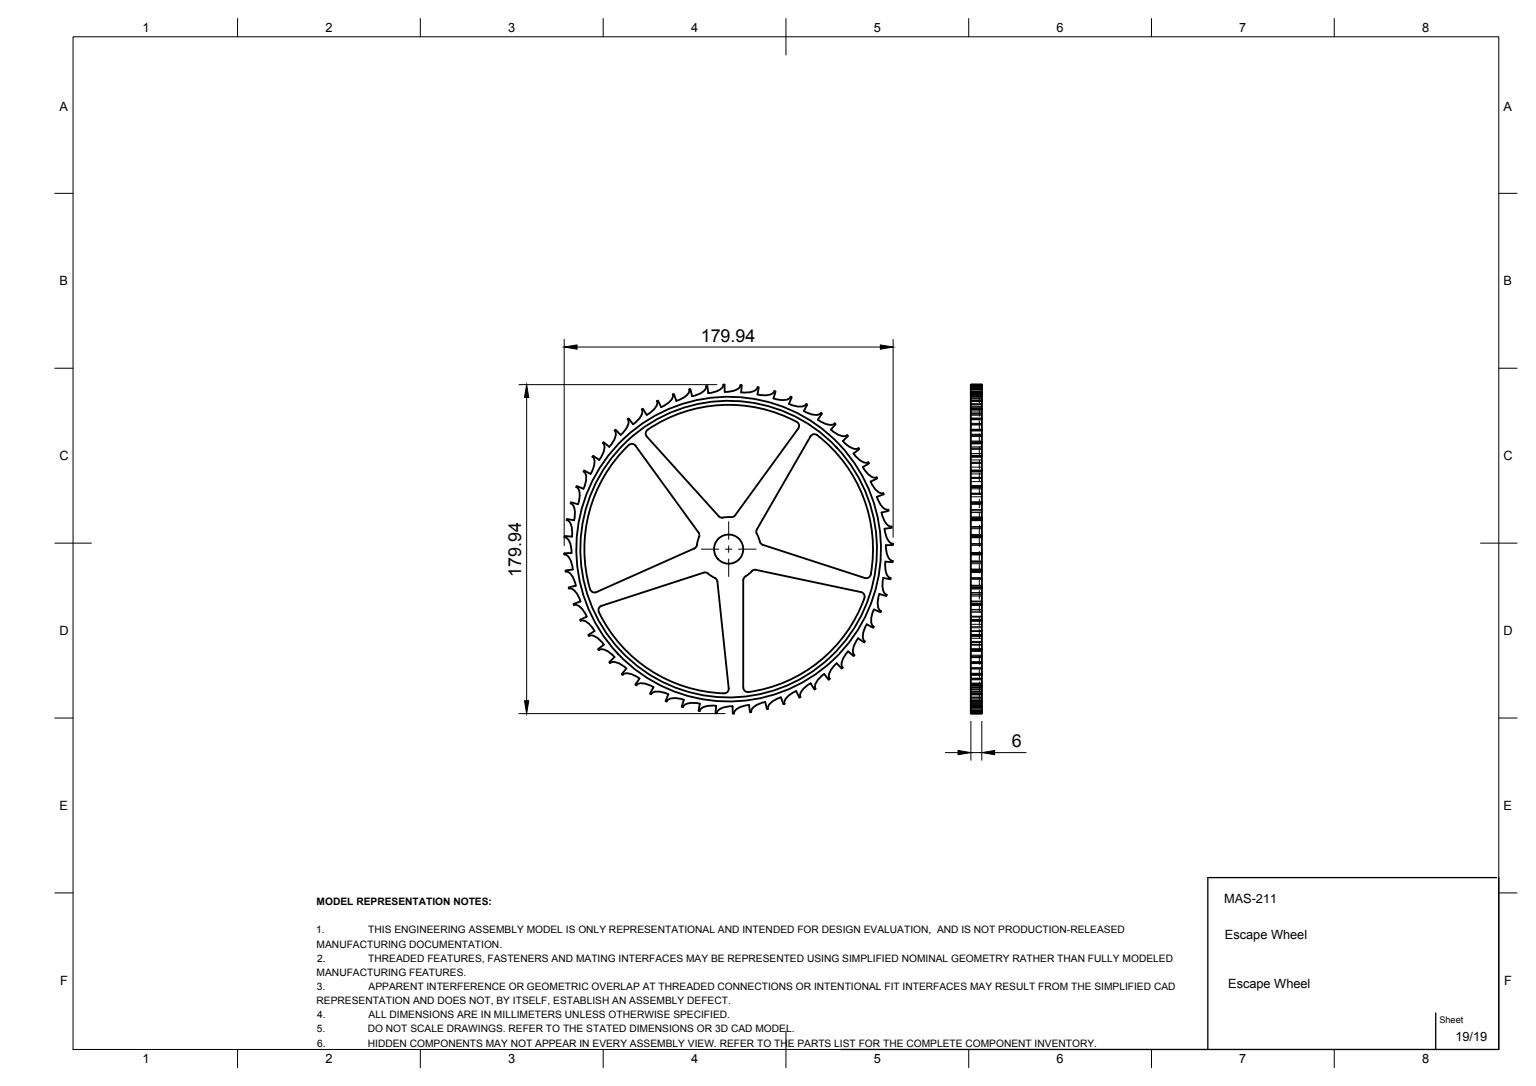
ISO-10303-21;
HEADER;
FILE_DESCRIPTION(
 (''),
 '2;1');
FILE_NAME ( 'Escape Wheel.step', '2026-10-05T20:07:59+06:00', ( '' ), ( '' ), 'STEP AP214', 'Unspecified', '' );
FILE_SCHEMA (('AUTOMOTIVE_DESIGN { 1 0 10303 214 3 1 1 }'));
ENDSEC;
DATA;
#10=MECHANICAL_DESIGN_GEOMETRIC_PRESENTATION_REPRESENTATION('',(#337),#196741);
#71=(
BOUNDED_SURFACE()
B_SPLINE_SURFACE(2,1,((#194862,#194863),(#194864,#194865),(#194866,#194867),
(#194868,#194869),(#194870,#194871)),.UNSPECIFIED.,.F.,.F.,.F.)
B_SPLINE_SURFACE_WITH_KNOTS((3,2,3),(2,2),(-88.8644935634662,-88.8637621488937,
-87.3177026764144),(0.,0.72),.UNSPECIFIED.)
GEOMETRIC_REPRESENTATION_ITEM()
RATIONAL_B_SPLINE_SURFACE(((1.,1.),(1.00013629089276,1.00013629089276),
(1.0002727088269,1.0002727088269),(0.711913347097769,0.711913347097769),
(0.991190559346467,0.991190559346467)))
REPRESENTATION_ITEM('')
SURFACE()
) ;
#72=(
BOUNDED_SURFACE()
B_SPLINE_SURFACE(2,1,((#194889,#194890),(#194891,#194892),(#194893,#194894),
(#194895,#194896),(#194897,#194898)),.UNSPECIFIED.,.F.,.F.,.F.)
B_SPLINE_SURFACE_WITH_KNOTS((3,2,3),(2,2),(-82.6275148008652,-82.6267833862927,
-81.0807239138134),(0.,0.720000000000001),.UNSPECIFIED.)
GEOMETRIC_REPRESENTATION_ITEM()
RATIONAL_B_SPLINE_SURFACE(((0.991190559346467,0.991190559346467),(0.991325649592695,
0.991325649592695),(0.991460865761138,0.991460865761138),(0.705641788716053,
0.705641788716053),(0.982458724937563,0.982458724937563)))
REPRESENTATION_ITEM('')
SURFACE()
) ;
#73=(
BOUNDED_SURFACE()
B_SPLINE_SURFACE(2,1,((#194916,#194917),(#194918,#194919),(#194920,#194921),
(#194922,#194923),(#194924,#194925)),.UNSPECIFIED.,.F.,.F.,.F.)
B_SPLINE_SURFACE_WITH_KNOTS((3,2,3),(2,2),(-76.3905360382642,-76.3898046236916,
-74.8437451512123),(0.,0.720000000000001),.UNSPECIFIED.)
GEOMETRIC_REPRESENTATION_ITEM()
RATIONAL_B_SPLINE_SURFACE(((0.982458724937563,0.982458724937563),(0.982592625114284,
0.982592625114284),(0.982726650103915,0.982726650103915),(0.699425479255707,
0.699425479255707),(0.97380381310568,0.97380381310568)))
REPRESENTATION_ITEM('')
SURFACE()
) ;
#74=(
BOUNDED_SURFACE()
B_SPLINE_SURFACE(2,1,((#194943,#194944),(#194945,#194946),(#194947,#194948),
(#194949,#194950),(#194951,#194952)),.UNSPECIFIED.,.F.,.F.,.F.)
B_SPLINE_SURFACE_WITH_KNOTS((3,2,3),(2,2),(-70.1535572756631,-70.1528258610906,
-68.6067663886113),(0.,0.720000000000001),.UNSPECIFIED.)
GEOMETRIC_REPRESENTATION_ITEM()
RATIONAL_B_SPLINE_SURFACE(((0.97380381310568,0.97380381310568),(0.97393653369674,
0.97393653369674),(0.974069378001179,0.974069378001179),(0.693263932004635,
0.693263932004635),(0.965225146205942,0.965225146205942)))
REPRESENTATION_ITEM('')
SURFACE()
) ;
#75=(
BOUNDED_SURFACE()
B_SPLINE_SURFACE(2,1,((#194970,#194971),(#194972,#194973),(#194974,#194975),
(#194976,#194977),(#194978,#194979)),.UNSPECIFIED.,.F.,.F.,.F.)
B_SPLINE_SURFACE_WITH_KNOTS((3,2,3),(2,2),(-63.9165785130621,-63.9158470984896,
-62.3697876260103),(0.,0.72),.UNSPECIFIED.)
GEOMETRIC_REPRESENTATION_ITEM()
RATIONAL_B_SPLINE_SURFACE(((0.965225146205942,0.965225146205942),(0.965356697602832,
0.965356697602832),(0.965488371623255,0.965488371623255),(0.687156664538405,
0.687156664538405),(0.956722052563143,0.956722052563143)))
REPRESENTATION_ITEM('')
SURFACE()
) ;
#76=(
BOUNDED_SURFACE()
B_SPLINE_SURFACE(2,1,((#194997,#194998),(#194999,#195000),(#195001,#195002),
(#195003,#195004),(#195005,#195006)),.UNSPECIFIED.,.F.,.F.,.F.)
B_SPLINE_SURFACE_WITH_KNOTS((3,2,3),(2,2),(-57.6795997504611,-57.6788683358886,
-56.1328088634093),(0.,0.720000000000001),.UNSPECIFIED.)
GEOMETRIC_REPRESENTATION_ITEM()
RATIONAL_B_SPLINE_SURFACE(((0.956722052563143,0.956722052563143),(0.956852445065809,
0.956852445065809),(0.956982959111764,0.956982959111764),(0.681103198682475,
0.681103198682475),(0.948293866419162,0.948293866419162)))
REPRESENTATION_ITEM('')
SURFACE()
) ;
#77=(
BOUNDED_SURFACE()
B_SPLINE_SURFACE(2,1,((#195024,#195025),(#195026,#195027),(#195028,#195029),
(#195030,#195031),(#195032,#195033)),.UNSPECIFIED.,.F.,.F.,.F.)
B_SPLINE_SURFACE_WITH_KNOTS((3,2,3),(2,2),(-51.4426209878601,-51.4418895732875,
-49.8958301008082),(0.,0.720000000000001),.UNSPECIFIED.)
GEOMETRIC_REPRESENTATION_ITEM()
RATIONAL_B_SPLINE_SURFACE(((0.948293866419162,0.948293866419162),(0.948423110236814,
0.948423110236814),(0.948552474527026,0.948552474527026),(0.67510306047475,
0.67510306047475),(0.939939927880833,0.939939927880833)))
REPRESENTATION_ITEM('')
SURFACE()
) ;
#78=(
BOUNDED_SURFACE()
B_SPLINE_SURFACE(2,1,((#195051,#195052),(#195053,#195054),(#195055,#195056),
(#195057,#195058),(#195059,#195060)),.UNSPECIFIED.,.F.,.F.,.F.)
B_SPLINE_SURFACE_WITH_KNOTS((3,2,3),(2,2),(-45.205642225259,-45.2049108106865,
-43.6588513382072),(0.,0.72),.UNSPECIFIED.)
GEOMETRIC_REPRESENTATION_ITEM()
RATIONAL_B_SPLINE_SURFACE(((0.939939927880833,0.939939927880833),(0.940068033132744,
0.940068033132744),(0.940196257795919,0.940196257795919),(0.66915578012848,
0.66915578012848),(0.931659582868281,0.931659582868281)))
REPRESENTATION_ITEM('')
SURFACE()
) ;
#79=(
BOUNDED_SURFACE()
B_SPLINE_SURFACE(2,1,((#195078,#195079),(#195080,#195081),(#195082,#195083),
(#195084,#195085),(#195086,#195087)),.UNSPECIFIED.,.F.,.F.,.F.)
B_SPLINE_SURFACE_WITH_KNOTS((3,2,3),(2,2),(-38.968663462658,-38.9679320480855,
-37.4218725756062),(0.,0.720000000000001),.UNSPECIFIED.)
GEOMETRIC_REPRESENTATION_ITEM()
RATIONAL_B_SPLINE_SURFACE(((0.931659582868281,0.931659582868281),(0.931786559584578,
0.931786559584578),(0.931913654660192,0.931913654660192),(0.663260891995469,
0.663260891995469),(0.923452183063708,0.923452183063708)))
REPRESENTATION_ITEM('')
SURFACE()
) ;
#80=(
BOUNDED_SURFACE()
B_SPLINE_SURFACE(2,1,((#195105,#195106),(#195107,#195108),(#195109,#195110),
(#195111,#195112),(#195113,#195114)),.UNSPECIFIED.,.F.,.F.,.F.)
B_SPLINE_SURFACE_WITH_KNOTS((3,2,3),(2,2),(-32.731684700057,-32.7309532854845,
-31.1848938130052),(0.,0.720000000000001),.UNSPECIFIED.)
GEOMETRIC_REPRESENTATION_ITEM()
RATIONAL_B_SPLINE_SURFACE(((0.923452183063708,0.923452183063708),(0.923578041186158,
0.923578041186158),(0.923704016625246,0.923704016625246),(0.657417934529626,
0.657417934529626),(0.915317085860633,0.915317085860633)))
REPRESENTATION_ITEM('')
SURFACE()
) ;
#81=(
BOUNDED_SURFACE()
B_SPLINE_SURFACE(2,1,((#195132,#195133),(#195134,#195135),(#195136,#195137),
(#195138,#195139),(#195140,#195141)),.UNSPECIFIED.,.F.,.F.,.F.)
B_SPLINE_SURFACE_WITH_KNOTS((3,2,3),(2,2),(-26.4947059374559,-26.4939745228834,
-24.9479150504041),(0.,0.720000000000004),.UNSPECIFIED.)
GEOMETRIC_REPRESENTATION_ITEM()
RATIONAL_B_SPLINE_SURFACE(((0.915317085860633,0.915317085860633),(0.915441835243423,
0.915441835243423),(0.915566700909357,0.915566700909357),(0.651626450250819,
0.651626450250819),(0.907253654313579,0.907253654313579)))
REPRESENTATION_ITEM('')
SURFACE()
) ;
#82=(
BOUNDED_SURFACE()
B_SPLINE_SURFACE(2,1,((#195159,#195160),(#195161,#195162),(#195163,#195164),
(#195165,#195166),(#195167,#195168)),.UNSPECIFIED.,.F.,.F.,.F.)
B_SPLINE_SURFACE_WITH_KNOTS((3,2,3),(2,2),(-20.2577271748549,-20.2569957602824,
-18.7109362878031),(0.,0.720000000000001),.UNSPECIFIED.)
GEOMETRIC_REPRESENTATION_ITEM()
RATIONAL_B_SPLINE_SURFACE(((0.907253654313579,0.907253654313579),(0.907377304724085,
0.907377304724085),(0.907501070393345,0.907501070393345),(0.645885985709063,
0.645885985709063),(0.899261257088203,0.899261257088203)))
REPRESENTATION_ITEM('')
SURFACE()
) ;
#83=(
BOUNDED_SURFACE()
B_SPLINE_SURFACE(2,1,((#195186,#195187),(#195188,#195189),(#195190,#195191),
(#195192,#195193),(#195194,#195195)),.UNSPECIFIED.,.F.,.F.,.F.)
B_SPLINE_SURFACE_WITH_KNOTS((3,2,3),(2,2),(-14.0207484122539,-14.0200169976814,
-12.4739575252021),(0.,0.72),.UNSPECIFIED.)
GEOMETRIC_REPRESENTATION_ITEM()
RATIONAL_B_SPLINE_SURFACE(((0.899261257088203,0.899261257088203),(0.899383818207756,
0.899383818207756),(0.899506493570697,0.899506493570697),(0.64019609144901,
0.64019609144901),(0.891339268411863,0.891339268411863)))
REPRESENTATION_ITEM('')
SURFACE()
) ;
#84=(
BOUNDED_SURFACE()
B_SPLINE_SURFACE(2,1,((#195213,#195214),(#195215,#195216),(#195217,#195218),
(#195219,#195220),(#195221,#195222)),.UNSPECIFIED.,.F.,.F.,.F.)
B_SPLINE_SURFACE_WITH_KNOTS((3,2,3),(2,2),(-7.78376964965284,-7.78303823508033,
-6.23697876260103),(0.,0.72),.UNSPECIFIED.)
GEOMETRIC_REPRESENTATION_ITEM()
RATIONAL_B_SPLINE_SURFACE(((0.891339268411863,0.891339268411863),(0.891460749836507,
0.891460749836507),(0.891582344498119,0.891582344498119),(0.634556321974766,
0.634556321974766),(0.883487068024626,0.883487068024626)))
REPRESENTATION_ITEM('')
SURFACE()
) ;
#85=(
BOUNDED_SURFACE()
B_SPLINE_SURFACE(2,1,((#195240,#195241),(#195242,#195243),(#195244,#195245),
(#195246,#195247),(#195248,#195249)),.UNSPECIFIED.,.F.,.F.,.F.)
B_SPLINE_SURFACE_WITH_KNOTS((3,2,3),(2,2),(-1.54679088705182,-1.54605947247931,
0.),(0.,0.72),.UNSPECIFIED.)
GEOMETRIC_REPRESENTATION_ITEM()
RATIONAL_B_SPLINE_SURFACE(((0.883487068024626,0.883487068024626),(0.883607479265868,
0.883607479265868),(0.883728002746525,0.883728002746525),(0.628966235715006,
0.628966235715006),(0.875704041130699,0.875704041130699)))
REPRESENTATION_ITEM('')
SURFACE()
) ;
#86=(
BOUNDED_SURFACE()
B_SPLINE_SURFACE(2,1,((#195267,#195268),(#195269,#195270),(#195271,#195272),
(#195273,#195274),(#195275,#195276)),.UNSPECIFIED.,.F.,.F.,.F.)
B_SPLINE_SURFACE_WITH_KNOTS((3,2,3),(2,2),(4.69018787554921,4.69091929012172,
6.23697876260103),(0.,0.72),.UNSPECIFIED.)
GEOMETRIC_REPRESENTATION_ITEM()
RATIONAL_B_SPLINE_SURFACE(((0.875704041130699,0.875704041130699),(0.875823391616258,
0.875823391616258),(0.875942853352465,0.875942853352465),(0.623425394988399,
0.623425394988399),(0.8679895783503,0.8679895783503)))
REPRESENTATION_ITEM('')
SURFACE()
) ;
#87=(
BOUNDED_SURFACE()
B_SPLINE_SURFACE(2,1,((#195294,#195295),(#195296,#195297),(#195298,#195299),
(#195300,#195301),(#195302,#195303)),.UNSPECIFIED.,.F.,.F.,.F.)
B_SPLINE_SURFACE_WITH_KNOTS((3,2,3),(2,2),(10.9271666381502,10.9278980527228,
12.4739575252021),(0.,0.72),.UNSPECIFIED.)
GEOMETRIC_REPRESENTATION_ITEM()
RATIONAL_B_SPLINE_SURFACE(((0.8679895783503,0.8679895783503),(0.868107877424839,
0.868107877424839),(0.86822628676997,0.86822628676997),(0.617933365969343,
0.617933365969343),(0.860343075671938,0.860343075671938)))
REPRESENTATION_ITEM('')
SURFACE()
) ;
#88=(
BOUNDED_SURFACE()
B_SPLINE_SURFACE(2,1,((#195321,#195322),(#195323,#195324),(#195325,#195326),
(#195327,#195328),(#195329,#195330)),.UNSPECIFIED.,.F.,.F.,.F.)
B_SPLINE_SURFACE_WITH_KNOTS((3,2,3),(2,2),(17.1641454007513,17.1648768153238,
18.7109362878031),(0.,0.72),.UNSPECIFIED.)
GEOMETRIC_REPRESENTATION_ITEM()
RATIONAL_B_SPLINE_SURFACE(((0.860343075671938,0.860343075671938),(0.8604603325978,
0.8604603325978),(0.860577698822833,0.860577698822833),(0.612489718653998,
0.612489718653998),(0.852763934405128,0.852763934405128)))
REPRESENTATION_ITEM('')
SURFACE()
) ;
#89=(
BOUNDED_SURFACE()
B_SPLINE_SURFACE(2,1,((#195348,#195349),(#195350,#195351),(#195352,#195353),
(#195354,#195355),(#195356,#195357)),.UNSPECIFIED.,.F.,.F.,.F.)
B_SPLINE_SURFACE_WITH_KNOTS((3,2,3),(2,2),(23.4011241633523,23.4018555779248,
24.9479150504041),(0.,0.72),.UNSPECIFIED.)
GEOMETRIC_REPRESENTATION_ITEM()
RATIONAL_B_SPLINE_SURFACE(((0.852763934405128,0.852763934405128),(0.852880158363061,
0.852880158363061),(0.8529964906573,0.8529964906573),(0.607094026826617,
0.607094026826617),(0.845251561133513,0.845251561133513)))
REPRESENTATION_ITEM('')
SURFACE()
) ;
#90=(
BOUNDED_SURFACE()
B_SPLINE_SURFACE(2,1,((#195375,#195376),(#195377,#195378),(#195379,#195380),
(#195381,#195382),(#195383,#195384)),.UNSPECIFIED.,.F.,.F.,.F.)
B_SPLINE_SURFACE_WITH_KNOTS((3,2,3),(2,2),(29.6381029259533,29.6388343405258,
31.1848938130052),(0.,0.72),.UNSPECIFIED.)
GEOMETRIC_REPRESENTATION_ITEM()
RATIONAL_B_SPLINE_SURFACE(((0.845251561133513,0.845251561133513),(0.845366761223386,
0.845366761223386),(0.845482068695182,0.845482068695182),(0.601745868026174,
0.601745868026174),(0.837805367668402,0.837805367668402)))
REPRESENTATION_ITEM('')
SURFACE()
) ;
#91=(
BOUNDED_SURFACE()
B_SPLINE_SURFACE(2,1,((#195402,#195403),(#195404,#195405),(#195406,#195407),
(#195408,#195409),(#195410,#195411)),.UNSPECIFIED.,.F.,.F.,.F.)
B_SPLINE_SURFACE_WITH_KNOTS((3,2,3),(2,2),(35.8750816885544,35.8758131031269,
37.4218725756062),(0.,0.72),.UNSPECIFIED.)
GEOMETRIC_REPRESENTATION_ITEM()
RATIONAL_B_SPLINE_SURFACE(((0.837805367668402,0.837805367668402),(0.83791955290992,
0.83791955290992),(0.838033844587386,0.838033844587386),(0.596444823513289,
0.596444823513289),(0.830424771002716,0.830424771002716)))
REPRESENTATION_ITEM('')
SURFACE()
) ;
#92=(
BOUNDED_SURFACE()
B_SPLINE_SURFACE(2,1,((#195429,#195430),(#195431,#195432),(#195433,#195434),
(#195435,#195436),(#195437,#195438)),.UNSPECIFIED.,.F.,.F.,.F.)
B_SPLINE_SURFACE_WITH_KNOTS((3,2,3),(2,2),(42.1120604511554,42.1127918657279,
43.6588513382072),(0.,0.72),.UNSPECIFIED.)
GEOMETRIC_REPRESENTATION_ITEM()
RATIONAL_B_SPLINE_SURFACE(((0.830424771002716,0.830424771002716),(0.830537950336125,
0.830537950336125),(0.830651235167842,0.830651235167842),(0.591190478237442,
0.591190478237442),(0.823109193265344,0.823109193265344)))
REPRESENTATION_ITEM('')
SURFACE()
) ;
#93=(
BOUNDED_SURFACE()
B_SPLINE_SURFACE(2,1,((#195456,#195457),(#195458,#195459),(#195460,#195461),
(#195462,#195463),(#195464,#195465)),.UNSPECIFIED.,.F.,.F.,.F.)
B_SPLINE_SURFACE_WITH_KNOTS((3,2,3),(2,2),(48.3490392137564,48.3497706283289,
49.8958301008082),(0.,0.72),.UNSPECIFIED.)
GEOMETRIC_REPRESENTATION_ITEM()
RATIONAL_B_SPLINE_SURFACE(((0.823109193265344,0.823109193265344),(0.823221375552132,
0.823221375552132),(0.823333662407847,0.823333662407847),(0.585982420804475,
0.585982420804475),(0.815858061675895,0.815858061675895)))
REPRESENTATION_ITEM('')
SURFACE()
) ;
#94=(
BOUNDED_SURFACE()
B_SPLINE_SURFACE(2,1,((#195483,#195484),(#195485,#195486),(#195487,#195488),
(#195489,#195490),(#195491,#195492)),.UNSPECIFIED.,.F.,.F.,.F.)
B_SPLINE_SURFACE_WITH_KNOTS((3,2,3),(2,2),(54.5860179763575,54.58674939093,
56.1328088634093),(0.,0.720000000000001),.UNSPECIFIED.)
GEOMETRIC_REPRESENTATION_ITEM()
RATIONAL_B_SPLINE_SURFACE(((0.815858061675895,0.815858061675895),(0.815969255699486,
0.815969255699486),(0.816080553370809,0.816080553370809),(0.580820243444385,
0.580820243444385),(0.808670808499855,0.808670808499855)))
REPRESENTATION_ITEM('')
SURFACE()
) ;
#95=(
BOUNDED_SURFACE()
B_SPLINE_SURFACE(2,1,((#195510,#195511),(#195512,#195513),(#195514,#195515),
(#195516,#195517),(#195518,#195519)),.UNSPECIFIED.,.F.,.F.,.F.)
B_SPLINE_SURFACE_WITH_KNOTS((3,2,3),(2,2),(60.8229967389585,60.823728153531,
62.3697876260103),(0.,0.720000000000001),.UNSPECIFIED.)
GEOMETRIC_REPRESENTATION_ITEM()
RATIONAL_B_SPLINE_SURFACE(((0.808670808499855,0.808670808499855),(0.808781022966294,
0.808781022966294),(0.808891340167387,0.808891340167387),(0.575703541979391,
0.575703541979391),(0.801546871004132,0.801546871004132)))
REPRESENTATION_ITEM('')
SURFACE()
) ;
#96=(
BOUNDED_SURFACE()
B_SPLINE_SURFACE(2,1,((#195537,#195538),(#195539,#195540),(#195541,#195542),
(#195543,#195544),(#195545,#195546)),.UNSPECIFIED.,.F.,.F.,.F.)
B_SPLINE_SURFACE_WITH_KNOTS((3,2,3),(2,2),(67.0599755015595,67.060706916132,
68.6067663886113),(0.,0.72),.UNSPECIFIED.)
GEOMETRIC_REPRESENTATION_ITEM()
RATIONAL_B_SPLINE_SURFACE(((0.801546871004132,0.801546871004132),(0.801656114542769,
0.801656114542769),(0.801765459911026,0.801765459911026),(0.570631915792295,
0.570631915792295),(0.794485691412996,0.794485691412996)))
REPRESENTATION_ITEM('')
SURFACE()
) ;
#97=(
BOUNDED_SURFACE()
B_SPLINE_SURFACE(2,1,((#195564,#195565),(#195566,#195567),(#195568,#195569),
(#195570,#195571),(#195572,#195573)),.UNSPECIFIED.,.F.,.F.,.F.)
B_SPLINE_SURFACE_WITH_KNOTS((3,2,3),(2,2),(73.2969542641605,73.2976856787331,
74.8437451512124),(0.,0.720000000000001),.UNSPECIFIED.)
GEOMETRIC_REPRESENTATION_ITEM()
RATIONAL_B_SPLINE_SURFACE(((0.794485691412996,0.794485691412996),(0.794593972577163,
0.794593972577163),(0.794702354673887,0.794702354673887),(0.565604967795111,
0.565604967795111),(0.787486716864412,0.787486716864412)))
REPRESENTATION_ITEM('')
SURFACE()
) ;
#98=(
BOUNDED_SURFACE()
B_SPLINE_SURFACE(2,1,((#195591,#195592),(#195593,#195594),(#195595,#195596),
(#195597,#195598),(#195599,#195600)),.UNSPECIFIED.,.F.,.F.,.F.)
B_SPLINE_SURFACE_WITH_KNOTS((3,2,3),(2,2),(79.5339330267616,79.5346644413341,
81.0807239138134),(0.,0.72),.UNSPECIFIED.)
GEOMETRIC_REPRESENTATION_ITEM()
RATIONAL_B_SPLINE_SURFACE(((0.787486716864412,0.787486716864412),(0.78759404413209,
0.78759404413209),(0.787701471443165,0.787701471443165),(0.560622304397977,
0.560622304397977),(0.78054939936675,0.78054939936675)))
REPRESENTATION_ITEM('')
SURFACE()
) ;
#99=(
BOUNDED_SURFACE()
B_SPLINE_SURFACE(2,1,((#195618,#195619),(#195620,#195621),(#195622,#195623),
(#195624,#195625),(#195626,#195627)),.UNSPECIFIED.,.F.,.F.,.F.)
B_SPLINE_SURFACE_WITH_KNOTS((3,2,3),(2,2),(85.7709117893626,85.7716432039351,
87.3177026764144),(0.,0.72),.UNSPECIFIED.)
GEOMETRIC_REPRESENTATION_ITEM()
RATIONAL_B_SPLINE_SURFACE(((0.78054939936675,0.78054939936675),(0.780655781141232,
0.780655781141232),(0.780762262077786,0.780762262077786),(0.555683535478336,
0.555683535478336),(0.773673195755878,0.773673195755878)))
REPRESENTATION_ITEM('')
SURFACE()
) ;
#100=(
BOUNDED_SURFACE()
B_SPLINE_SURFACE(2,1,((#195645,#195646),(#195647,#195648),(#195649,#195650),
(#195651,#195652),(#195653,#195654)),.UNSPECIFIED.,.F.,.F.,.F.)
B_SPLINE_SURFACE_WITH_KNOTS((3,2,3),(2,2),(92.0078905519636,92.0086219665361,
93.5546814390155),(0.,0.720000000000001),.UNSPECIFIED.)
GEOMETRIC_REPRESENTATION_ITEM()
RATIONAL_B_SPLINE_SURFACE(((0.773673195755878,0.773673195755878),(0.773778640366431,
0.773778640366431),(0.773884183265494,0.773884183265494),(0.550788274350394,
0.550788274350394),(0.766857567652637,0.766857567652637)))
REPRESENTATION_ITEM('')
SURFACE()
) ;
#101=(
BOUNDED_SURFACE()
B_SPLINE_SURFACE(2,1,((#195672,#195673),(#195674,#195675),(#195676,#195677),
(#195678,#195679),(#195680,#195681)),.UNSPECIFIED.,.F.,.F.,.F.)
B_SPLINE_SURFACE_WITH_KNOTS((3,2,3),(2,2),(98.2448693145647,98.2456007291372,
99.7916602016165),(0.,0.720000000000001),.UNSPECIFIED.)
GEOMETRIC_REPRESENTATION_ITEM()
RATIONAL_B_SPLINE_SURFACE(((0.766857567652637,0.766857567652637),(0.766962083355152,
0.766962083355152),(0.767066696480309,0.767066696480309),(0.545936137734843,
0.545936137734843),(0.760101981420689,0.760101981420689)))
REPRESENTATION_ITEM('')
SURFACE()
) ;
#102=(
BOUNDED_SURFACE()
B_SPLINE_SURFACE(2,1,((#195699,#195700),(#195701,#195702),(#195703,#195704),
(#195705,#195706),(#195707,#195708)),.UNSPECIFIED.,.F.,.F.,.F.)
B_SPLINE_SURFACE_WITH_KNOTS((3,2,3),(2,2),(104.481848077166,104.482579491738,
106.028638964218),(0.,0.720000000000001),.UNSPECIFIED.)
GEOMETRIC_REPRESENTATION_ITEM()
RATIONAL_B_SPLINE_SURFACE(((0.760101981420689,0.760101981420689),(0.760205576398325,
0.760205576398325),(0.760309267940364,0.760309267940364),(0.541126745728849,
0.541126745728849),(0.753405908124731,0.753405908124731)))
REPRESENTATION_ITEM('')
SURFACE()
) ;
#103=(
BOUNDED_SURFACE()
B_SPLINE_SURFACE(2,1,((#195726,#195727),(#195728,#195729),(#195730,#195731),
(#195732,#195733),(#195734,#195735)),.UNSPECIFIED.,.F.,.F.,.F.)
B_SPLINE_SURFACE_WITH_KNOTS((3,2,3),(2,2),(110.718826839767,110.719558254339,
112.265617726819),(0.,0.720000000000001),.UNSPECIFIED.)
GEOMETRIC_REPRESENTATION_ITEM()
RATIONAL_B_SPLINE_SURFACE(((0.753405908124731,0.753405908124731),(0.753508590488559,
0.753508590488559),(0.753611368566113,0.753611368566113),(0.536359721776312,
0.536359721776312),(0.746768823489085,0.746768823489085)))
REPRESENTATION_ITEM('')
SURFACE()
) ;
#104=(
BOUNDED_SURFACE()
B_SPLINE_SURFACE(2,1,((#195753,#195754),(#195755,#195756),(#195757,#195758),
(#195759,#195760),(#195761,#195762)),.UNSPECIFIED.,.F.,.F.,.F.)
B_SPLINE_SURFACE_WITH_KNOTS((3,2,3),(2,2),(116.955805602368,116.95653701694,
118.50259648942),(0.,0.720000000000001),.UNSPECIFIED.)
GEOMETRIC_REPRESENTATION_ITEM()
RATIONAL_B_SPLINE_SURFACE(((0.746768823489085,0.746768823489085),(0.746870601278723,
0.746870601278723),(0.746972473938902,0.746972473938902),(0.531634692638378,
0.531634692638378),(0.74019020785665,0.74019020785665)))
REPRESENTATION_ITEM('')
SURFACE()
) ;
#105=(
BOUNDED_SURFACE()
B_SPLINE_SURFACE(2,1,((#195780,#195781),(#195782,#195783),(#195784,#195785),
(#195786,#195787),(#195788,#195789)),.UNSPECIFIED.,.F.,.F.,.F.)
B_SPLINE_SURFACE_WITH_KNOTS((3,2,3),(2,2),(123.192784364969,123.193515779541,
124.739575252021),(0.,0.720000000000001),.UNSPECIFIED.)
GEOMETRIC_REPRESENTATION_ITEM()
RATIONAL_B_SPLINE_SURFACE(((0.74019020785665,0.74019020785665),(0.74029108904089,
0.74029108904089),(0.740392064259915,0.740392064259915),(0.526951288364221,
0.526951288364221),(0.73366954614821,0.73366954614821)))
REPRESENTATION_ITEM('')
SURFACE()
) ;
#106=(
BOUNDED_SURFACE()
B_SPLINE_SURFACE(2,1,((#195807,#195808),(#195809,#195810),(#195811,#195812),
(#195813,#195814),(#195815,#195816)),.UNSPECIFIED.,.F.,.F.,.F.)
B_SPLINE_SURFACE_WITH_KNOTS((3,2,3),(2,2),(129.42976312757,129.430494542142,
130.976554014622),(0.,0.720000000000003),.UNSPECIFIED.)
GEOMETRIC_REPRESENTATION_ITEM()
RATIONAL_B_SPLINE_SURFACE(((0.73366954614821,0.73366954614821),(0.733769538625645,
0.733769538625645),(0.73386962430947,0.73386962430947),(0.522309142262074,
0.522309142262074),(0.727206327822113,0.727206327822113)))
REPRESENTATION_ITEM('')
SURFACE()
) ;
#107=(
BOUNDED_SURFACE()
B_SPLINE_SURFACE(2,1,((#195834,#195835),(#195836,#195837),(#195838,#195839),
(#195840,#195841),(#195842,#195843)),.UNSPECIFIED.,.F.,.F.,.F.)
B_SPLINE_SURFACE_WITH_KNOTS((3,2,3),(2,2),(135.666741890171,135.667473304743,
137.213532777223),(0.,0.72),.UNSPECIFIED.)
GEOMETRIC_REPRESENTATION_ITEM()
RATIONAL_B_SPLINE_SURFACE(((0.727206327822113,0.727206327822113),(0.727305439421753,
0.727305439421753),(0.727404643406686,0.727404643406686),(0.517707890870518,
0.517707890870518),(0.720800046834291,0.720800046834291)))
REPRESENTATION_ITEM('')
SURFACE()
) ;
#108=(
BOUNDED_SURFACE()
B_SPLINE_SURFACE(2,1,((#195861,#195862),(#195863,#195864),(#195865,#195866),
(#195867,#195868),(#195869,#195870)),.UNSPECIFIED.,.F.,.F.,.F.)
B_SPLINE_SURFACE_WITH_KNOTS((3,2,3),(2,2),(141.903720652772,141.904452067344,
143.450511539824),(0.,0.72),.UNSPECIFIED.)
GEOMETRIC_REPRESENTATION_ITEM()
RATIONAL_B_SPLINE_SURFACE(((0.720800046834291,0.720800046834291),(0.720898285316175,
0.720898285316175),(0.72099661536949,0.72099661536949),(0.513147173930029,
0.513147173930029),(0.714450201598641,0.714450201598641)))
REPRESENTATION_ITEM('')
SURFACE()
) ;
#109=(
BOUNDED_SURFACE()
B_SPLINE_SURFACE(2,1,((#195888,#195889),(#195890,#195891),(#195892,#195893),
(#195894,#195895),(#195896,#195897)),.UNSPECIFIED.,.F.,.F.,.F.)
B_SPLINE_SURFACE_WITH_KNOTS((3,2,3),(2,2),(148.140699415373,148.141430829945,
149.687490302425),(0.,0.72),.UNSPECIFIED.)
GEOMETRIC_REPRESENTATION_ITEM()
RATIONAL_B_SPLINE_SURFACE(((0.714450201598641,0.714450201598641),(0.714547574654449,
0.714547574654449),(0.714645038474995,0.714645038474995),(0.508626634354764,
0.508626634354764),(0.708156294947753,0.708156294947753)))
REPRESENTATION_ITEM('')
SURFACE()
) ;
#110=(
BOUNDED_SURFACE()
B_SPLINE_SURFACE(2,1,((#195915,#195916),(#195917,#195918),(#195919,#195920),
(#195921,#195922),(#195923,#195924)),.UNSPECIFIED.,.F.,.F.,.F.)
B_SPLINE_SURFACE_WITH_KNOTS((3,2,3),(2,2),(154.377678177974,154.378409592546,
155.924469065026),(0.,0.72),.UNSPECIFIED.)
GEOMETRIC_REPRESENTATION_ITEM()
RATIONAL_B_SPLINE_SURFACE(((0.708156294947753,0.708156294947753),(0.708252810201405,
0.708252810201405),(0.708349415420208,0.708349415420208),(0.50414591820461,
0.50414591820461),(0.701917834093985,0.701917834093985)))
REPRESENTATION_ITEM('')
SURFACE()
) ;
#111=(
BOUNDED_SURFACE()
B_SPLINE_SURFACE(2,1,((#195942,#195943),(#195944,#195945),(#195946,#195947),
(#195948,#195949),(#195950,#195951)),.UNSPECIFIED.,.F.,.F.,.F.)
B_SPLINE_SURFACE_WITH_KNOTS((3,2,3),(2,2),(160.614656940575,160.615388355147,
162.161447827627),(0.,0.72),.UNSPECIFIED.)
GEOMETRIC_REPRESENTATION_ITEM()
RATIONAL_B_SPLINE_SURFACE(((0.701917834093985,0.701917834093985),(0.702013499102238,
0.702013499102238),(0.702109253283099,0.702109253283099),(0.499704674657466,
0.499704674657466),(0.695734330590878,0.695734330590878)))
REPRESENTATION_ITEM('')
SURFACE()
) ;
#112=(
BOUNDED_SURFACE()
B_SPLINE_SURFACE(2,1,((#195969,#195970),(#195971,#195972),(#195973,#195974),
(#195975,#195976),(#195977,#195978)),.UNSPECIFIED.,.F.,.F.,.F.)
B_SPLINE_SURFACE_WITH_KNOTS((3,2,3),(2,2),(166.851635703176,166.852367117749,
168.398426590228),(0.,0.720000000000001),.UNSPECIFIED.)
GEOMETRIC_REPRESENTATION_ITEM()
RATIONAL_B_SPLINE_SURFACE(((0.695734330590878,0.695734330590878),(0.695829152843917,
0.695829152843917),(0.695924063484005,0.695924063484005),(0.495302555981778,
0.495302555981778),(0.689605300294912,0.689605300294912)))
REPRESENTATION_ITEM('')
SURFACE()
) ;
#113=(
BOUNDED_SURFACE()
B_SPLINE_SURFACE(2,1,((#195996,#195997),(#195998,#195999),(#196000,#196001),
(#196002,#196003),(#196004,#196005)),.UNSPECIFIED.,.F.,.F.,.F.)
B_SPLINE_SURFACE_WITH_KNOTS((3,2,3),(2,2),(173.088614465777,173.08934588035,
174.635405352829),(0.,0.72),.UNSPECIFIED.)
GEOMETRIC_REPRESENTATION_ITEM()
RATIONAL_B_SPLINE_SURFACE(((0.689605300294912,0.689605300294912),(0.689699287216941,
0.689699287216941),(0.689793361747377,0.689793361747377),(0.490939217509313,
0.490939217509313),(0.683530263327603,0.683530263327603)))
REPRESENTATION_ITEM('')
SURFACE()
) ;
#114=(
BOUNDED_SURFACE()
B_SPLINE_SURFACE(2,1,((#196023,#196024),(#196025,#196026),(#196027,#196028),
(#196029,#196030),(#196031,#196032)),.UNSPECIFIED.,.F.,.F.,.F.)
B_SPLINE_SURFACE_WITH_KNOTS((3,2,3),(2,2),(179.325593228378,179.326324642951,
180.87238411543),(0.,0.72),.UNSPECIFIED.)
GEOMETRIC_REPRESENTATION_ITEM()
RATIONAL_B_SPLINE_SURFACE(((0.683530263327603,0.683530263327603),(0.68362342227742,
0.68362342227742),(0.683716668063863,0.683716668063863),(0.486614317608173,
0.486614317608173),(0.677508744037925,0.677508744037925)))
REPRESENTATION_ITEM('')
SURFACE()
) ;
#115=(
BOUNDED_SURFACE()
B_SPLINE_SURFACE(2,1,((#196050,#196051),(#196052,#196053),(#196054,#196055),
(#196056,#196057),(#196058,#196059)),.UNSPECIFIED.,.F.,.F.,.F.)
B_SPLINE_SURFACE_WITH_KNOTS((3,2,3),(2,2),(185.562571990979,185.563303405552,
187.109362878031),(0.,0.72),.UNSPECIFIED.)
GEOMETRIC_REPRESENTATION_ITEM()
RATIONAL_B_SPLINE_SURFACE(((0.677508744037925,0.677508744037925),(0.677601082309502,
0.677601082309502),(0.677693506652723,0.677693506652723),(0.482327517656045,
0.482327517656045),(0.671540270965073,0.671540270965073)))
REPRESENTATION_ITEM('')
SURFACE()
) ;
#116=(
BOUNDED_SURFACE()
B_SPLINE_SURFACE(2,1,((#196077,#196078),(#196079,#196080),(#196081,#196082),
(#196083,#196084),(#196085,#196086)),.UNSPECIFIED.,.F.,.F.,.F.)
B_SPLINE_SURFACE_WITH_KNOTS((3,2,3),(2,2),(191.79955075358,191.800282168153,
193.346341640632),(0.,0.72),.UNSPECIFIED.)
GEOMETRIC_REPRESENTATION_ITEM()
RATIONAL_B_SPLINE_SURFACE(((0.671540270965073,0.671540270965073),(0.671631795788127,
0.671631795788127),(0.671723405924582,0.671723405924582),(0.478078482013688,
0.478078482013688),(0.665624376801549,0.665624376801549)))
REPRESENTATION_ITEM('')
SURFACE()
) ;
#117=(
BOUNDED_SURFACE()
B_SPLINE_SURFACE(2,1,((#196104,#196105),(#196106,#196107),(#196108,#196109),
(#196110,#196111),(#196112,#196113)),.UNSPECIFIED.,.F.,.F.,.F.)
B_SPLINE_SURFACE_WITH_KNOTS((3,2,3),(2,2),(198.036529516181,198.037260930754,
199.583320403233),(0.,0.72),.UNSPECIFIED.)
GEOMETRIC_REPRESENTATION_ITEM()
RATIONAL_B_SPLINE_SURFACE(((0.665624376801549,0.665624376801549),(0.665715095342106,
0.665715095342106),(0.6658058984445,0.6658058984445),(0.473866877998657,
0.473866877998657),(0.659760598356571,0.659760598356571)))
REPRESENTATION_ITEM('')
SURFACE()
) ;
#118=(
BOUNDED_SURFACE()
B_SPLINE_SURFACE(2,1,((#196131,#196132),(#196133,#196134),(#196135,#196136),
(#196137,#196138),(#196139,#196140)),.UNSPECIFIED.,.F.,.F.,.F.)
B_SPLINE_SURFACE_WITH_KNOTS((3,2,3),(2,2),(204.273508278782,204.274239693355,
205.820299165834),(0.,0.72),.UNSPECIFIED.)
GEOMETRIC_REPRESENTATION_ITEM()
RATIONAL_B_SPLINE_SURFACE(((0.659760598356571,0.659760598356571),(0.659850517717528,
0.659850517717528),(0.659940520895381,0.659940520895381),(0.469692375859253,
0.469692375859253),(0.65394847651981,0.65394847651981)))
REPRESENTATION_ITEM('')
SURFACE()
) ;
#119=(
BOUNDED_SURFACE()
B_SPLINE_SURFACE(2,1,((#196158,#196159),(#196160,#196161),(#196162,#196163),
(#196164,#196165),(#196166,#196167)),.UNSPECIFIED.,.F.,.F.,.F.)
B_SPLINE_SURFACE_WITH_KNOTS((3,2,3),(2,2),(210.510487041383,210.511218455956,
212.057277928435),(0.,0.72),.UNSPECIFIED.)
GEOMETRIC_REPRESENTATION_ITEM()
RATIONAL_B_SPLINE_SURFACE(((0.65394847651981,0.65394847651981),(0.654037603741493,
0.654037603741493),(0.654126814041692,0.654126814041692),(0.465554648748704,
0.465554648748704),(0.64818755622544,0.64818755622544)))
REPRESENTATION_ITEM('')
SURFACE()
) ;
#120=(
BOUNDED_SURFACE()
B_SPLINE_SURFACE(2,1,((#196185,#196186),(#196187,#196188),(#196189,#196190),
(#196191,#196192),(#196193,#196194)),.UNSPECIFIED.,.F.,.F.,.F.)
B_SPLINE_SURFACE_WITH_KNOTS((3,2,3),(2,2),(216.747465803984,216.748197218557,
218.294256691036),(0.,0.720000000000001),.UNSPECIFIED.)
GEOMETRIC_REPRESENTATION_ITEM()
RATIONAL_B_SPLINE_SURFACE(((0.64818755622544,0.64818755622544),(0.648275898286154,
0.648275898286154),(0.648364322693508,0.648364322693508),(0.461453372699577,
0.461453372699577),(0.642477386416514,0.642477386416514)))
REPRESENTATION_ITEM('')
SURFACE()
) ;
#121=(
BOUNDED_SURFACE()
B_SPLINE_SURFACE(2,1,((#196212,#196213),(#196214,#196215),(#196216,#196217),
(#196218,#196219),(#196220,#196221)),.UNSPECIFIED.,.F.,.F.,.F.)
B_SPLINE_SURFACE_WITH_KNOTS((3,2,3),(2,2),(222.984444566585,222.985175981158,
224.531235453637),(0.,0.72),.UNSPECIFIED.)
GEOMETRIC_REPRESENTATION_ITEM()
RATIONAL_B_SPLINE_SURFACE(((0.642477386416514,0.642477386416514),(0.642564950233086,
0.642564950233086),(0.642652595670871,0.642652595670871),(0.457388226598407,
0.457388226598407),(0.636817520009641,0.636817520009641)))
REPRESENTATION_ITEM('')
SURFACE()
) ;
#122=(
BOUNDED_SURFACE()
B_SPLINE_SURFACE(2,1,((#196239,#196240),(#196241,#196242),(#196243,#196244),
(#196245,#196246),(#196247,#196248)),.UNSPECIFIED.,.F.,.F.,.F.)
B_SPLINE_SURFACE_WITH_KNOTS((3,2,3),(2,2),(229.221423329186,229.222154743759,
230.768214216238),(0.,0.72),.UNSPECIFIED.)
GEOMETRIC_REPRESENTATION_ITEM()
RATIONAL_B_SPLINE_SURFACE(((0.636817520009641,0.636817520009641),(0.636904312437968,
0.636904312437968),(0.63699118576847,0.63699118576847),(0.453358892160564,
0.453358892160564),(0.631207513859986,0.631207513859986)))
REPRESENTATION_ITEM('')
SURFACE()
) ;
#123=(
BOUNDED_SURFACE()
B_SPLINE_SURFACE(2,1,((#196266,#196267),(#196268,#196269),(#196270,#196271),
(#196272,#196273),(#196274,#196275)),.UNSPECIFIED.,.F.,.F.,.F.)
B_SPLINE_SURFACE_WITH_KNOTS((3,2,3),(2,2),(235.458402091787,235.45913350636,
237.005192978839),(0.,0.72),.UNSPECIFIED.)
GEOMETRIC_REPRESENTATION_ITEM()
RATIONAL_B_SPLINE_SURFACE(((0.631207513859986,0.631207513859986),(0.631293541695566,
0.631293541695566),(0.631379649720619,0.631379649720619),(0.449365053905324,
0.449365053905324),(0.625646928726572,0.625646928726572)))
REPRESENTATION_ITEM('')
SURFACE()
) ;
#124=(
BOUNDED_SURFACE()
B_SPLINE_SURFACE(2,1,((#196293,#196294),(#196295,#196296),(#196297,#196298),
(#196299,#196300),(#196301,#196302)),.UNSPECIFIED.,.F.,.F.,.F.)
B_SPLINE_SURFACE_WITH_KNOTS((3,2,3),(2,2),(241.695380854388,241.696112268961,
243.24217174144),(0.,0.72),.UNSPECIFIED.)
GEOMETRIC_REPRESENTATION_ITEM()
RATIONAL_B_SPLINE_SURFACE(((0.625646928726572,0.625646928726572),(0.625732198705041,
0.625732198705041),(0.625817548166557,0.625817548166557),(0.445406399131173,
0.445406399131173),(0.620135329237891,0.620135329237891)))
REPRESENTATION_ITEM('')
SURFACE()
) ;
#125=(
BOUNDED_SURFACE()
B_SPLINE_SURFACE(2,1,((#196320,#196321),(#196322,#196323),(#196324,#196325),
(#196326,#196327),(#196328,#196329)),.UNSPECIFIED.,.F.,.F.,.F.)
B_SPLINE_SURFACE_WITH_KNOTS((3,2,3),(2,2),(247.932359616989,247.933091031562,
249.479150504041),(0.,0.72),.UNSPECIFIED.)
GEOMETRIC_REPRESENTATION_ITEM()
RATIONAL_B_SPLINE_SURFACE(((0.620135329237891,0.620135329237891),(0.620219848035544,
0.620219848035544),(0.620304445616044,0.620304445616044),(0.441482617891324,
0.441482617891324),(0.61467228385781,0.61467228385781)))
REPRESENTATION_ITEM('')
SURFACE()
) ;
#126=(
BOUNDED_SURFACE()
B_SPLINE_SURFACE(2,1,((#196347,#196348),(#196349,#196350),(#196351,#196352),
(#196353,#196354),(#196355,#196356)),.UNSPECIFIED.,.F.,.F.,.F.)
B_SPLINE_SURFACE_WITH_KNOTS((3,2,3),(2,2),(254.16933837959,254.170069794163,
255.716129266642),(0.,0.72),.UNSPECIFIED.)
GEOMETRIC_REPRESENTATION_ITEM()
RATIONAL_B_SPLINE_SURFACE(((0.61467228385781,0.61467228385781),(0.614756058092132,
0.614756058092132),(0.614839910415267,0.614839910415267),(0.437593402969444,
0.437593402969444),(0.609257364851794,0.609257364851794)))
REPRESENTATION_ITEM('')
SURFACE()
) ;
#127=(
BOUNDED_SURFACE()
B_SPLINE_SURFACE(2,1,((#196374,#196375),(#196376,#196377),(#196378,#196379),
(#196380,#196381),(#196382,#196383)),.UNSPECIFIED.,.F.,.F.,.F.)
B_SPLINE_SURFACE_WITH_KNOTS((3,2,3),(2,2),(260.406317142191,260.407048556764,
261.953108029243),(0.,0.720000000000001),.UNSPECIFIED.)
GEOMETRIC_REPRESENTATION_ITEM()
RATIONAL_B_SPLINE_SURFACE(((0.609257364851794,0.609257364851794),(0.609340401081969,
0.609340401081969),(0.60942351471304,0.60942351471304),(0.433738449855607,
0.433738449855607),(0.603890148253404,0.603890148253404)))
REPRESENTATION_ITEM('')
SURFACE()
) ;
#128=(
BOUNDED_SURFACE()
B_SPLINE_SURFACE(2,1,((#196401,#196402),(#196403,#196404),(#196405,#196406),
(#196407,#196408),(#196409,#196410)),.UNSPECIFIED.,.F.,.F.,.F.)
B_SPLINE_SURFACE_WITH_KNOTS((3,2,3),(2,2),(266.643295904792,266.644027319365,
268.190086791844),(0.,0.72),.UNSPECIFIED.)
GEOMETRIC_REPRESENTATION_ITEM()
RATIONAL_B_SPLINE_SURFACE(((0.603890148253404,0.603890148253404),(0.603972452980838,
0.603972452980838),(0.604054834427309,0.604054834427309),(0.429917456722449,
0.429917456722449),(0.598570213831113,0.598570213831113)))
REPRESENTATION_ITEM('')
SURFACE()
) ;
#129=(
BOUNDED_SURFACE()
B_SPLINE_SURFACE(2,1,((#196428,#196429),(#196430,#196431),(#196432,#196433),
(#196434,#196435),(#196436,#196437)),.UNSPECIFIED.,.F.,.F.,.F.)
B_SPLINE_SURFACE_WITH_KNOTS((3,2,3),(2,2),(272.880274667394,272.881006081966,
274.427065554445),(0.,0.72),.UNSPECIFIED.)
GEOMETRIC_REPRESENTATION_ITEM()
RATIONAL_B_SPLINE_SURFACE(((0.598570213831113,0.598570213831113),(0.598651793499935,
0.598651793499935),(0.598733449211942,0.598733449211942),(0.426130124401535,
0.426130124401535),(0.593297145055395,0.593297145055395)))
REPRESENTATION_ITEM('')
SURFACE()
) ;
#130=(
BOUNDED_SURFACE()
B_SPLINE_SURFACE(2,1,((#196455,#196456),(#196457,#196458),(#196459,#196460),
(#196461,#196462),(#196463,#196464)),.UNSPECIFIED.,.F.,.F.,.F.)
B_SPLINE_SURFACE_WITH_KNOTS((3,2,3),(2,2),(279.117253429995,279.117984844567,
280.664044317046),(0.,0.720000000000001),.UNSPECIFIED.)
GEOMETRIC_REPRESENTATION_ITEM()
RATIONAL_B_SPLINE_SURFACE(((0.593297145055395,0.593297145055395),(0.593378006052966,
0.593378006052966),(0.593458942423824,0.593458942423824),(0.422376156359937,
0.422376156359937),(0.588070529066119,0.588070529066119)))
REPRESENTATION_ITEM('')
SURFACE()
) ;
#191=ELLIPSE('',#9102,8.73317010092234,3.9982389407695) ;
#192=ELLIPSE('',#9103,8.73317010092295,3.99823894076973) ;
#193=ELLIPSE('',#9106,8.73317010092743,3.99823894077223) ;
#194=ELLIPSE('',#9107,8.73317010092743,3.99823894077213) ;
#195=ELLIPSE('',#9110,8.73317010092711,3.99823894077243) ;
#196=ELLIPSE('',#9111,8.73317010092743,3.9982389407726) ;
#197=ELLIPSE('',#9114,8.73317010092821,3.9982389407731) ;
#198=ELLIPSE('',#9115,8.73317010092973,3.99823894077377) ;
#199=ELLIPSE('',#9118,8.73317010092634,3.99823894077158) ;
#200=ELLIPSE('',#9119,8.73317010092438,3.99823894077077) ;
#201=ELLIPSE('',#9122,8.73317010092548,3.99823894077123) ;
#202=ELLIPSE('',#9123,8.73317010092314,3.99823894077033) ;
#203=ELLIPSE('',#9126,8.73317010092227,3.99823894076999) ;
#204=ELLIPSE('',#9127,8.73317010092042,3.99823894076914) ;
#205=ELLIPSE('',#9130,8.7331701009258,3.99823894077184) ;
#206=ELLIPSE('',#9131,8.73317010092579,3.99823894077183) ;
#207=ELLIPSE('',#9134,8.73317010092678,3.99823894077257) ;
#208=ELLIPSE('',#9135,8.73317010092553,3.99823894077202) ;
#209=ELLIPSE('',#9138,8.7331701009272,3.99823894077287) ;
#210=ELLIPSE('',#9139,8.73317010092561,3.99823894077221) ;
#211=ELLIPSE('',#9142,8.73317010092469,3.99823894077177) ;
#212=ELLIPSE('',#9143,8.7331701009245,3.99823894077166) ;
#213=ELLIPSE('',#9146,8.73317010092758,3.99823894077321) ;
#214=ELLIPSE('',#9147,8.73317010092748,3.99823894077321) ;
#215=ELLIPSE('',#9150,8.73317010092198,3.99823894076988) ;
#216=ELLIPSE('',#9151,8.73317010092244,3.99823894077009) ;
#217=ELLIPSE('',#9154,8.73317010092626,3.99823894077208) ;
#218=ELLIPSE('',#9155,8.73317010092699,3.99823894077238) ;
#219=ELLIPSE('',#9158,8.73317010092677,3.99823894077194) ;
#220=ELLIPSE('',#9159,8.73317010092738,3.99823894077216) ;
#221=ELLIPSE('',#9162,8.73317010092297,3.99823894077055) ;
#222=ELLIPSE('',#9163,8.73317010092318,3.99823894077063) ;
#223=ELLIPSE('',#9166,8.73317010092442,3.99823894077025) ;
#224=ELLIPSE('',#9167,8.73317010092408,3.9982389407701) ;
#225=ELLIPSE('',#9170,8.73317010092396,3.99823894077075) ;
#226=ELLIPSE('',#9171,8.73317010092319,3.9982389407704) ;
#227=ELLIPSE('',#9174,8.73317010092369,3.99823894077059) ;
#228=ELLIPSE('',#9175,8.73317010092371,3.9982389407706) ;
#229=ELLIPSE('',#9178,8.73317010092631,3.99823894077224) ;
#230=ELLIPSE('',#9179,8.73317010092631,3.99823894077225) ;
#231=ELLIPSE('',#9182,8.73317010092421,3.99823894077116) ;
#232=ELLIPSE('',#9183,8.7331701009243,3.99823894077121) ;
#233=ELLIPSE('',#9186,8.73317010092502,3.99823894077177) ;
#234=ELLIPSE('',#9187,8.7331701009251,3.99823894077182) ;
#235=ELLIPSE('',#9190,8.73317010092506,3.99823894077112) ;
#236=ELLIPSE('',#9191,8.73317010092501,3.99823894077111) ;
#237=ELLIPSE('',#9194,8.73317010092443,3.99823894077097) ;
#238=ELLIPSE('',#9195,8.73317010092454,3.99823894077102) ;
#239=ELLIPSE('',#9198,8.73317010092613,3.99823894077172) ;
#240=ELLIPSE('',#9199,8.73317010092622,3.99823894077175) ;
#241=ELLIPSE('',#9202,8.73317010092691,3.99823894077243) ;
#242=ELLIPSE('',#9203,8.73317010092707,3.9982389407725) ;
#243=ELLIPSE('',#9206,8.73317010092902,3.99823894077356) ;
#244=ELLIPSE('',#9207,8.73317010092857,3.99823894077338) ;
#245=ELLIPSE('',#9210,8.7331701009226,3.99823894077018) ;
#246=ELLIPSE('',#9211,8.73317010092281,3.99823894077021) ;
#247=ELLIPSE('',#9214,8.73317010092556,3.99823894077181) ;
#248=ELLIPSE('',#9215,8.73317010092559,3.99823894077178) ;
#249=ELLIPSE('',#9218,8.73317010092635,3.99823894077231) ;
#250=ELLIPSE('',#9219,8.73317010092611,3.9982389407722) ;
#251=ELLIPSE('',#9222,8.73317010092494,3.99823894077155) ;
#252=ELLIPSE('',#9223,8.73317010092546,3.9982389407718) ;
#253=ELLIPSE('',#9226,8.73317010092672,3.9982389407724) ;
#254=ELLIPSE('',#9227,8.73317010092759,3.99823894077281) ;
#255=ELLIPSE('',#9230,8.73317010092427,3.99823894077119) ;
#256=ELLIPSE('',#9231,8.73317010092464,3.99823894077128) ;
#257=ELLIPSE('',#9234,8.73317010092349,3.99823894076998) ;
#258=ELLIPSE('',#9235,8.73317010092349,3.99823894076998) ;
#259=ELLIPSE('',#9238,8.733170100929,3.99823894077289) ;
#260=ELLIPSE('',#9239,8.73317010092749,3.99823894077221) ;
#261=ELLIPSE('',#9242,8.73317010092275,3.99823894077023) ;
#262=ELLIPSE('',#9243,8.7331701009221,3.99823894077012) ;
#263=ELLIPSE('',#9246,8.7331701009272,3.99823894077234) ;
#264=ELLIPSE('',#9247,8.73317010092575,3.99823894077179) ;
#265=ELLIPSE('',#9250,8.73317010092357,3.9982389407703) ;
#266=ELLIPSE('',#9251,8.73317010092264,3.99823894076992) ;
#267=ELLIPSE('',#9254,8.73317010092163,3.99823894076961) ;
#268=ELLIPSE('',#9255,8.73317010092226,3.99823894076974) ;
#269=ELLIPSE('',#9258,8.73317010092482,3.99823894077158) ;
#270=ELLIPSE('',#9259,8.73317010092302,3.99823894077092) ;
#271=ELLIPSE('',#9262,8.733170100925,3.99823894077123) ;
#272=ELLIPSE('',#9263,8.73317010092482,3.99823894077119) ;
#273=ELLIPSE('',#9266,8.73317010092451,3.99823894077103) ;
#274=ELLIPSE('',#9267,8.73317010092509,3.99823894077124) ;
#275=ELLIPSE('',#9270,8.73317010092322,3.99823894077001) ;
#276=ELLIPSE('',#9271,8.7331701009224,3.99823894076959) ;
#277=ELLIPSE('',#9274,8.73317010092819,3.9982389407725) ;
#278=ELLIPSE('',#9275,8.73317010092786,3.99823894077243) ;
#279=ELLIPSE('',#9278,8.7331701009259,3.99823894077201) ;
#280=ELLIPSE('',#9279,8.73317010092555,3.99823894077185) ;
#281=ELLIPSE('',#9282,8.73317010092734,3.99823894077257) ;
#282=ELLIPSE('',#9283,8.73317010092781,3.99823894077276) ;
#283=ELLIPSE('',#9286,8.73317010092432,3.99823894077033) ;
#284=ELLIPSE('',#9287,8.73317010092421,3.99823894077031) ;
#285=ELLIPSE('',#9290,8.73317010092571,3.99823894077219) ;
#286=ELLIPSE('',#9291,8.73317010092551,3.99823894077214) ;
#287=ELLIPSE('',#9294,8.73317010092575,3.99823894077112) ;
#288=ELLIPSE('',#9295,8.73317010092583,3.99823894077117) ;
#289=ELLIPSE('',#9298,8.73317010092938,3.99823894077288) ;
#290=ELLIPSE('',#9299,8.73317010092941,3.99823894077288) ;
#291=ELLIPSE('',#9302,8.73317010092498,3.99823894077171) ;
#292=ELLIPSE('',#9303,8.73317010092507,3.99823894077176) ;
#293=ELLIPSE('',#9306,8.73317010092869,3.99823894077326) ;
#294=ELLIPSE('',#9307,8.73317010092866,3.99823894077325) ;
#295=ELLIPSE('',#9310,8.73317010092302,3.99823894077023) ;
#296=ELLIPSE('',#9311,8.73317010092305,3.99823894077024) ;
#297=ELLIPSE('',#9314,8.73317010092288,3.99823894077039) ;
#298=ELLIPSE('',#9315,8.73317010092291,3.99823894077042) ;
#299=ELLIPSE('',#9318,8.73317010092245,3.99823894077027) ;
#300=ELLIPSE('',#9319,8.73317010092265,3.99823894077034) ;
#301=ELLIPSE('',#9322,8.7331701009217,3.99823894076996) ;
#302=ELLIPSE('',#9323,8.73317010092196,3.99823894077008) ;
#303=ELLIPSE('',#9326,8.73317010092363,3.99823894077092) ;
#304=ELLIPSE('',#9327,8.73317010092318,3.99823894077077) ;
#305=ELLIPSE('',#9330,8.73317010092656,3.99823894077185) ;
#306=ELLIPSE('',#9331,8.73317010092601,3.99823894077162) ;
#307=ELLIPSE('',#9334,8.73317010092627,3.99823894077187) ;
#308=ELLIPSE('',#9335,8.73317010092609,3.99823894077178) ;
#309=ELLIPSE('',#9338,8.73317010092587,3.99823894077181) ;
#310=ELLIPSE('',#9339,8.73317010092569,3.99823894077163) ;
#337=STYLED_ITEM('',(#196765),#356) ;
#356=MANIFOLD_SOLID_BREP('Escape Wheel',#8733) ;
#420=PLANE('',#9101) ;
#421=PLANE('',#9104) ;
#422=PLANE('',#9105) ;
#423=PLANE('',#9108) ;
#424=PLANE('',#9109) ;
#425=PLANE('',#9112) ;
#426=PLANE('',#9113) ;
#427=PLANE('',#9116) ;
#428=PLANE('',#9117) ;
#429=PLANE('',#9120) ;
#430=PLANE('',#9121) ;
#431=PLANE('',#9124) ;
#432=PLANE('',#9125) ;
#433=PLANE('',#9128) ;
#434=PLANE('',#9129) ;
#435=PLANE('',#9132) ;
#436=PLANE('',#9133) ;
#437=PLANE('',#9136) ;
#438=PLANE('',#9137) ;
#439=PLANE('',#9140) ;
#440=PLANE('',#9141) ;
#441=PLANE('',#9144) ;
#442=PLANE('',#9145) ;
#443=PLANE('',#9148) ;
#444=PLANE('',#9149) ;
#445=PLANE('',#9152) ;
#446=PLANE('',#9153) ;
#447=PLANE('',#9156) ;
#448=PLANE('',#9157) ;
#449=PLANE('',#9160) ;
#450=PLANE('',#9161) ;
#451=PLANE('',#9164) ;
#452=PLANE('',#9165) ;
#453=PLANE('',#9168) ;
#454=PLANE('',#9169) ;
#455=PLANE('',#9172) ;
#456=PLANE('',#9173) ;
#457=PLANE('',#9176) ;
#458=PLANE('',#9177) ;
#459=PLANE('',#9180) ;
#460=PLANE('',#9181) ;
#461=PLANE('',#9184) ;
#462=PLANE('',#9185) ;
#463=PLANE('',#9188) ;
#464=PLANE('',#9189) ;
#465=PLANE('',#9192) ;
#466=PLANE('',#9193) ;
#467=PLANE('',#9196) ;
#468=PLANE('',#9197) ;
#469=PLANE('',#9200) ;
#470=PLANE('',#9201) ;
#471=PLANE('',#9204) ;
#472=PLANE('',#9205) ;
#473=PLANE('',#9208) ;
#474=PLANE('',#9209) ;
#475=PLANE('',#9212) ;
#476=PLANE('',#9213) ;
#477=PLANE('',#9216) ;
#478=PLANE('',#9217) ;
#479=PLANE('',#9220) ;
#480=PLANE('',#9221) ;
#481=PLANE('',#9224) ;
#482=PLANE('',#9225) ;
#483=PLANE('',#9228) ;
#484=PLANE('',#9229) ;
#485=PLANE('',#9232) ;
#486=PLANE('',#9233) ;
#487=PLANE('',#9236) ;
#488=PLANE('',#9237) ;
#489=PLANE('',#9240) ;
#490=PLANE('',#9241) ;
#491=PLANE('',#9244) ;
#492=PLANE('',#9245) ;
#493=PLANE('',#9248) ;
#494=PLANE('',#9249) ;
#495=PLANE('',#9252) ;
#496=PLANE('',#9253) ;
#497=PLANE('',#9256) ;
#498=PLANE('',#9257) ;
#499=PLANE('',#9260) ;
#500=PLANE('',#9261) ;
#501=PLANE('',#9264) ;
#502=PLANE('',#9265) ;
#503=PLANE('',#9268) ;
#504=PLANE('',#9269) ;
#505=PLANE('',#9272) ;
#506=PLANE('',#9273) ;
#507=PLANE('',#9276) ;
#508=PLANE('',#9277) ;
#509=PLANE('',#9280) ;
#510=PLANE('',#9281) ;
#511=PLANE('',#9284) ;
#512=PLANE('',#9285) ;
#513=PLANE('',#9288) ;
#514=PLANE('',#9289) ;
#515=PLANE('',#9292) ;
#516=PLANE('',#9293) ;
#517=PLANE('',#9296) ;
#518=PLANE('',#9297) ;
#519=PLANE('',#9300) ;
#520=PLANE('',#9301) ;
#521=PLANE('',#9304) ;
#522=PLANE('',#9305) ;
#523=PLANE('',#9308) ;
#524=PLANE('',#9309) ;
#525=PLANE('',#9312) ;
#526=PLANE('',#9313) ;
#527=PLANE('',#9316) ;
#528=PLANE('',#9317) ;
#529=PLANE('',#9320) ;
#530=PLANE('',#9321) ;
#531=PLANE('',#9324) ;
#532=PLANE('',#9325) ;
#533=PLANE('',#9328) ;
#534=PLANE('',#9329) ;
#535=PLANE('',#9332) ;
#536=PLANE('',#9333) ;
#537=PLANE('',#9336) ;
#538=PLANE('',#9337) ;
#539=PLANE('',#9340) ;
#540=PLANE('',#9341) ;
#541=PLANE('',#9373) ;
#542=PLANE('',#9379) ;
#543=PLANE('',#9386) ;
#544=PLANE('',#9395) ;
#545=PLANE('',#9402) ;
#546=PLANE('',#9409) ;
#547=PLANE('',#9416) ;
#548=PLANE('',#9423) ;
#549=PLANE('',#9430) ;
#550=PLANE('',#9437) ;
#551=PLANE('',#9444) ;
#552=PLANE('',#9452) ;
#553=PLANE('',#9453) ;
#598=FACE_BOUND('',#1803,.T.) ;
#599=FACE_BOUND('',#1804,.T.) ;
#600=FACE_BOUND('',#1805,.T.) ;
#601=FACE_BOUND('',#1806,.T.) ;
#602=FACE_BOUND('',#1807,.T.) ;
#603=FACE_BOUND('',#1808,.T.) ;
#604=FACE_BOUND('',#1810,.T.) ;
#605=FACE_BOUND('',#1855,.T.) ;
#606=FACE_BOUND('',#1857,.T.) ;
#607=FACE_BOUND('',#1858,.T.) ;
#608=FACE_BOUND('',#1859,.T.) ;
#609=FACE_BOUND('',#1860,.T.) ;
#610=FACE_BOUND('',#1861,.T.) ;
#611=FACE_BOUND('',#1862,.T.) ;
#745=CIRCLE('',#9342,2.49999999999987) ;
#746=CIRCLE('',#9343,78.9146368237007) ;
#747=CIRCLE('',#9344,2.49999999999996) ;
#748=CIRCLE('',#9345,2.49999999999929) ;
#749=CIRCLE('',#9346,17.4999999999883) ;
#750=CIRCLE('',#9347,2.49999999999988) ;
#751=CIRCLE('',#9348,8.00000000000006) ;
#752=CIRCLE('',#9349,2.50000000000011) ;
#753=CIRCLE('',#9350,78.9146368237009) ;
#754=CIRCLE('',#9351,2.50000000000036) ;
#755=CIRCLE('',#9352,2.49999999999919) ;
#756=CIRCLE('',#9353,17.4999999999808) ;
#757=CIRCLE('',#9354,2.50000000000025) ;
#758=CIRCLE('',#9355,2.49999999999974) ;
#759=CIRCLE('',#9356,78.9146368237008) ;
#760=CIRCLE('',#9357,2.49999999999989) ;
#761=CIRCLE('',#9358,2.49999999999919) ;
#762=CIRCLE('',#9359,17.4999999999877) ;
#763=CIRCLE('',#9360,2.50000000000021) ;
#764=CIRCLE('',#9361,2.49999999999996) ;
#765=CIRCLE('',#9362,78.9146368237009) ;
#766=CIRCLE('',#9363,2.49999999999969) ;
#767=CIRCLE('',#9364,2.49999999999911) ;
#768=CIRCLE('',#9365,17.4999999999922) ;
#769=CIRCLE('',#9366,2.49999999999997) ;
#770=CIRCLE('',#9367,2.49999999999985) ;
#771=CIRCLE('',#9368,78.9146368237006) ;
#772=CIRCLE('',#9369,2.50000000000015) ;
#773=CIRCLE('',#9370,2.49999999999888) ;
#774=CIRCLE('',#9371,17.4999999999909) ;
#775=CIRCLE('',#9372,2.49999999999995) ;
#776=CIRCLE('',#9374,83.314636823702) ;
#777=CIRCLE('',#9376,17.4999999999885) ;
#778=CIRCLE('',#9378,2.49999999999986) ;
#779=CIRCLE('',#9381,2.49999999999987) ;
#780=CIRCLE('',#9383,78.9146368237007) ;
#781=CIRCLE('',#9385,2.49999999999997) ;
#782=CIRCLE('',#9388,2.49999999999928) ;
#783=CIRCLE('',#9390,8.00000000000006) ;
#784=CIRCLE('',#9392,17.4999999999808) ;
#785=CIRCLE('',#9394,2.50000000000025) ;
#786=CIRCLE('',#9397,2.50000000000011) ;
#787=CIRCLE('',#9399,78.9146368237007) ;
#788=CIRCLE('',#9401,2.50000000000036) ;
#789=CIRCLE('',#9404,2.4999999999992) ;
#790=CIRCLE('',#9406,17.4999999999878) ;
#791=CIRCLE('',#9408,2.50000000000022) ;
#792=CIRCLE('',#9411,2.49999999999976) ;
#793=CIRCLE('',#9413,78.9146368237008) ;
#794=CIRCLE('',#9415,2.4999999999999) ;
#795=CIRCLE('',#9418,2.49999999999919) ;
#796=CIRCLE('',#9420,17.4999999999923) ;
#797=CIRCLE('',#9422,2.49999999999998) ;
#798=CIRCLE('',#9425,2.49999999999996) ;
#799=CIRCLE('',#9427,78.9146368237009) ;
#800=CIRCLE('',#9429,2.49999999999968) ;
#801=CIRCLE('',#9432,2.49999999999912) ;
#802=CIRCLE('',#9434,17.4999999999908) ;
#803=CIRCLE('',#9436,2.49999999999996) ;
#804=CIRCLE('',#9439,2.49999999999987) ;
#805=CIRCLE('',#9441,78.9146368237006) ;
#806=CIRCLE('',#9443,2.50000000000016) ;
#807=CIRCLE('',#9446,2.49999999999888) ;
#808=CIRCLE('',#9448,83.314636823702) ;
#809=CIRCLE('',#9450,81.1146368237019) ;
#810=CIRCLE('',#9451,81.1146368237019) ;
#1105=FACE_OUTER_BOUND('',#1622,.T.) ;
#1106=FACE_OUTER_BOUND('',#1623,.T.) ;
#1107=FACE_OUTER_BOUND('',#1624,.T.) ;
#1108=FACE_OUTER_BOUND('',#1625,.T.) ;
#1109=FACE_OUTER_BOUND('',#1626,.T.) ;
#1110=FACE_OUTER_BOUND('',#1627,.T.) ;
#1111=FACE_OUTER_BOUND('',#1628,.T.) ;
#1112=FACE_OUTER_BOUND('',#1629,.T.) ;
#1113=FACE_OUTER_BOUND('',#1630,.T.) ;
#1114=FACE_OUTER_BOUND('',#1631,.T.) ;
#1115=FACE_OUTER_BOUND('',#1632,.T.) ;
#1116=FACE_OUTER_BOUND('',#1633,.T.) ;
#1117=FACE_OUTER_BOUND('',#1634,.T.) ;
#1118=FACE_OUTER_BOUND('',#1635,.T.) ;
#1119=FACE_OUTER_BOUND('',#1636,.T.) ;
#1120=FACE_OUTER_BOUND('',#1637,.T.) ;
#1121=FACE_OUTER_BOUND('',#1638,.T.) ;
#1122=FACE_OUTER_BOUND('',#1639,.T.) ;
#1123=FACE_OUTER_BOUND('',#1640,.T.) ;
#1124=FACE_OUTER_BOUND('',#1641,.T.) ;
#1125=FACE_OUTER_BOUND('',#1642,.T.) ;
#1126=FACE_OUTER_BOUND('',#1643,.T.) ;
#1127=FACE_OUTER_BOUND('',#1644,.T.) ;
#1128=FACE_OUTER_BOUND('',#1645,.T.) ;
#1129=FACE_OUTER_BOUND('',#1646,.T.) ;
#1130=FACE_OUTER_BOUND('',#1647,.T.) ;
#1131=FACE_OUTER_BOUND('',#1648,.T.) ;
#1132=FACE_OUTER_BOUND('',#1649,.T.) ;
#1133=FACE_OUTER_BOUND('',#1650,.T.) ;
#1134=FACE_OUTER_BOUND('',#1651,.T.) ;
#1135=FACE_OUTER_BOUND('',#1652,.T.) ;
#1136=FACE_OUTER_BOUND('',#1653,.T.) ;
#1137=FACE_OUTER_BOUND('',#1654,.T.) ;
#1138=FACE_OUTER_BOUND('',#1655,.T.) ;
#1139=FACE_OUTER_BOUND('',#1656,.T.) ;
#1140=FACE_OUTER_BOUND('',#1657,.T.) ;
#1141=FACE_OUTER_BOUND('',#1658,.T.) ;
#1142=FACE_OUTER_BOUND('',#1659,.T.) ;
#1143=FACE_OUTER_BOUND('',#1660,.T.) ;
#1144=FACE_OUTER_BOUND('',#1661,.T.) ;
#1145=FACE_OUTER_BOUND('',#1662,.T.) ;
#1146=FACE_OUTER_BOUND('',#1663,.T.) ;
#1147=FACE_OUTER_BOUND('',#1664,.T.) ;
#1148=FACE_OUTER_BOUND('',#1665,.T.) ;
#1149=FACE_OUTER_BOUND('',#1666,.T.) ;
#1150=FACE_OUTER_BOUND('',#1667,.T.) ;
#1151=FACE_OUTER_BOUND('',#1668,.T.) ;
#1152=FACE_OUTER_BOUND('',#1669,.T.) ;
#1153=FACE_OUTER_BOUND('',#1670,.T.) ;
#1154=FACE_OUTER_BOUND('',#1671,.T.) ;
#1155=FACE_OUTER_BOUND('',#1672,.T.) ;
#1156=FACE_OUTER_BOUND('',#1673,.T.) ;
#1157=FACE_OUTER_BOUND('',#1674,.T.) ;
#1158=FACE_OUTER_BOUND('',#1675,.T.) ;
#1159=FACE_OUTER_BOUND('',#1676,.T.) ;
#1160=FACE_OUTER_BOUND('',#1677,.T.) ;
#1161=FACE_OUTER_BOUND('',#1678,.T.) ;
#1162=FACE_OUTER_BOUND('',#1679,.T.) ;
#1163=FACE_OUTER_BOUND('',#1680,.T.) ;
#1164=FACE_OUTER_BOUND('',#1681,.T.) ;
#1165=FACE_OUTER_BOUND('',#1682,.T.) ;
#1166=FACE_OUTER_BOUND('',#1683,.T.) ;
#1167=FACE_OUTER_BOUND('',#1684,.T.) ;
#1168=FACE_OUTER_BOUND('',#1685,.T.) ;
#1169=FACE_OUTER_BOUND('',#1686,.T.) ;
#1170=FACE_OUTER_BOUND('',#1687,.T.) ;
#1171=FACE_OUTER_BOUND('',#1688,.T.) ;
#1172=FACE_OUTER_BOUND('',#1689,.T.) ;
#1173=FACE_OUTER_BOUND('',#1690,.T.) ;
#1174=FACE_OUTER_BOUND('',#1691,.T.) ;
#1175=FACE_OUTER_BOUND('',#1692,.T.) ;
#1176=FACE_OUTER_BOUND('',#1693,.T.) ;
#1177=FACE_OUTER_BOUND('',#1694,.T.) ;
#1178=FACE_OUTER_BOUND('',#1695,.T.) ;
#1179=FACE_OUTER_BOUND('',#1696,.T.) ;
#1180=FACE_OUTER_BOUND('',#1697,.T.) ;
#1181=FACE_OUTER_BOUND('',#1698,.T.) ;
#1182=FACE_OUTER_BOUND('',#1699,.T.) ;
#1183=FACE_OUTER_BOUND('',#1700,.T.) ;
#1184=FACE_OUTER_BOUND('',#1701,.T.) ;
#1185=FACE_OUTER_BOUND('',#1702,.T.) ;
#1186=FACE_OUTER_BOUND('',#1703,.T.) ;
#1187=FACE_OUTER_BOUND('',#1704,.T.) ;
#1188=FACE_OUTER_BOUND('',#1705,.T.) ;
#1189=FACE_OUTER_BOUND('',#1706,.T.) ;
#1190=FACE_OUTER_BOUND('',#1707,.T.) ;
#1191=FACE_OUTER_BOUND('',#1708,.T.) ;
#1192=FACE_OUTER_BOUND('',#1709,.T.) ;
#1193=FACE_OUTER_BOUND('',#1710,.T.) ;
#1194=FACE_OUTER_BOUND('',#1711,.T.) ;
#1195=FACE_OUTER_BOUND('',#1712,.T.) ;
#1196=FACE_OUTER_BOUND('',#1713,.T.) ;
#1197=FACE_OUTER_BOUND('',#1714,.T.) ;
#1198=FACE_OUTER_BOUND('',#1715,.T.) ;
#1199=FACE_OUTER_BOUND('',#1716,.T.) ;
#1200=FACE_OUTER_BOUND('',#1717,.T.) ;
#1201=FACE_OUTER_BOUND('',#1718,.T.) ;
#1202=FACE_OUTER_BOUND('',#1719,.T.) ;
#1203=FACE_OUTER_BOUND('',#1720,.T.) ;
#1204=FACE_OUTER_BOUND('',#1721,.T.) ;
#1205=FACE_OUTER_BOUND('',#1722,.T.) ;
#1206=FACE_OUTER_BOUND('',#1723,.T.) ;
#1207=FACE_OUTER_BOUND('',#1724,.T.) ;
#1208=FACE_OUTER_BOUND('',#1725,.T.) ;
#1209=FACE_OUTER_BOUND('',#1726,.T.) ;
#1210=FACE_OUTER_BOUND('',#1727,.T.) ;
#1211=FACE_OUTER_BOUND('',#1728,.T.) ;
#1212=FACE_OUTER_BOUND('',#1729,.T.) ;
#1213=FACE_OUTER_BOUND('',#1730,.T.) ;
#1214=FACE_OUTER_BOUND('',#1731,.T.) ;
#1215=FACE_OUTER_BOUND('',#1732,.T.) ;
#1216=FACE_OUTER_BOUND('',#1733,.T.) ;
#1217=FACE_OUTER_BOUND('',#1734,.T.) ;
#1218=FACE_OUTER_BOUND('',#1735,.T.) ;
#1219=FACE_OUTER_BOUND('',#1736,.T.) ;
#1220=FACE_OUTER_BOUND('',#1737,.T.) ;
#1221=FACE_OUTER_BOUND('',#1738,.T.) ;
#1222=FACE_OUTER_BOUND('',#1739,.T.) ;
#1223=FACE_OUTER_BOUND('',#1740,.T.) ;
#1224=FACE_OUTER_BOUND('',#1741,.T.) ;
#1225=FACE_OUTER_BOUND('',#1742,.T.) ;
#1226=FACE_OUTER_BOUND('',#1743,.T.) ;
#1227=FACE_OUTER_BOUND('',#1744,.T.) ;
#1228=FACE_OUTER_BOUND('',#1745,.T.) ;
#1229=FACE_OUTER_BOUND('',#1746,.T.) ;
#1230=FACE_OUTER_BOUND('',#1747,.T.) ;
#1231=FACE_OUTER_BOUND('',#1748,.T.) ;
#1232=FACE_OUTER_BOUND('',#1749,.T.) ;
#1233=FACE_OUTER_BOUND('',#1750,.T.) ;
#1234=FACE_OUTER_BOUND('',#1751,.T.) ;
#1235=FACE_OUTER_BOUND('',#1752,.T.) ;
#1236=FACE_OUTER_BOUND('',#1753,.T.) ;
#1237=FACE_OUTER_BOUND('',#1754,.T.) ;
#1238=FACE_OUTER_BOUND('',#1755,.T.) ;
#1239=FACE_OUTER_BOUND('',#1756,.T.) ;
#1240=FACE_OUTER_BOUND('',#1757,.T.) ;
#1241=FACE_OUTER_BOUND('',#1758,.T.) ;
#1242=FACE_OUTER_BOUND('',#1759,.T.) ;
#1243=FACE_OUTER_BOUND('',#1760,.T.) ;
#1244=FACE_OUTER_BOUND('',#1761,.T.) ;
#1245=FACE_OUTER_BOUND('',#1762,.T.) ;
#1246=FACE_OUTER_BOUND('',#1763,.T.) ;
#1247=FACE_OUTER_BOUND('',#1764,.T.) ;
#1248=FACE_OUTER_BOUND('',#1765,.T.) ;
#1249=FACE_OUTER_BOUND('',#1766,.T.) ;
#1250=FACE_OUTER_BOUND('',#1767,.T.) ;
#1251=FACE_OUTER_BOUND('',#1768,.T.) ;
#1252=FACE_OUTER_BOUND('',#1769,.T.) ;
#1253=FACE_OUTER_BOUND('',#1770,.T.) ;
#1254=FACE_OUTER_BOUND('',#1771,.T.) ;
#1255=FACE_OUTER_BOUND('',#1772,.T.) ;
#1256=FACE_OUTER_BOUND('',#1773,.T.) ;
#1257=FACE_OUTER_BOUND('',#1774,.T.) ;
#1258=FACE_OUTER_BOUND('',#1775,.T.) ;
#1259=FACE_OUTER_BOUND('',#1776,.T.) ;
#1260=FACE_OUTER_BOUND('',#1777,.T.) ;
#1261=FACE_OUTER_BOUND('',#1778,.T.) ;
#1262=FACE_OUTER_BOUND('',#1779,.T.) ;
#1263=FACE_OUTER_BOUND('',#1780,.T.) ;
#1264=FACE_OUTER_BOUND('',#1781,.T.) ;
#1265=FACE_OUTER_BOUND('',#1782,.T.) ;
#1266=FACE_OUTER_BOUND('',#1783,.T.) ;
#1267=FACE_OUTER_BOUND('',#1784,.T.) ;
#1268=FACE_OUTER_BOUND('',#1785,.T.) ;
#1269=FACE_OUTER_BOUND('',#1786,.T.) ;
#1270=FACE_OUTER_BOUND('',#1787,.T.) ;
#1271=FACE_OUTER_BOUND('',#1788,.T.) ;
#1272=FACE_OUTER_BOUND('',#1789,.T.) ;
#1273=FACE_OUTER_BOUND('',#1790,.T.) ;
#1274=FACE_OUTER_BOUND('',#1791,.T.) ;
#1275=FACE_OUTER_BOUND('',#1792,.T.) ;
#1276=FACE_OUTER_BOUND('',#1793,.T.) ;
#1277=FACE_OUTER_BOUND('',#1794,.T.) ;
#1278=FACE_OUTER_BOUND('',#1795,.T.) ;
#1279=FACE_OUTER_BOUND('',#1796,.T.) ;
#1280=FACE_OUTER_BOUND('',#1797,.T.) ;
#1281=FACE_OUTER_BOUND('',#1798,.T.) ;
#1282=FACE_OUTER_BOUND('',#1799,.T.) ;
#1283=FACE_OUTER_BOUND('',#1800,.T.) ;
#1284=FACE_OUTER_BOUND('',#1801,.T.) ;
#1285=FACE_OUTER_BOUND('',#1802,.T.) ;
#1286=FACE_OUTER_BOUND('',#1809,.T.) ;
#1287=FACE_OUTER_BOUND('',#1811,.T.) ;
#1288=FACE_OUTER_BOUND('',#1812,.T.) ;
#1289=FACE_OUTER_BOUND('',#1813,.T.) ;
#1290=FACE_OUTER_BOUND('',#1814,.T.) ;
#1291=FACE_OUTER_BOUND('',#1815,.T.) ;
#1292=FACE_OUTER_BOUND('',#1816,.T.) ;
#1293=FACE_OUTER_BOUND('',#1817,.T.) ;
#1294=FACE_OUTER_BOUND('',#1818,.T.) ;
#1295=FACE_OUTER_BOUND('',#1819,.T.) ;
#1296=FACE_OUTER_BOUND('',#1820,.T.) ;
#1297=FACE_OUTER_BOUND('',#1821,.T.) ;
#1298=FACE_OUTER_BOUND('',#1822,.T.) ;
#1299=FACE_OUTER_BOUND('',#1823,.T.) ;
#1300=FACE_OUTER_BOUND('',#1824,.T.) ;
#1301=FACE_OUTER_BOUND('',#1825,.T.) ;
#1302=FACE_OUTER_BOUND('',#1826,.T.) ;
#1303=FACE_OUTER_BOUND('',#1827,.T.) ;
#1304=FACE_OUTER_BOUND('',#1828,.T.) ;
#1305=FACE_OUTER_BOUND('',#1829,.T.) ;
#1306=FACE_OUTER_BOUND('',#1830,.T.) ;
#1307=FACE_OUTER_BOUND('',#1831,.T.) ;
#1308=FACE_OUTER_BOUND('',#1832,.T.) ;
#1309=FACE_OUTER_BOUND('',#1833,.T.) ;
#1310=FACE_OUTER_BOUND('',#1834,.T.) ;
#1311=FACE_OUTER_BOUND('',#1835,.T.) ;
#1312=FACE_OUTER_BOUND('',#1836,.T.) ;
#1313=FACE_OUTER_BOUND('',#1837,.T.) ;
#1314=FACE_OUTER_BOUND('',#1838,.T.) ;
#1315=FACE_OUTER_BOUND('',#1839,.T.) ;
#1316=FACE_OUTER_BOUND('',#1840,.T.) ;
#1317=FACE_OUTER_BOUND('',#1841,.T.) ;
#1318=FACE_OUTER_BOUND('',#1842,.T.) ;
#1319=FACE_OUTER_BOUND('',#1843,.T.) ;
#1320=FACE_OUTER_BOUND('',#1844,.T.) ;
#1321=FACE_OUTER_BOUND('',#1845,.T.) ;
#1322=FACE_OUTER_BOUND('',#1846,.T.) ;
#1323=FACE_OUTER_BOUND('',#1847,.T.) ;
#1324=FACE_OUTER_BOUND('',#1848,.T.) ;
#1325=FACE_OUTER_BOUND('',#1849,.T.) ;
#1326=FACE_OUTER_BOUND('',#1850,.T.) ;
#1327=FACE_OUTER_BOUND('',#1851,.T.) ;
#1328=FACE_OUTER_BOUND('',#1852,.T.) ;
#1329=FACE_OUTER_BOUND('',#1853,.T.) ;
#1330=FACE_OUTER_BOUND('',#1854,.T.) ;
#1331=FACE_OUTER_BOUND('',#1856,.T.) ;
#1622=EDGE_LOOP('',(#6782,#6783,#6784,#6785)) ;
#1623=EDGE_LOOP('',(#6786,#6787,#6788,#6789)) ;
#1624=EDGE_LOOP('',(#6790,#6791,#6792,#6793)) ;
#1625=EDGE_LOOP('',(#6794,#6795,#6796,#6797)) ;
#1626=EDGE_LOOP('',(#6798,#6799,#6800,#6801)) ;
#1627=EDGE_LOOP('',(#6802,#6803,#6804,#6805)) ;
#1628=EDGE_LOOP('',(#6806,#6807,#6808,#6809)) ;
#1629=EDGE_LOOP('',(#6810,#6811,#6812,#6813)) ;
#1630=EDGE_LOOP('',(#6814,#6815,#6816,#6817)) ;
#1631=EDGE_LOOP('',(#6818,#6819,#6820,#6821)) ;
#1632=EDGE_LOOP('',(#6822,#6823,#6824,#6825)) ;
#1633=EDGE_LOOP('',(#6826,#6827,#6828,#6829)) ;
#1634=EDGE_LOOP('',(#6830,#6831,#6832,#6833)) ;
#1635=EDGE_LOOP('',(#6834,#6835,#6836,#6837)) ;
#1636=EDGE_LOOP('',(#6838,#6839,#6840,#6841)) ;
#1637=EDGE_LOOP('',(#6842,#6843,#6844,#6845)) ;
#1638=EDGE_LOOP('',(#6846,#6847,#6848,#6849)) ;
#1639=EDGE_LOOP('',(#6850,#6851,#6852,#6853)) ;
#1640=EDGE_LOOP('',(#6854,#6855,#6856,#6857)) ;
#1641=EDGE_LOOP('',(#6858,#6859,#6860,#6861)) ;
#1642=EDGE_LOOP('',(#6862,#6863,#6864,#6865)) ;
#1643=EDGE_LOOP('',(#6866,#6867,#6868,#6869)) ;
#1644=EDGE_LOOP('',(#6870,#6871,#6872,#6873)) ;
#1645=EDGE_LOOP('',(#6874,#6875,#6876,#6877)) ;
#1646=EDGE_LOOP('',(#6878,#6879,#6880,#6881)) ;
#1647=EDGE_LOOP('',(#6882,#6883,#6884,#6885)) ;
#1648=EDGE_LOOP('',(#6886,#6887,#6888,#6889)) ;
#1649=EDGE_LOOP('',(#6890,#6891,#6892,#6893)) ;
#1650=EDGE_LOOP('',(#6894,#6895,#6896,#6897)) ;
#1651=EDGE_LOOP('',(#6898,#6899,#6900,#6901)) ;
#1652=EDGE_LOOP('',(#6902,#6903,#6904,#6905)) ;
#1653=EDGE_LOOP('',(#6906,#6907,#6908,#6909)) ;
#1654=EDGE_LOOP('',(#6910,#6911,#6912,#6913)) ;
#1655=EDGE_LOOP('',(#6914,#6915,#6916,#6917)) ;
#1656=EDGE_LOOP('',(#6918,#6919,#6920,#6921)) ;
#1657=EDGE_LOOP('',(#6922,#6923,#6924,#6925)) ;
#1658=EDGE_LOOP('',(#6926,#6927,#6928,#6929)) ;
#1659=EDGE_LOOP('',(#6930,#6931,#6932,#6933)) ;
#1660=EDGE_LOOP('',(#6934,#6935,#6936,#6937)) ;
#1661=EDGE_LOOP('',(#6938,#6939,#6940,#6941)) ;
#1662=EDGE_LOOP('',(#6942,#6943,#6944,#6945)) ;
#1663=EDGE_LOOP('',(#6946,#6947,#6948,#6949)) ;
#1664=EDGE_LOOP('',(#6950,#6951,#6952,#6953)) ;
#1665=EDGE_LOOP('',(#6954,#6955,#6956,#6957)) ;
#1666=EDGE_LOOP('',(#6958,#6959,#6960,#6961)) ;
#1667=EDGE_LOOP('',(#6962,#6963,#6964,#6965)) ;
#1668=EDGE_LOOP('',(#6966,#6967,#6968,#6969)) ;
#1669=EDGE_LOOP('',(#6970,#6971,#6972,#6973)) ;
#1670=EDGE_LOOP('',(#6974,#6975,#6976,#6977)) ;
#1671=EDGE_LOOP('',(#6978,#6979,#6980,#6981)) ;
#1672=EDGE_LOOP('',(#6982,#6983,#6984,#6985)) ;
#1673=EDGE_LOOP('',(#6986,#6987,#6988,#6989)) ;
#1674=EDGE_LOOP('',(#6990,#6991,#6992,#6993)) ;
#1675=EDGE_LOOP('',(#6994,#6995,#6996,#6997)) ;
#1676=EDGE_LOOP('',(#6998,#6999,#7000,#7001)) ;
#1677=EDGE_LOOP('',(#7002,#7003,#7004,#7005)) ;
#1678=EDGE_LOOP('',(#7006,#7007,#7008,#7009)) ;
#1679=EDGE_LOOP('',(#7010,#7011,#7012,#7013)) ;
#1680=EDGE_LOOP('',(#7014,#7015,#7016,#7017)) ;
#1681=EDGE_LOOP('',(#7018,#7019,#7020,#7021)) ;
#1682=EDGE_LOOP('',(#7022,#7023,#7024,#7025)) ;
#1683=EDGE_LOOP('',(#7026,#7027,#7028,#7029)) ;
#1684=EDGE_LOOP('',(#7030,#7031,#7032,#7033)) ;
#1685=EDGE_LOOP('',(#7034,#7035,#7036,#7037)) ;
#1686=EDGE_LOOP('',(#7038,#7039,#7040,#7041)) ;
#1687=EDGE_LOOP('',(#7042,#7043,#7044,#7045)) ;
#1688=EDGE_LOOP('',(#7046,#7047,#7048,#7049)) ;
#1689=EDGE_LOOP('',(#7050,#7051,#7052,#7053)) ;
#1690=EDGE_LOOP('',(#7054,#7055,#7056,#7057)) ;
#1691=EDGE_LOOP('',(#7058,#7059,#7060,#7061)) ;
#1692=EDGE_LOOP('',(#7062,#7063,#7064,#7065)) ;
#1693=EDGE_LOOP('',(#7066,#7067,#7068,#7069)) ;
#1694=EDGE_LOOP('',(#7070,#7071,#7072,#7073)) ;
#1695=EDGE_LOOP('',(#7074,#7075,#7076,#7077)) ;
#1696=EDGE_LOOP('',(#7078,#7079,#7080,#7081)) ;
#1697=EDGE_LOOP('',(#7082,#7083,#7084,#7085)) ;
#1698=EDGE_LOOP('',(#7086,#7087,#7088,#7089)) ;
#1699=EDGE_LOOP('',(#7090,#7091,#7092,#7093)) ;
#1700=EDGE_LOOP('',(#7094,#7095,#7096,#7097)) ;
#1701=EDGE_LOOP('',(#7098,#7099,#7100,#7101)) ;
#1702=EDGE_LOOP('',(#7102,#7103,#7104,#7105)) ;
#1703=EDGE_LOOP('',(#7106,#7107,#7108,#7109)) ;
#1704=EDGE_LOOP('',(#7110,#7111,#7112,#7113)) ;
#1705=EDGE_LOOP('',(#7114,#7115,#7116,#7117)) ;
#1706=EDGE_LOOP('',(#7118,#7119,#7120,#7121)) ;
#1707=EDGE_LOOP('',(#7122,#7123,#7124,#7125)) ;
#1708=EDGE_LOOP('',(#7126,#7127,#7128,#7129)) ;
#1709=EDGE_LOOP('',(#7130,#7131,#7132,#7133)) ;
#1710=EDGE_LOOP('',(#7134,#7135,#7136,#7137)) ;
#1711=EDGE_LOOP('',(#7138,#7139,#7140,#7141)) ;
#1712=EDGE_LOOP('',(#7142,#7143,#7144,#7145)) ;
#1713=EDGE_LOOP('',(#7146,#7147,#7148,#7149)) ;
#1714=EDGE_LOOP('',(#7150,#7151,#7152,#7153)) ;
#1715=EDGE_LOOP('',(#7154,#7155,#7156,#7157)) ;
#1716=EDGE_LOOP('',(#7158,#7159,#7160,#7161)) ;
#1717=EDGE_LOOP('',(#7162,#7163,#7164,#7165)) ;
#1718=EDGE_LOOP('',(#7166,#7167,#7168,#7169)) ;
#1719=EDGE_LOOP('',(#7170,#7171,#7172,#7173)) ;
#1720=EDGE_LOOP('',(#7174,#7175,#7176,#7177)) ;
#1721=EDGE_LOOP('',(#7178,#7179,#7180,#7181)) ;
#1722=EDGE_LOOP('',(#7182,#7183,#7184,#7185)) ;
#1723=EDGE_LOOP('',(#7186,#7187,#7188,#7189)) ;
#1724=EDGE_LOOP('',(#7190,#7191,#7192,#7193)) ;
#1725=EDGE_LOOP('',(#7194,#7195,#7196,#7197)) ;
#1726=EDGE_LOOP('',(#7198,#7199,#7200,#7201)) ;
#1727=EDGE_LOOP('',(#7202,#7203,#7204,#7205)) ;
#1728=EDGE_LOOP('',(#7206,#7207,#7208,#7209)) ;
#1729=EDGE_LOOP('',(#7210,#7211,#7212,#7213)) ;
#1730=EDGE_LOOP('',(#7214,#7215,#7216,#7217)) ;
#1731=EDGE_LOOP('',(#7218,#7219,#7220,#7221)) ;
#1732=EDGE_LOOP('',(#7222,#7223,#7224,#7225)) ;
#1733=EDGE_LOOP('',(#7226,#7227,#7228,#7229)) ;
#1734=EDGE_LOOP('',(#7230,#7231,#7232,#7233)) ;
#1735=EDGE_LOOP('',(#7234,#7235,#7236,#7237)) ;
#1736=EDGE_LOOP('',(#7238,#7239,#7240,#7241)) ;
#1737=EDGE_LOOP('',(#7242,#7243,#7244,#7245)) ;
#1738=EDGE_LOOP('',(#7246,#7247,#7248,#7249)) ;
#1739=EDGE_LOOP('',(#7250,#7251,#7252,#7253)) ;
#1740=EDGE_LOOP('',(#7254,#7255,#7256,#7257)) ;
#1741=EDGE_LOOP('',(#7258,#7259,#7260,#7261)) ;
#1742=EDGE_LOOP('',(#7262,#7263,#7264,#7265)) ;
#1743=EDGE_LOOP('',(#7266,#7267,#7268,#7269)) ;
#1744=EDGE_LOOP('',(#7270,#7271,#7272,#7273)) ;
#1745=EDGE_LOOP('',(#7274,#7275,#7276,#7277)) ;
#1746=EDGE_LOOP('',(#7278,#7279,#7280,#7281)) ;
#1747=EDGE_LOOP('',(#7282,#7283,#7284,#7285)) ;
#1748=EDGE_LOOP('',(#7286,#7287,#7288,#7289)) ;
#1749=EDGE_LOOP('',(#7290,#7291,#7292,#7293)) ;
#1750=EDGE_LOOP('',(#7294,#7295,#7296,#7297)) ;
#1751=EDGE_LOOP('',(#7298,#7299,#7300,#7301)) ;
#1752=EDGE_LOOP('',(#7302,#7303,#7304,#7305)) ;
#1753=EDGE_LOOP('',(#7306,#7307,#7308,#7309)) ;
#1754=EDGE_LOOP('',(#7310,#7311,#7312,#7313)) ;
#1755=EDGE_LOOP('',(#7314,#7315,#7316,#7317)) ;
#1756=EDGE_LOOP('',(#7318,#7319,#7320,#7321)) ;
#1757=EDGE_LOOP('',(#7322,#7323,#7324,#7325)) ;
#1758=EDGE_LOOP('',(#7326,#7327,#7328,#7329)) ;
#1759=EDGE_LOOP('',(#7330,#7331,#7332,#7333)) ;
#1760=EDGE_LOOP('',(#7334,#7335,#7336,#7337)) ;
#1761=EDGE_LOOP('',(#7338,#7339,#7340,#7341)) ;
#1762=EDGE_LOOP('',(#7342,#7343,#7344,#7345)) ;
#1763=EDGE_LOOP('',(#7346,#7347,#7348,#7349)) ;
#1764=EDGE_LOOP('',(#7350,#7351,#7352,#7353)) ;
#1765=EDGE_LOOP('',(#7354,#7355,#7356,#7357)) ;
#1766=EDGE_LOOP('',(#7358,#7359,#7360,#7361)) ;
#1767=EDGE_LOOP('',(#7362,#7363,#7364,#7365)) ;
#1768=EDGE_LOOP('',(#7366,#7367,#7368,#7369)) ;
#1769=EDGE_LOOP('',(#7370,#7371,#7372,#7373)) ;
#1770=EDGE_LOOP('',(#7374,#7375,#7376,#7377)) ;
#1771=EDGE_LOOP('',(#7378,#7379,#7380,#7381)) ;
#1772=EDGE_LOOP('',(#7382,#7383,#7384,#7385)) ;
#1773=EDGE_LOOP('',(#7386,#7387,#7388,#7389)) ;
#1774=EDGE_LOOP('',(#7390,#7391,#7392,#7393)) ;
#1775=EDGE_LOOP('',(#7394,#7395,#7396,#7397)) ;
#1776=EDGE_LOOP('',(#7398,#7399,#7400,#7401)) ;
#1777=EDGE_LOOP('',(#7402,#7403,#7404,#7405)) ;
#1778=EDGE_LOOP('',(#7406,#7407,#7408,#7409)) ;
#1779=EDGE_LOOP('',(#7410,#7411,#7412,#7413)) ;
#1780=EDGE_LOOP('',(#7414,#7415,#7416,#7417)) ;
#1781=EDGE_LOOP('',(#7418,#7419,#7420,#7421)) ;
#1782=EDGE_LOOP('',(#7422,#7423,#7424,#7425)) ;
#1783=EDGE_LOOP('',(#7426,#7427,#7428,#7429)) ;
#1784=EDGE_LOOP('',(#7430,#7431,#7432,#7433)) ;
#1785=EDGE_LOOP('',(#7434,#7435,#7436,#7437)) ;
#1786=EDGE_LOOP('',(#7438,#7439,#7440,#7441)) ;
#1787=EDGE_LOOP('',(#7442,#7443,#7444,#7445)) ;
#1788=EDGE_LOOP('',(#7446,#7447,#7448,#7449)) ;
#1789=EDGE_LOOP('',(#7450,#7451,#7452,#7453)) ;
#1790=EDGE_LOOP('',(#7454,#7455,#7456,#7457)) ;
#1791=EDGE_LOOP('',(#7458,#7459,#7460,#7461)) ;
#1792=EDGE_LOOP('',(#7462,#7463,#7464,#7465)) ;
#1793=EDGE_LOOP('',(#7466,#7467,#7468,#7469)) ;
#1794=EDGE_LOOP('',(#7470,#7471,#7472,#7473)) ;
#1795=EDGE_LOOP('',(#7474,#7475,#7476,#7477)) ;
#1796=EDGE_LOOP('',(#7478,#7479,#7480,#7481)) ;
#1797=EDGE_LOOP('',(#7482,#7483,#7484,#7485)) ;
#1798=EDGE_LOOP('',(#7486,#7487,#7488,#7489)) ;
#1799=EDGE_LOOP('',(#7490,#7491,#7492,#7493)) ;
#1800=EDGE_LOOP('',(#7494,#7495,#7496,#7497)) ;
#1801=EDGE_LOOP('',(#7498,#7499,#7500,#7501)) ;
#1802=EDGE_LOOP('',(#7502,#7503,#7504,#7505,#7506,#7507,#7508,#7509,#7510,
#7511,#7512,#7513,#7514,#7515,#7516,#7517,#7518,#7519,#7520,#7521,#7522,
#7523,#7524,#7525,#7526,#7527,#7528,#7529,#7530,#7531,#7532,#7533,#7534,
#7535,#7536,#7537,#7538,#7539,#7540,#7541,#7542,#7543,#7544,#7545,#7546,
#7547,#7548,#7549,#7550,#7551,#7552,#7553,#7554,#7555,#7556,#7557,#7558,
#7559,#7560,#7561,#7562,#7563,#7564,#7565,#7566,#7567,#7568,#7569,#7570,
#7571,#7572,#7573,#7574,#7575,#7576,#7577,#7578,#7579,#7580,#7581,#7582,
#7583,#7584,#7585,#7586,#7587,#7588,#7589,#7590,#7591,#7592,#7593,#7594,
#7595,#7596,#7597,#7598,#7599,#7600,#7601,#7602,#7603,#7604,#7605,#7606,
#7607,#7608,#7609,#7610,#7611,#7612,#7613,#7614,#7615,#7616,#7617,#7618,
#7619,#7620,#7621,#7622,#7623,#7624,#7625,#7626,#7627,#7628,#7629,#7630,
#7631,#7632,#7633,#7634,#7635,#7636,#7637,#7638,#7639,#7640,#7641,#7642,
#7643,#7644,#7645,#7646,#7647,#7648,#7649,#7650,#7651,#7652,#7653,#7654,
#7655,#7656,#7657,#7658,#7659,#7660,#7661,#7662,#7663,#7664,#7665,#7666,
#7667,#7668,#7669,#7670,#7671,#7672,#7673,#7674,#7675,#7676,#7677,#7678,
#7679,#7680,#7681)) ;
#1803=EDGE_LOOP('',(#7682,#7683,#7684,#7685,#7686,#7687,#7688,#7689)) ;
#1804=EDGE_LOOP('',(#7690)) ;
#1805=EDGE_LOOP('',(#7691,#7692,#7693,#7694,#7695,#7696,#7697,#7698)) ;
#1806=EDGE_LOOP('',(#7699,#7700,#7701,#7702,#7703,#7704,#7705,#7706)) ;
#1807=EDGE_LOOP('',(#7707,#7708,#7709,#7710,#7711,#7712,#7713,#7714)) ;
#1808=EDGE_LOOP('',(#7715,#7716,#7717,#7718,#7719,#7720,#7721,#7722)) ;
#1809=EDGE_LOOP('',(#7723,#7724,#7725,#7726,#7727,#7728,#7729,#7730,#7731,
#7732,#7733,#7734,#7735,#7736,#7737,#7738,#7739,#7740,#7741,#7742,#7743,
#7744,#7745,#7746,#7747,#7748,#7749,#7750,#7751,#7752,#7753,#7754,#7755,
#7756,#7757,#7758,#7759,#7760,#7761,#7762,#7763,#7764,#7765,#7766,#7767,
#7768,#7769,#7770,#7771,#7772,#7773,#7774,#7775,#7776,#7777,#7778,#7779,
#7780,#7781,#7782,#7783,#7784,#7785,#7786,#7787,#7788,#7789,#7790,#7791,
#7792,#7793,#7794,#7795,#7796,#7797,#7798,#7799,#7800,#7801,#7802,#7803,
#7804,#7805,#7806,#7807,#7808,#7809,#7810,#7811,#7812,#7813,#7814,#7815,
#7816,#7817,#7818,#7819,#7820,#7821,#7822,#7823,#7824,#7825,#7826,#7827,
#7828,#7829,#7830,#7831,#7832,#7833,#7834,#7835,#7836,#7837,#7838,#7839,
#7840,#7841,#7842,#7843,#7844,#7845,#7846,#7847,#7848,#7849,#7850,#7851,
#7852,#7853,#7854,#7855,#7856,#7857,#7858,#7859,#7860,#7861,#7862,#7863,
#7864,#7865,#7866,#7867,#7868,#7869,#7870,#7871,#7872,#7873,#7874,#7875,
#7876,#7877,#7878,#7879,#7880,#7881,#7882,#7883,#7884,#7885,#7886,#7887,
#7888,#7889,#7890,#7891,#7892,#7893,#7894,#7895,#7896,#7897,#7898,#7899,
#7900,#7901,#7902)) ;
#1810=EDGE_LOOP('',(#7903)) ;
#1811=EDGE_LOOP('',(#7904,#7905,#7906,#7907)) ;
#1812=EDGE_LOOP('',(#7908,#7909,#7910,#7911)) ;
#1813=EDGE_LOOP('',(#7912,#7913,#7914,#7915)) ;
#1814=EDGE_LOOP('',(#7916,#7917,#7918,#7919)) ;
#1815=EDGE_LOOP('',(#7920,#7921,#7922,#7923)) ;
#1816=EDGE_LOOP('',(#7924,#7925,#7926,#7927)) ;
#1817=EDGE_LOOP('',(#7928,#7929,#7930,#7931)) ;
#1818=EDGE_LOOP('',(#7932,#7933,#7934,#7935)) ;
#1819=EDGE_LOOP('',(#7936,#7937,#7938,#7939)) ;
#1820=EDGE_LOOP('',(#7940,#7941,#7942,#7943)) ;
#1821=EDGE_LOOP('',(#7944,#7945,#7946,#7947)) ;
#1822=EDGE_LOOP('',(#7948,#7949,#7950,#7951)) ;
#1823=EDGE_LOOP('',(#7952,#7953,#7954,#7955)) ;
#1824=EDGE_LOOP('',(#7956,#7957,#7958,#7959)) ;
#1825=EDGE_LOOP('',(#7960,#7961,#7962,#7963)) ;
#1826=EDGE_LOOP('',(#7964,#7965,#7966,#7967)) ;
#1827=EDGE_LOOP('',(#7968,#7969,#7970,#7971)) ;
#1828=EDGE_LOOP('',(#7972,#7973,#7974,#7975)) ;
#1829=EDGE_LOOP('',(#7976,#7977,#7978,#7979)) ;
#1830=EDGE_LOOP('',(#7980,#7981,#7982,#7983)) ;
#1831=EDGE_LOOP('',(#7984,#7985,#7986,#7987)) ;
#1832=EDGE_LOOP('',(#7988,#7989,#7990,#7991)) ;
#1833=EDGE_LOOP('',(#7992,#7993,#7994,#7995)) ;
#1834=EDGE_LOOP('',(#7996,#7997,#7998,#7999)) ;
#1835=EDGE_LOOP('',(#8000,#8001,#8002,#8003)) ;
#1836=EDGE_LOOP('',(#8004,#8005,#8006,#8007)) ;
#1837=EDGE_LOOP('',(#8008,#8009,#8010,#8011)) ;
#1838=EDGE_LOOP('',(#8012,#8013,#8014,#8015)) ;
#1839=EDGE_LOOP('',(#8016,#8017,#8018,#8019)) ;
#1840=EDGE_LOOP('',(#8020,#8021,#8022,#8023)) ;
#1841=EDGE_LOOP('',(#8024,#8025,#8026,#8027)) ;
#1842=EDGE_LOOP('',(#8028,#8029,#8030,#8031)) ;
#1843=EDGE_LOOP('',(#8032,#8033,#8034,#8035)) ;
#1844=EDGE_LOOP('',(#8036,#8037,#8038,#8039)) ;
#1845=EDGE_LOOP('',(#8040,#8041,#8042,#8043)) ;
#1846=EDGE_LOOP('',(#8044,#8045,#8046,#8047)) ;
#1847=EDGE_LOOP('',(#8048,#8049,#8050,#8051)) ;
#1848=EDGE_LOOP('',(#8052,#8053,#8054,#8055)) ;
#1849=EDGE_LOOP('',(#8056,#8057,#8058,#8059)) ;
#1850=EDGE_LOOP('',(#8060,#8061,#8062,#8063)) ;
#1851=EDGE_LOOP('',(#8064,#8065,#8066,#8067)) ;
#1852=EDGE_LOOP('',(#8068,#8069,#8070,#8071)) ;
#1853=EDGE_LOOP('',(#8072,#8073,#8074,#8075)) ;
#1854=EDGE_LOOP('',(#8076)) ;
#1855=EDGE_LOOP('',(#8077)) ;
#1856=EDGE_LOOP('',(#8078)) ;
#1857=EDGE_LOOP('',(#8079,#8080,#8081,#8082,#8083,#8084,#8085,#8086)) ;
#1858=EDGE_LOOP('',(#8087)) ;
#1859=EDGE_LOOP('',(#8088,#8089,#8090,#8091,#8092,#8093,#8094,#8095)) ;
#1860=EDGE_LOOP('',(#8096,#8097,#8098,#8099,#8100,#8101,#8102,#8103)) ;
#1861=EDGE_LOOP('',(#8104,#8105,#8106,#8107,#8108,#8109,#8110,#8111)) ;
#1862=EDGE_LOOP('',(#8112,#8113,#8114,#8115,#8116,#8117,#8118,#8119)) ;
#2083=LINE('',#194856,#2786) ;
#2084=LINE('',#194858,#2787) ;
#2085=LINE('',#194860,#2788) ;
#2086=LINE('',#194861,#2789) ;
#2087=LINE('',#194875,#2790) ;
#2088=LINE('',#194879,#2791) ;
#2089=LINE('',#194881,#2792) ;
#2090=LINE('',#194882,#2793) ;
#2091=LINE('',#194885,#2794) ;
#2092=LINE('',#194887,#2795) ;
#2093=LINE('',#194888,#2796) ;
#2094=LINE('',#194902,#2797) ;
#2095=LINE('',#194906,#2798) ;
#2096=LINE('',#194908,#2799) ;
#2097=LINE('',#194909,#2800) ;
#2098=LINE('',#194912,#2801) ;
#2099=LINE('',#194914,#2802) ;
#2100=LINE('',#194915,#2803) ;
#2101=LINE('',#194929,#2804) ;
#2102=LINE('',#194933,#2805) ;
#2103=LINE('',#194935,#2806) ;
#2104=LINE('',#194936,#2807) ;
#2105=LINE('',#194939,#2808) ;
#2106=LINE('',#194941,#2809) ;
#2107=LINE('',#194942,#2810) ;
#2108=LINE('',#194956,#2811) ;
#2109=LINE('',#194960,#2812) ;
#2110=LINE('',#194962,#2813) ;
#2111=LINE('',#194963,#2814) ;
#2112=LINE('',#194966,#2815) ;
#2113=LINE('',#194968,#2816) ;
#2114=LINE('',#194969,#2817) ;
#2115=LINE('',#194983,#2818) ;
#2116=LINE('',#194987,#2819) ;
#2117=LINE('',#194989,#2820) ;
#2118=LINE('',#194990,#2821) ;
#2119=LINE('',#194993,#2822) ;
#2120=LINE('',#194995,#2823) ;
#2121=LINE('',#194996,#2824) ;
#2122=LINE('',#195010,#2825) ;
#2123=LINE('',#195014,#2826) ;
#2124=LINE('',#195016,#2827) ;
#2125=LINE('',#195017,#2828) ;
#2126=LINE('',#195020,#2829) ;
#2127=LINE('',#195022,#2830) ;
#2128=LINE('',#195023,#2831) ;
#2129=LINE('',#195037,#2832) ;
#2130=LINE('',#195041,#2833) ;
#2131=LINE('',#195043,#2834) ;
#2132=LINE('',#195044,#2835) ;
#2133=LINE('',#195047,#2836) ;
#2134=LINE('',#195049,#2837) ;
#2135=LINE('',#195050,#2838) ;
#2136=LINE('',#195064,#2839) ;
#2137=LINE('',#195068,#2840) ;
#2138=LINE('',#195070,#2841) ;
#2139=LINE('',#195071,#2842) ;
#2140=LINE('',#195074,#2843) ;
#2141=LINE('',#195076,#2844) ;
#2142=LINE('',#195077,#2845) ;
#2143=LINE('',#195091,#2846) ;
#2144=LINE('',#195095,#2847) ;
#2145=LINE('',#195097,#2848) ;
#2146=LINE('',#195098,#2849) ;
#2147=LINE('',#195101,#2850) ;
#2148=LINE('',#195103,#2851) ;
#2149=LINE('',#195104,#2852) ;
#2150=LINE('',#195118,#2853) ;
#2151=LINE('',#195122,#2854) ;
#2152=LINE('',#195124,#2855) ;
#2153=LINE('',#195125,#2856) ;
#2154=LINE('',#195128,#2857) ;
#2155=LINE('',#195130,#2858) ;
#2156=LINE('',#195131,#2859) ;
#2157=LINE('',#195145,#2860) ;
#2158=LINE('',#195149,#2861) ;
#2159=LINE('',#195151,#2862) ;
#2160=LINE('',#195152,#2863) ;
#2161=LINE('',#195155,#2864) ;
#2162=LINE('',#195157,#2865) ;
#2163=LINE('',#195158,#2866) ;
#2164=LINE('',#195172,#2867) ;
#2165=LINE('',#195176,#2868) ;
#2166=LINE('',#195178,#2869) ;
#2167=LINE('',#195179,#2870) ;
#2168=LINE('',#195182,#2871) ;
#2169=LINE('',#195184,#2872) ;
#2170=LINE('',#195185,#2873) ;
#2171=LINE('',#195199,#2874) ;
#2172=LINE('',#195203,#2875) ;
#2173=LINE('',#195205,#2876) ;
#2174=LINE('',#195206,#2877) ;
#2175=LINE('',#195209,#2878) ;
#2176=LINE('',#195211,#2879) ;
#2177=LINE('',#195212,#2880) ;
#2178=LINE('',#195226,#2881) ;
#2179=LINE('',#195230,#2882) ;
#2180=LINE('',#195232,#2883) ;
#2181=LINE('',#195233,#2884) ;
#2182=LINE('',#195236,#2885) ;
#2183=LINE('',#195238,#2886) ;
#2184=LINE('',#195239,#2887) ;
#2185=LINE('',#195253,#2888) ;
#2186=LINE('',#195257,#2889) ;
#2187=LINE('',#195259,#2890) ;
#2188=LINE('',#195260,#2891) ;
#2189=LINE('',#195263,#2892) ;
#2190=LINE('',#195265,#2893) ;
#2191=LINE('',#195266,#2894) ;
#2192=LINE('',#195280,#2895) ;
#2193=LINE('',#195284,#2896) ;
#2194=LINE('',#195286,#2897) ;
#2195=LINE('',#195287,#2898) ;
#2196=LINE('',#195290,#2899) ;
#2197=LINE('',#195292,#2900) ;
#2198=LINE('',#195293,#2901) ;
#2199=LINE('',#195307,#2902) ;
#2200=LINE('',#195311,#2903) ;
#2201=LINE('',#195313,#2904) ;
#2202=LINE('',#195314,#2905) ;
#2203=LINE('',#195317,#2906) ;
#2204=LINE('',#195319,#2907) ;
#2205=LINE('',#195320,#2908) ;
#2206=LINE('',#195334,#2909) ;
#2207=LINE('',#195338,#2910) ;
#2208=LINE('',#195340,#2911) ;
#2209=LINE('',#195341,#2912) ;
#2210=LINE('',#195344,#2913) ;
#2211=LINE('',#195346,#2914) ;
#2212=LINE('',#195347,#2915) ;
#2213=LINE('',#195361,#2916) ;
#2214=LINE('',#195365,#2917) ;
#2215=LINE('',#195367,#2918) ;
#2216=LINE('',#195368,#2919) ;
#2217=LINE('',#195371,#2920) ;
#2218=LINE('',#195373,#2921) ;
#2219=LINE('',#195374,#2922) ;
#2220=LINE('',#195388,#2923) ;
#2221=LINE('',#195392,#2924) ;
#2222=LINE('',#195394,#2925) ;
#2223=LINE('',#195395,#2926) ;
#2224=LINE('',#195398,#2927) ;
#2225=LINE('',#195400,#2928) ;
#2226=LINE('',#195401,#2929) ;
#2227=LINE('',#195415,#2930) ;
#2228=LINE('',#195419,#2931) ;
#2229=LINE('',#195421,#2932) ;
#2230=LINE('',#195422,#2933) ;
#2231=LINE('',#195425,#2934) ;
#2232=LINE('',#195427,#2935) ;
#2233=LINE('',#195428,#2936) ;
#2234=LINE('',#195442,#2937) ;
#2235=LINE('',#195446,#2938) ;
#2236=LINE('',#195448,#2939) ;
#2237=LINE('',#195449,#2940) ;
#2238=LINE('',#195452,#2941) ;
#2239=LINE('',#195454,#2942) ;
#2240=LINE('',#195455,#2943) ;
#2241=LINE('',#195469,#2944) ;
#2242=LINE('',#195473,#2945) ;
#2243=LINE('',#195475,#2946) ;
#2244=LINE('',#195476,#2947) ;
#2245=LINE('',#195479,#2948) ;
#2246=LINE('',#195481,#2949) ;
#2247=LINE('',#195482,#2950) ;
#2248=LINE('',#195496,#2951) ;
#2249=LINE('',#195500,#2952) ;
#2250=LINE('',#195502,#2953) ;
#2251=LINE('',#195503,#2954) ;
#2252=LINE('',#195506,#2955) ;
#2253=LINE('',#195508,#2956) ;
#2254=LINE('',#195509,#2957) ;
#2255=LINE('',#195523,#2958) ;
#2256=LINE('',#195527,#2959) ;
#2257=LINE('',#195529,#2960) ;
#2258=LINE('',#195530,#2961) ;
#2259=LINE('',#195533,#2962) ;
#2260=LINE('',#195535,#2963) ;
#2261=LINE('',#195536,#2964) ;
#2262=LINE('',#195550,#2965) ;
#2263=LINE('',#195554,#2966) ;
#2264=LINE('',#195556,#2967) ;
#2265=LINE('',#195557,#2968) ;
#2266=LINE('',#195560,#2969) ;
#2267=LINE('',#195562,#2970) ;
#2268=LINE('',#195563,#2971) ;
#2269=LINE('',#195577,#2972) ;
#2270=LINE('',#195581,#2973) ;
#2271=LINE('',#195583,#2974) ;
#2272=LINE('',#195584,#2975) ;
#2273=LINE('',#195587,#2976) ;
#2274=LINE('',#195589,#2977) ;
#2275=LINE('',#195590,#2978) ;
#2276=LINE('',#195604,#2979) ;
#2277=LINE('',#195608,#2980) ;
#2278=LINE('',#195610,#2981) ;
#2279=LINE('',#195611,#2982) ;
#2280=LINE('',#195614,#2983) ;
#2281=LINE('',#195616,#2984) ;
#2282=LINE('',#195617,#2985) ;
#2283=LINE('',#195631,#2986) ;
#2284=LINE('',#195635,#2987) ;
#2285=LINE('',#195637,#2988) ;
#2286=LINE('',#195638,#2989) ;
#2287=LINE('',#195641,#2990) ;
#2288=LINE('',#195643,#2991) ;
#2289=LINE('',#195644,#2992) ;
#2290=LINE('',#195658,#2993) ;
#2291=LINE('',#195662,#2994) ;
#2292=LINE('',#195664,#2995) ;
#2293=LINE('',#195665,#2996) ;
#2294=LINE('',#195668,#2997) ;
#2295=LINE('',#195670,#2998) ;
#2296=LINE('',#195671,#2999) ;
#2297=LINE('',#195685,#3000) ;
#2298=LINE('',#195689,#3001) ;
#2299=LINE('',#195691,#3002) ;
#2300=LINE('',#195692,#3003) ;
#2301=LINE('',#195695,#3004) ;
#2302=LINE('',#195697,#3005) ;
#2303=LINE('',#195698,#3006) ;
#2304=LINE('',#195712,#3007) ;
#2305=LINE('',#195716,#3008) ;
#2306=LINE('',#195718,#3009) ;
#2307=LINE('',#195719,#3010) ;
#2308=LINE('',#195722,#3011) ;
#2309=LINE('',#195724,#3012) ;
#2310=LINE('',#195725,#3013) ;
#2311=LINE('',#195739,#3014) ;
#2312=LINE('',#195743,#3015) ;
#2313=LINE('',#195745,#3016) ;
#2314=LINE('',#195746,#3017) ;
#2315=LINE('',#195749,#3018) ;
#2316=LINE('',#195751,#3019) ;
#2317=LINE('',#195752,#3020) ;
#2318=LINE('',#195766,#3021) ;
#2319=LINE('',#195770,#3022) ;
#2320=LINE('',#195772,#3023) ;
#2321=LINE('',#195773,#3024) ;
#2322=LINE('',#195776,#3025) ;
#2323=LINE('',#195778,#3026) ;
#2324=LINE('',#195779,#3027) ;
#2325=LINE('',#195793,#3028) ;
#2326=LINE('',#195797,#3029) ;
#2327=LINE('',#195799,#3030) ;
#2328=LINE('',#195800,#3031) ;
#2329=LINE('',#195803,#3032) ;
#2330=LINE('',#195805,#3033) ;
#2331=LINE('',#195806,#3034) ;
#2332=LINE('',#195820,#3035) ;
#2333=LINE('',#195824,#3036) ;
#2334=LINE('',#195826,#3037) ;
#2335=LINE('',#195827,#3038) ;
#2336=LINE('',#195830,#3039) ;
#2337=LINE('',#195832,#3040) ;
#2338=LINE('',#195833,#3041) ;
#2339=LINE('',#195847,#3042) ;
#2340=LINE('',#195851,#3043) ;
#2341=LINE('',#195853,#3044) ;
#2342=LINE('',#195854,#3045) ;
#2343=LINE('',#195857,#3046) ;
#2344=LINE('',#195859,#3047) ;
#2345=LINE('',#195860,#3048) ;
#2346=LINE('',#195874,#3049) ;
#2347=LINE('',#195878,#3050) ;
#2348=LINE('',#195880,#3051) ;
#2349=LINE('',#195881,#3052) ;
#2350=LINE('',#195884,#3053) ;
#2351=LINE('',#195886,#3054) ;
#2352=LINE('',#195887,#3055) ;
#2353=LINE('',#195901,#3056) ;
#2354=LINE('',#195905,#3057) ;
#2355=LINE('',#195907,#3058) ;
#2356=LINE('',#195908,#3059) ;
#2357=LINE('',#195911,#3060) ;
#2358=LINE('',#195913,#3061) ;
#2359=LINE('',#195914,#3062) ;
#2360=LINE('',#195928,#3063) ;
#2361=LINE('',#195932,#3064) ;
#2362=LINE('',#195934,#3065) ;
#2363=LINE('',#195935,#3066) ;
#2364=LINE('',#195938,#3067) ;
#2365=LINE('',#195940,#3068) ;
#2366=LINE('',#195941,#3069) ;
#2367=LINE('',#195955,#3070) ;
#2368=LINE('',#195959,#3071) ;
#2369=LINE('',#195961,#3072) ;
#2370=LINE('',#195962,#3073) ;
#2371=LINE('',#195965,#3074) ;
#2372=LINE('',#195967,#3075) ;
#2373=LINE('',#195968,#3076) ;
#2374=LINE('',#195982,#3077) ;
#2375=LINE('',#195986,#3078) ;
#2376=LINE('',#195988,#3079) ;
#2377=LINE('',#195989,#3080) ;
#2378=LINE('',#195992,#3081) ;
#2379=LINE('',#195994,#3082) ;
#2380=LINE('',#195995,#3083) ;
#2381=LINE('',#196009,#3084) ;
#2382=LINE('',#196013,#3085) ;
#2383=LINE('',#196015,#3086) ;
#2384=LINE('',#196016,#3087) ;
#2385=LINE('',#196019,#3088) ;
#2386=LINE('',#196021,#3089) ;
#2387=LINE('',#196022,#3090) ;
#2388=LINE('',#196036,#3091) ;
#2389=LINE('',#196040,#3092) ;
#2390=LINE('',#196042,#3093) ;
#2391=LINE('',#196043,#3094) ;
#2392=LINE('',#196046,#3095) ;
#2393=LINE('',#196048,#3096) ;
#2394=LINE('',#196049,#3097) ;
#2395=LINE('',#196063,#3098) ;
#2396=LINE('',#196067,#3099) ;
#2397=LINE('',#196069,#3100) ;
#2398=LINE('',#196070,#3101) ;
#2399=LINE('',#196073,#3102) ;
#2400=LINE('',#196075,#3103) ;
#2401=LINE('',#196076,#3104) ;
#2402=LINE('',#196090,#3105) ;
#2403=LINE('',#196094,#3106) ;
#2404=LINE('',#196096,#3107) ;
#2405=LINE('',#196097,#3108) ;
#2406=LINE('',#196100,#3109) ;
#2407=LINE('',#196102,#3110) ;
#2408=LINE('',#196103,#3111) ;
#2409=LINE('',#196117,#3112) ;
#2410=LINE('',#196121,#3113) ;
#2411=LINE('',#196123,#3114) ;
#2412=LINE('',#196124,#3115) ;
#2413=LINE('',#196127,#3116) ;
#2414=LINE('',#196129,#3117) ;
#2415=LINE('',#196130,#3118) ;
#2416=LINE('',#196144,#3119) ;
#2417=LINE('',#196148,#3120) ;
#2418=LINE('',#196150,#3121) ;
#2419=LINE('',#196151,#3122) ;
#2420=LINE('',#196154,#3123) ;
#2421=LINE('',#196156,#3124) ;
#2422=LINE('',#196157,#3125) ;
#2423=LINE('',#196171,#3126) ;
#2424=LINE('',#196175,#3127) ;
#2425=LINE('',#196177,#3128) ;
#2426=LINE('',#196178,#3129) ;
#2427=LINE('',#196181,#3130) ;
#2428=LINE('',#196183,#3131) ;
#2429=LINE('',#196184,#3132) ;
#2430=LINE('',#196198,#3133) ;
#2431=LINE('',#196202,#3134) ;
#2432=LINE('',#196204,#3135) ;
#2433=LINE('',#196205,#3136) ;
#2434=LINE('',#196208,#3137) ;
#2435=LINE('',#196210,#3138) ;
#2436=LINE('',#196211,#3139) ;
#2437=LINE('',#196225,#3140) ;
#2438=LINE('',#196229,#3141) ;
#2439=LINE('',#196231,#3142) ;
#2440=LINE('',#196232,#3143) ;
#2441=LINE('',#196235,#3144) ;
#2442=LINE('',#196237,#3145) ;
#2443=LINE('',#196238,#3146) ;
#2444=LINE('',#196252,#3147) ;
#2445=LINE('',#196256,#3148) ;
#2446=LINE('',#196258,#3149) ;
#2447=LINE('',#196259,#3150) ;
#2448=LINE('',#196262,#3151) ;
#2449=LINE('',#196264,#3152) ;
#2450=LINE('',#196265,#3153) ;
#2451=LINE('',#196279,#3154) ;
#2452=LINE('',#196283,#3155) ;
#2453=LINE('',#196285,#3156) ;
#2454=LINE('',#196286,#3157) ;
#2455=LINE('',#196289,#3158) ;
#2456=LINE('',#196291,#3159) ;
#2457=LINE('',#196292,#3160) ;
#2458=LINE('',#196306,#3161) ;
#2459=LINE('',#196310,#3162) ;
#2460=LINE('',#196312,#3163) ;
#2461=LINE('',#196313,#3164) ;
#2462=LINE('',#196316,#3165) ;
#2463=LINE('',#196318,#3166) ;
#2464=LINE('',#196319,#3167) ;
#2465=LINE('',#196333,#3168) ;
#2466=LINE('',#196337,#3169) ;
#2467=LINE('',#196339,#3170) ;
#2468=LINE('',#196340,#3171) ;
#2469=LINE('',#196343,#3172) ;
#2470=LINE('',#196345,#3173) ;
#2471=LINE('',#196346,#3174) ;
#2472=LINE('',#196360,#3175) ;
#2473=LINE('',#196364,#3176) ;
#2474=LINE('',#196366,#3177) ;
#2475=LINE('',#196367,#3178) ;
#2476=LINE('',#196370,#3179) ;
#2477=LINE('',#196372,#3180) ;
#2478=LINE('',#196373,#3181) ;
#2479=LINE('',#196387,#3182) ;
#2480=LINE('',#196391,#3183) ;
#2481=LINE('',#196393,#3184) ;
#2482=LINE('',#196394,#3185) ;
#2483=LINE('',#196397,#3186) ;
#2484=LINE('',#196399,#3187) ;
#2485=LINE('',#196400,#3188) ;
#2486=LINE('',#196414,#3189) ;
#2487=LINE('',#196418,#3190) ;
#2488=LINE('',#196420,#3191) ;
#2489=LINE('',#196421,#3192) ;
#2490=LINE('',#196424,#3193) ;
#2491=LINE('',#196426,#3194) ;
#2492=LINE('',#196427,#3195) ;
#2493=LINE('',#196441,#3196) ;
#2494=LINE('',#196445,#3197) ;
#2495=LINE('',#196447,#3198) ;
#2496=LINE('',#196448,#3199) ;
#2497=LINE('',#196451,#3200) ;
#2498=LINE('',#196453,#3201) ;
#2499=LINE('',#196454,#3202) ;
#2500=LINE('',#196468,#3203) ;
#2501=LINE('',#196471,#3204) ;
#2502=LINE('',#196472,#3205) ;
#2503=LINE('',#196476,#3206) ;
#2504=LINE('',#196484,#3207) ;
#2505=LINE('',#196494,#3208) ;
#2506=LINE('',#196502,#3209) ;
#2507=LINE('',#196510,#3210) ;
#2508=LINE('',#196518,#3211) ;
#2509=LINE('',#196526,#3212) ;
#2510=LINE('',#196534,#3213) ;
#2511=LINE('',#196542,#3214) ;
#2512=LINE('',#196550,#3215) ;
#2513=LINE('',#196561,#3216) ;
#2514=LINE('',#196564,#3217) ;
#2515=LINE('',#196568,#3218) ;
#2516=LINE('',#196571,#3219) ;
#2517=LINE('',#196572,#3220) ;
#2518=LINE('',#196576,#3221) ;
#2519=LINE('',#196580,#3222) ;
#2520=LINE('',#196584,#3223) ;
#2521=LINE('',#196587,#3224) ;
#2522=LINE('',#196588,#3225) ;
#2523=LINE('',#196594,#3226) ;
#2524=LINE('',#196597,#3227) ;
#2525=LINE('',#196600,#3228) ;
#2526=LINE('',#196604,#3229) ;
#2527=LINE('',#196607,#3230) ;
#2528=LINE('',#196608,#3231) ;
#2529=LINE('',#196612,#3232) ;
#2530=LINE('',#196616,#3233) ;
#2531=LINE('',#196620,#3234) ;
#2532=LINE('',#196623,#3235) ;
#2533=LINE('',#196624,#3236) ;
#2534=LINE('',#196629,#3237) ;
#2535=LINE('',#196632,#3238) ;
#2536=LINE('',#196636,#3239) ;
#2537=LINE('',#196639,#3240) ;
#2538=LINE('',#196640,#3241) ;
#2539=LINE('',#196644,#3242) ;
#2540=LINE('',#196648,#3243) ;
#2541=LINE('',#196652,#3244) ;
#2542=LINE('',#196655,#3245) ;
#2543=LINE('',#196656,#3246) ;
#2544=LINE('',#196661,#3247) ;
#2545=LINE('',#196664,#3248) ;
#2546=LINE('',#196668,#3249) ;
#2547=LINE('',#196671,#3250) ;
#2548=LINE('',#196672,#3251) ;
#2549=LINE('',#196676,#3252) ;
#2550=LINE('',#196680,#3253) ;
#2551=LINE('',#196684,#3254) ;
#2552=LINE('',#196687,#3255) ;
#2553=LINE('',#196688,#3256) ;
#2554=LINE('',#196693,#3257) ;
#2555=LINE('',#196696,#3258) ;
#2556=LINE('',#196700,#3259) ;
#2557=LINE('',#196703,#3260) ;
#2558=LINE('',#196704,#3261) ;
#2559=LINE('',#196708,#3262) ;
#2560=LINE('',#196712,#3263) ;
#2561=LINE('',#196716,#3264) ;
#2562=LINE('',#196719,#3265) ;
#2563=LINE('',#196720,#3266) ;
#2564=LINE('',#196725,#3267) ;
#2565=LINE('',#196731,#3268) ;
#2786=VECTOR('',#10387,10.) ;
#2787=VECTOR('',#10388,10.) ;
#2788=VECTOR('',#10389,10.) ;
#2789=VECTOR('',#10390,10.) ;
#2790=VECTOR('',#10393,10.) ;
#2791=VECTOR('',#10398,10.) ;
#2792=VECTOR('',#10399,10.) ;
#2793=VECTOR('',#10400,10.) ;
#2794=VECTOR('',#10403,10.) ;
#2795=VECTOR('',#10404,10.) ;
#2796=VECTOR('',#10405,10.) ;
#2797=VECTOR('',#10408,10.) ;
#2798=VECTOR('',#10413,10.) ;
#2799=VECTOR('',#10414,10.) ;
#2800=VECTOR('',#10415,10.) ;
#2801=VECTOR('',#10418,10.) ;
#2802=VECTOR('',#10419,10.) ;
#2803=VECTOR('',#10420,10.) ;
#2804=VECTOR('',#10423,10.) ;
#2805=VECTOR('',#10428,10.) ;
#2806=VECTOR('',#10429,10.) ;
#2807=VECTOR('',#10430,10.) ;
#2808=VECTOR('',#10433,10.) ;
#2809=VECTOR('',#10434,10.) ;
#2810=VECTOR('',#10435,10.) ;
#2811=VECTOR('',#10438,10.) ;
#2812=VECTOR('',#10443,10.) ;
#2813=VECTOR('',#10444,10.) ;
#2814=VECTOR('',#10445,10.) ;
#2815=VECTOR('',#10448,10.) ;
#2816=VECTOR('',#10449,10.) ;
#2817=VECTOR('',#10450,10.) ;
#2818=VECTOR('',#10453,10.) ;
#2819=VECTOR('',#10458,10.) ;
#2820=VECTOR('',#10459,10.) ;
#2821=VECTOR('',#10460,10.) ;
#2822=VECTOR('',#10463,10.) ;
#2823=VECTOR('',#10464,10.) ;
#2824=VECTOR('',#10465,10.) ;
#2825=VECTOR('',#10468,10.) ;
#2826=VECTOR('',#10473,10.) ;
#2827=VECTOR('',#10474,10.) ;
#2828=VECTOR('',#10475,10.) ;
#2829=VECTOR('',#10478,10.) ;
#2830=VECTOR('',#10479,10.) ;
#2831=VECTOR('',#10480,10.) ;
#2832=VECTOR('',#10483,10.) ;
#2833=VECTOR('',#10488,10.) ;
#2834=VECTOR('',#10489,10.) ;
#2835=VECTOR('',#10490,10.) ;
#2836=VECTOR('',#10493,10.) ;
#2837=VECTOR('',#10494,10.) ;
#2838=VECTOR('',#10495,10.) ;
#2839=VECTOR('',#10498,10.) ;
#2840=VECTOR('',#10503,10.) ;
#2841=VECTOR('',#10504,10.) ;
#2842=VECTOR('',#10505,10.) ;
#2843=VECTOR('',#10508,10.) ;
#2844=VECTOR('',#10509,10.) ;
#2845=VECTOR('',#10510,10.) ;
#2846=VECTOR('',#10513,10.) ;
#2847=VECTOR('',#10518,10.) ;
#2848=VECTOR('',#10519,10.) ;
#2849=VECTOR('',#10520,10.) ;
#2850=VECTOR('',#10523,10.) ;
#2851=VECTOR('',#10524,10.) ;
#2852=VECTOR('',#10525,10.) ;
#2853=VECTOR('',#10528,10.) ;
#2854=VECTOR('',#10533,10.) ;
#2855=VECTOR('',#10534,10.) ;
#2856=VECTOR('',#10535,10.) ;
#2857=VECTOR('',#10538,10.) ;
#2858=VECTOR('',#10539,10.) ;
#2859=VECTOR('',#10540,10.) ;
#2860=VECTOR('',#10543,10.) ;
#2861=VECTOR('',#10548,10.) ;
#2862=VECTOR('',#10549,10.) ;
#2863=VECTOR('',#10550,10.) ;
#2864=VECTOR('',#10553,10.) ;
#2865=VECTOR('',#10554,10.) ;
#2866=VECTOR('',#10555,10.) ;
#2867=VECTOR('',#10558,10.) ;
#2868=VECTOR('',#10563,10.) ;
#2869=VECTOR('',#10564,10.) ;
#2870=VECTOR('',#10565,10.) ;
#2871=VECTOR('',#10568,10.) ;
#2872=VECTOR('',#10569,10.) ;
#2873=VECTOR('',#10570,10.) ;
#2874=VECTOR('',#10573,10.) ;
#2875=VECTOR('',#10578,10.) ;
#2876=VECTOR('',#10579,10.) ;
#2877=VECTOR('',#10580,10.) ;
#2878=VECTOR('',#10583,10.) ;
#2879=VECTOR('',#10584,10.) ;
#2880=VECTOR('',#10585,10.) ;
#2881=VECTOR('',#10588,10.) ;
#2882=VECTOR('',#10593,10.) ;
#2883=VECTOR('',#10594,10.) ;
#2884=VECTOR('',#10595,10.) ;
#2885=VECTOR('',#10598,10.) ;
#2886=VECTOR('',#10599,10.) ;
#2887=VECTOR('',#10600,10.) ;
#2888=VECTOR('',#10603,10.) ;
#2889=VECTOR('',#10608,10.) ;
#2890=VECTOR('',#10609,10.) ;
#2891=VECTOR('',#10610,10.) ;
#2892=VECTOR('',#10613,10.) ;
#2893=VECTOR('',#10614,10.) ;
#2894=VECTOR('',#10615,10.) ;
#2895=VECTOR('',#10618,10.) ;
#2896=VECTOR('',#10623,10.) ;
#2897=VECTOR('',#10624,10.) ;
#2898=VECTOR('',#10625,10.) ;
#2899=VECTOR('',#10628,10.) ;
#2900=VECTOR('',#10629,10.) ;
#2901=VECTOR('',#10630,10.) ;
#2902=VECTOR('',#10633,10.) ;
#2903=VECTOR('',#10638,10.) ;
#2904=VECTOR('',#10639,10.) ;
#2905=VECTOR('',#10640,10.) ;
#2906=VECTOR('',#10643,10.) ;
#2907=VECTOR('',#10644,10.) ;
#2908=VECTOR('',#10645,10.) ;
#2909=VECTOR('',#10648,10.) ;
#2910=VECTOR('',#10653,10.) ;
#2911=VECTOR('',#10654,10.) ;
#2912=VECTOR('',#10655,10.) ;
#2913=VECTOR('',#10658,10.) ;
#2914=VECTOR('',#10659,10.) ;
#2915=VECTOR('',#10660,10.) ;
#2916=VECTOR('',#10663,10.) ;
#2917=VECTOR('',#10668,10.) ;
#2918=VECTOR('',#10669,10.) ;
#2919=VECTOR('',#10670,10.) ;
#2920=VECTOR('',#10673,10.) ;
#2921=VECTOR('',#10674,10.) ;
#2922=VECTOR('',#10675,10.) ;
#2923=VECTOR('',#10678,10.) ;
#2924=VECTOR('',#10683,10.) ;
#2925=VECTOR('',#10684,10.) ;
#2926=VECTOR('',#10685,10.) ;
#2927=VECTOR('',#10688,10.) ;
#2928=VECTOR('',#10689,10.) ;
#2929=VECTOR('',#10690,10.) ;
#2930=VECTOR('',#10693,10.) ;
#2931=VECTOR('',#10698,10.) ;
#2932=VECTOR('',#10699,10.) ;
#2933=VECTOR('',#10700,10.) ;
#2934=VECTOR('',#10703,10.) ;
#2935=VECTOR('',#10704,10.) ;
#2936=VECTOR('',#10705,10.) ;
#2937=VECTOR('',#10708,10.) ;
#2938=VECTOR('',#10713,10.) ;
#2939=VECTOR('',#10714,10.) ;
#2940=VECTOR('',#10715,10.) ;
#2941=VECTOR('',#10718,10.) ;
#2942=VECTOR('',#10719,10.) ;
#2943=VECTOR('',#10720,10.) ;
#2944=VECTOR('',#10723,10.) ;
#2945=VECTOR('',#10728,10.) ;
#2946=VECTOR('',#10729,10.) ;
#2947=VECTOR('',#10730,10.) ;
#2948=VECTOR('',#10733,10.) ;
#2949=VECTOR('',#10734,10.) ;
#2950=VECTOR('',#10735,10.) ;
#2951=VECTOR('',#10738,10.) ;
#2952=VECTOR('',#10743,10.) ;
#2953=VECTOR('',#10744,10.) ;
#2954=VECTOR('',#10745,10.) ;
#2955=VECTOR('',#10748,10.) ;
#2956=VECTOR('',#10749,10.) ;
#2957=VECTOR('',#10750,10.) ;
#2958=VECTOR('',#10753,10.) ;
#2959=VECTOR('',#10758,10.) ;
#2960=VECTOR('',#10759,10.) ;
#2961=VECTOR('',#10760,10.) ;
#2962=VECTOR('',#10763,10.) ;
#2963=VECTOR('',#10764,10.) ;
#2964=VECTOR('',#10765,10.) ;
#2965=VECTOR('',#10768,10.) ;
#2966=VECTOR('',#10773,10.) ;
#2967=VECTOR('',#10774,10.) ;
#2968=VECTOR('',#10775,10.) ;
#2969=VECTOR('',#10778,10.) ;
#2970=VECTOR('',#10779,10.) ;
#2971=VECTOR('',#10780,10.) ;
#2972=VECTOR('',#10783,10.) ;
#2973=VECTOR('',#10788,10.) ;
#2974=VECTOR('',#10789,10.) ;
#2975=VECTOR('',#10790,10.) ;
#2976=VECTOR('',#10793,10.) ;
#2977=VECTOR('',#10794,10.) ;
#2978=VECTOR('',#10795,10.) ;
#2979=VECTOR('',#10798,10.) ;
#2980=VECTOR('',#10803,10.) ;
#2981=VECTOR('',#10804,10.) ;
#2982=VECTOR('',#10805,10.) ;
#2983=VECTOR('',#10808,10.) ;
#2984=VECTOR('',#10809,10.) ;
#2985=VECTOR('',#10810,10.) ;
#2986=VECTOR('',#10813,10.) ;
#2987=VECTOR('',#10818,10.) ;
#2988=VECTOR('',#10819,10.) ;
#2989=VECTOR('',#10820,10.) ;
#2990=VECTOR('',#10823,10.) ;
#2991=VECTOR('',#10824,10.) ;
#2992=VECTOR('',#10825,10.) ;
#2993=VECTOR('',#10828,10.) ;
#2994=VECTOR('',#10833,10.) ;
#2995=VECTOR('',#10834,10.) ;
#2996=VECTOR('',#10835,10.) ;
#2997=VECTOR('',#10838,10.) ;
#2998=VECTOR('',#10839,10.) ;
#2999=VECTOR('',#10840,10.) ;
#3000=VECTOR('',#10843,10.) ;
#3001=VECTOR('',#10848,10.) ;
#3002=VECTOR('',#10849,10.) ;
#3003=VECTOR('',#10850,10.) ;
#3004=VECTOR('',#10853,10.) ;
#3005=VECTOR('',#10854,10.) ;
#3006=VECTOR('',#10855,10.) ;
#3007=VECTOR('',#10858,10.) ;
#3008=VECTOR('',#10863,10.) ;
#3009=VECTOR('',#10864,10.) ;
#3010=VECTOR('',#10865,10.) ;
#3011=VECTOR('',#10868,10.) ;
#3012=VECTOR('',#10869,10.) ;
#3013=VECTOR('',#10870,10.) ;
#3014=VECTOR('',#10873,10.) ;
#3015=VECTOR('',#10878,10.) ;
#3016=VECTOR('',#10879,10.) ;
#3017=VECTOR('',#10880,10.) ;
#3018=VECTOR('',#10883,10.) ;
#3019=VECTOR('',#10884,10.) ;
#3020=VECTOR('',#10885,10.) ;
#3021=VECTOR('',#10888,10.) ;
#3022=VECTOR('',#10893,10.) ;
#3023=VECTOR('',#10894,10.) ;
#3024=VECTOR('',#10895,10.) ;
#3025=VECTOR('',#10898,10.) ;
#3026=VECTOR('',#10899,10.) ;
#3027=VECTOR('',#10900,10.) ;
#3028=VECTOR('',#10903,10.) ;
#3029=VECTOR('',#10908,10.) ;
#3030=VECTOR('',#10909,10.) ;
#3031=VECTOR('',#10910,10.) ;
#3032=VECTOR('',#10913,10.) ;
#3033=VECTOR('',#10914,10.) ;
#3034=VECTOR('',#10915,10.) ;
#3035=VECTOR('',#10918,10.) ;
#3036=VECTOR('',#10923,10.) ;
#3037=VECTOR('',#10924,10.) ;
#3038=VECTOR('',#10925,10.) ;
#3039=VECTOR('',#10928,10.) ;
#3040=VECTOR('',#10929,10.) ;
#3041=VECTOR('',#10930,10.) ;
#3042=VECTOR('',#10933,10.) ;
#3043=VECTOR('',#10938,10.) ;
#3044=VECTOR('',#10939,10.) ;
#3045=VECTOR('',#10940,10.) ;
#3046=VECTOR('',#10943,10.) ;
#3047=VECTOR('',#10944,10.) ;
#3048=VECTOR('',#10945,10.) ;
#3049=VECTOR('',#10948,10.) ;
#3050=VECTOR('',#10953,10.) ;
#3051=VECTOR('',#10954,10.) ;
#3052=VECTOR('',#10955,10.) ;
#3053=VECTOR('',#10958,10.) ;
#3054=VECTOR('',#10959,10.) ;
#3055=VECTOR('',#10960,10.) ;
#3056=VECTOR('',#10963,10.) ;
#3057=VECTOR('',#10968,10.) ;
#3058=VECTOR('',#10969,10.) ;
#3059=VECTOR('',#10970,10.) ;
#3060=VECTOR('',#10973,10.) ;
#3061=VECTOR('',#10974,10.) ;
#3062=VECTOR('',#10975,10.) ;
#3063=VECTOR('',#10978,10.) ;
#3064=VECTOR('',#10983,10.) ;
#3065=VECTOR('',#10984,10.) ;
#3066=VECTOR('',#10985,10.) ;
#3067=VECTOR('',#10988,10.) ;
#3068=VECTOR('',#10989,10.) ;
#3069=VECTOR('',#10990,10.) ;
#3070=VECTOR('',#10993,10.) ;
#3071=VECTOR('',#10998,10.) ;
#3072=VECTOR('',#10999,10.) ;
#3073=VECTOR('',#11000,10.) ;
#3074=VECTOR('',#11003,10.) ;
#3075=VECTOR('',#11004,10.) ;
#3076=VECTOR('',#11005,10.) ;
#3077=VECTOR('',#11008,10.) ;
#3078=VECTOR('',#11013,10.) ;
#3079=VECTOR('',#11014,10.) ;
#3080=VECTOR('',#11015,10.) ;
#3081=VECTOR('',#11018,10.) ;
#3082=VECTOR('',#11019,10.) ;
#3083=VECTOR('',#11020,10.) ;
#3084=VECTOR('',#11023,10.) ;
#3085=VECTOR('',#11028,10.) ;
#3086=VECTOR('',#11029,10.) ;
#3087=VECTOR('',#11030,10.) ;
#3088=VECTOR('',#11033,10.) ;
#3089=VECTOR('',#11034,10.) ;
#3090=VECTOR('',#11035,10.) ;
#3091=VECTOR('',#11038,10.) ;
#3092=VECTOR('',#11043,10.) ;
#3093=VECTOR('',#11044,10.) ;
#3094=VECTOR('',#11045,10.) ;
#3095=VECTOR('',#11048,10.) ;
#3096=VECTOR('',#11049,10.) ;
#3097=VECTOR('',#11050,10.) ;
#3098=VECTOR('',#11053,10.) ;
#3099=VECTOR('',#11058,10.) ;
#3100=VECTOR('',#11059,10.) ;
#3101=VECTOR('',#11060,10.) ;
#3102=VECTOR('',#11063,10.) ;
#3103=VECTOR('',#11064,10.) ;
#3104=VECTOR('',#11065,10.) ;
#3105=VECTOR('',#11068,10.) ;
#3106=VECTOR('',#11073,10.) ;
#3107=VECTOR('',#11074,10.) ;
#3108=VECTOR('',#11075,10.) ;
#3109=VECTOR('',#11078,10.) ;
#3110=VECTOR('',#11079,10.) ;
#3111=VECTOR('',#11080,10.) ;
#3112=VECTOR('',#11083,10.) ;
#3113=VECTOR('',#11088,10.) ;
#3114=VECTOR('',#11089,10.) ;
#3115=VECTOR('',#11090,10.) ;
#3116=VECTOR('',#11093,10.) ;
#3117=VECTOR('',#11094,10.) ;
#3118=VECTOR('',#11095,10.) ;
#3119=VECTOR('',#11098,10.) ;
#3120=VECTOR('',#11103,10.) ;
#3121=VECTOR('',#11104,10.) ;
#3122=VECTOR('',#11105,10.) ;
#3123=VECTOR('',#11108,10.) ;
#3124=VECTOR('',#11109,10.) ;
#3125=VECTOR('',#11110,10.) ;
#3126=VECTOR('',#11113,10.) ;
#3127=VECTOR('',#11118,10.) ;
#3128=VECTOR('',#11119,10.) ;
#3129=VECTOR('',#11120,10.) ;
#3130=VECTOR('',#11123,10.) ;
#3131=VECTOR('',#11124,10.) ;
#3132=VECTOR('',#11125,10.) ;
#3133=VECTOR('',#11128,10.) ;
#3134=VECTOR('',#11133,10.) ;
#3135=VECTOR('',#11134,10.) ;
#3136=VECTOR('',#11135,10.) ;
#3137=VECTOR('',#11138,10.) ;
#3138=VECTOR('',#11139,10.) ;
#3139=VECTOR('',#11140,10.) ;
#3140=VECTOR('',#11143,10.) ;
#3141=VECTOR('',#11148,10.) ;
#3142=VECTOR('',#11149,10.) ;
#3143=VECTOR('',#11150,10.) ;
#3144=VECTOR('',#11153,10.) ;
#3145=VECTOR('',#11154,10.) ;
#3146=VECTOR('',#11155,10.) ;
#3147=VECTOR('',#11158,10.) ;
#3148=VECTOR('',#11163,10.) ;
#3149=VECTOR('',#11164,10.) ;
#3150=VECTOR('',#11165,10.) ;
#3151=VECTOR('',#11168,10.) ;
#3152=VECTOR('',#11169,10.) ;
#3153=VECTOR('',#11170,10.) ;
#3154=VECTOR('',#11173,10.) ;
#3155=VECTOR('',#11178,10.) ;
#3156=VECTOR('',#11179,10.) ;
#3157=VECTOR('',#11180,10.) ;
#3158=VECTOR('',#11183,10.) ;
#3159=VECTOR('',#11184,10.) ;
#3160=VECTOR('',#11185,10.) ;
#3161=VECTOR('',#11188,10.) ;
#3162=VECTOR('',#11193,10.) ;
#3163=VECTOR('',#11194,10.) ;
#3164=VECTOR('',#11195,10.) ;
#3165=VECTOR('',#11198,10.) ;
#3166=VECTOR('',#11199,10.) ;
#3167=VECTOR('',#11200,10.) ;
#3168=VECTOR('',#11203,10.) ;
#3169=VECTOR('',#11208,10.) ;
#3170=VECTOR('',#11209,10.) ;
#3171=VECTOR('',#11210,10.) ;
#3172=VECTOR('',#11213,10.) ;
#3173=VECTOR('',#11214,10.) ;
#3174=VECTOR('',#11215,10.) ;
#3175=VECTOR('',#11218,10.) ;
#3176=VECTOR('',#11223,10.) ;
#3177=VECTOR('',#11224,10.) ;
#3178=VECTOR('',#11225,10.) ;
#3179=VECTOR('',#11228,10.) ;
#3180=VECTOR('',#11229,10.) ;
#3181=VECTOR('',#11230,10.) ;
#3182=VECTOR('',#11233,10.) ;
#3183=VECTOR('',#11238,10.) ;
#3184=VECTOR('',#11239,10.) ;
#3185=VECTOR('',#11240,10.) ;
#3186=VECTOR('',#11243,10.) ;
#3187=VECTOR('',#11244,10.) ;
#3188=VECTOR('',#11245,10.) ;
#3189=VECTOR('',#11248,10.) ;
#3190=VECTOR('',#11253,10.) ;
#3191=VECTOR('',#11254,10.) ;
#3192=VECTOR('',#11255,10.) ;
#3193=VECTOR('',#11258,10.) ;
#3194=VECTOR('',#11259,10.) ;
#3195=VECTOR('',#11260,10.) ;
#3196=VECTOR('',#11263,10.) ;
#3197=VECTOR('',#11268,10.) ;
#3198=VECTOR('',#11269,10.) ;
#3199=VECTOR('',#11270,10.) ;
#3200=VECTOR('',#11273,10.) ;
#3201=VECTOR('',#11274,10.) ;
#3202=VECTOR('',#11275,10.) ;
#3203=VECTOR('',#11278,10.) ;
#3204=VECTOR('',#11283,10.) ;
#3205=VECTOR('',#11284,10.) ;
#3206=VECTOR('',#11287,10.) ;
#3207=VECTOR('',#11294,10.) ;
#3208=VECTOR('',#11303,10.) ;
#3209=VECTOR('',#11310,10.) ;
#3210=VECTOR('',#11317,10.) ;
#3211=VECTOR('',#11324,10.) ;
#3212=VECTOR('',#11331,10.) ;
#3213=VECTOR('',#11338,10.) ;
#3214=VECTOR('',#11345,10.) ;
#3215=VECTOR('',#11352,10.) ;
#3216=VECTOR('',#11365,10.) ;
#3217=VECTOR('',#11368,10.) ;
#3218=VECTOR('',#11373,10.) ;
#3219=VECTOR('',#11376,10.) ;
#3220=VECTOR('',#11377,10.) ;
#3221=VECTOR('',#11382,10.) ;
#3222=VECTOR('',#11387,10.) ;
#3223=VECTOR('',#11392,10.) ;
#3224=VECTOR('',#11395,10.) ;
#3225=VECTOR('',#11396,10.) ;
#3226=VECTOR('',#11405,8.00000000000007) ;
#3227=VECTOR('',#11408,10.) ;
#3228=VECTOR('',#11411,10.) ;
#3229=VECTOR('',#11416,10.) ;
#3230=VECTOR('',#11419,10.) ;
#3231=VECTOR('',#11420,10.) ;
#3232=VECTOR('',#11425,10.) ;
#3233=VECTOR('',#11430,10.) ;
#3234=VECTOR('',#11435,10.) ;
#3235=VECTOR('',#11438,10.) ;
#3236=VECTOR('',#11439,10.) ;
#3237=VECTOR('',#11446,10.) ;
#3238=VECTOR('',#11449,10.) ;
#3239=VECTOR('',#11454,10.) ;
#3240=VECTOR('',#11457,10.) ;
#3241=VECTOR('',#11458,10.) ;
#3242=VECTOR('',#11463,10.) ;
#3243=VECTOR('',#11468,10.) ;
#3244=VECTOR('',#11473,10.) ;
#3245=VECTOR('',#11476,10.) ;
#3246=VECTOR('',#11477,10.) ;
#3247=VECTOR('',#11484,10.) ;
#3248=VECTOR('',#11487,10.) ;
#3249=VECTOR('',#11492,10.) ;
#3250=VECTOR('',#11495,10.) ;
#3251=VECTOR('',#11496,10.) ;
#3252=VECTOR('',#11501,10.) ;
#3253=VECTOR('',#11506,10.) ;
#3254=VECTOR('',#11511,10.) ;
#3255=VECTOR('',#11514,10.) ;
#3256=VECTOR('',#11515,10.) ;
#3257=VECTOR('',#11522,10.) ;
#3258=VECTOR('',#11525,10.) ;
#3259=VECTOR('',#11530,10.) ;
#3260=VECTOR('',#11533,10.) ;
#3261=VECTOR('',#11534,10.) ;
#3262=VECTOR('',#11539,10.) ;
#3263=VECTOR('',#11544,10.) ;
#3264=VECTOR('',#11549,10.) ;
#3265=VECTOR('',#11552,10.) ;
#3266=VECTOR('',#11553,10.) ;
#3267=VECTOR('',#11560,83.314636823702) ;
#3268=VECTOR('',#11567,81.1146368237021) ;
#3846=VERTEX_POINT('',#194854) ;
#3847=VERTEX_POINT('',#194855) ;
#3848=VERTEX_POINT('',#194857) ;
#3849=VERTEX_POINT('',#194859) ;
#3850=VERTEX_POINT('',#194872) ;
#3851=VERTEX_POINT('',#194874) ;
#3852=VERTEX_POINT('',#194878) ;
#3853=VERTEX_POINT('',#194880) ;
#3854=VERTEX_POINT('',#194884) ;
#3855=VERTEX_POINT('',#194886) ;
#3856=VERTEX_POINT('',#194899) ;
#3857=VERTEX_POINT('',#194901) ;
#3858=VERTEX_POINT('',#194905) ;
#3859=VERTEX_POINT('',#194907) ;
#3860=VERTEX_POINT('',#194911) ;
#3861=VERTEX_POINT('',#194913) ;
#3862=VERTEX_POINT('',#194926) ;
#3863=VERTEX_POINT('',#194928) ;
#3864=VERTEX_POINT('',#194932) ;
#3865=VERTEX_POINT('',#194934) ;
#3866=VERTEX_POINT('',#194938) ;
#3867=VERTEX_POINT('',#194940) ;
#3868=VERTEX_POINT('',#194953) ;
#3869=VERTEX_POINT('',#194955) ;
#3870=VERTEX_POINT('',#194959) ;
#3871=VERTEX_POINT('',#194961) ;
#3872=VERTEX_POINT('',#194965) ;
#3873=VERTEX_POINT('',#194967) ;
#3874=VERTEX_POINT('',#194980) ;
#3875=VERTEX_POINT('',#194982) ;
#3876=VERTEX_POINT('',#194986) ;
#3877=VERTEX_POINT('',#194988) ;
#3878=VERTEX_POINT('',#194992) ;
#3879=VERTEX_POINT('',#194994) ;
#3880=VERTEX_POINT('',#195007) ;
#3881=VERTEX_POINT('',#195009) ;
#3882=VERTEX_POINT('',#195013) ;
#3883=VERTEX_POINT('',#195015) ;
#3884=VERTEX_POINT('',#195019) ;
#3885=VERTEX_POINT('',#195021) ;
#3886=VERTEX_POINT('',#195034) ;
#3887=VERTEX_POINT('',#195036) ;
#3888=VERTEX_POINT('',#195040) ;
#3889=VERTEX_POINT('',#195042) ;
#3890=VERTEX_POINT('',#195046) ;
#3891=VERTEX_POINT('',#195048) ;
#3892=VERTEX_POINT('',#195061) ;
#3893=VERTEX_POINT('',#195063) ;
#3894=VERTEX_POINT('',#195067) ;
#3895=VERTEX_POINT('',#195069) ;
#3896=VERTEX_POINT('',#195073) ;
#3897=VERTEX_POINT('',#195075) ;
#3898=VERTEX_POINT('',#195088) ;
#3899=VERTEX_POINT('',#195090) ;
#3900=VERTEX_POINT('',#195094) ;
#3901=VERTEX_POINT('',#195096) ;
#3902=VERTEX_POINT('',#195100) ;
#3903=VERTEX_POINT('',#195102) ;
#3904=VERTEX_POINT('',#195115) ;
#3905=VERTEX_POINT('',#195117) ;
#3906=VERTEX_POINT('',#195121) ;
#3907=VERTEX_POINT('',#195123) ;
#3908=VERTEX_POINT('',#195127) ;
#3909=VERTEX_POINT('',#195129) ;
#3910=VERTEX_POINT('',#195142) ;
#3911=VERTEX_POINT('',#195144) ;
#3912=VERTEX_POINT('',#195148) ;
#3913=VERTEX_POINT('',#195150) ;
#3914=VERTEX_POINT('',#195154) ;
#3915=VERTEX_POINT('',#195156) ;
#3916=VERTEX_POINT('',#195169) ;
#3917=VERTEX_POINT('',#195171) ;
#3918=VERTEX_POINT('',#195175) ;
#3919=VERTEX_POINT('',#195177) ;
#3920=VERTEX_POINT('',#195181) ;
#3921=VERTEX_POINT('',#195183) ;
#3922=VERTEX_POINT('',#195196) ;
#3923=VERTEX_POINT('',#195198) ;
#3924=VERTEX_POINT('',#195202) ;
#3925=VERTEX_POINT('',#195204) ;
#3926=VERTEX_POINT('',#195208) ;
#3927=VERTEX_POINT('',#195210) ;
#3928=VERTEX_POINT('',#195223) ;
#3929=VERTEX_POINT('',#195225) ;
#3930=VERTEX_POINT('',#195229) ;
#3931=VERTEX_POINT('',#195231) ;
#3932=VERTEX_POINT('',#195235) ;
#3933=VERTEX_POINT('',#195237) ;
#3934=VERTEX_POINT('',#195250) ;
#3935=VERTEX_POINT('',#195252) ;
#3936=VERTEX_POINT('',#195256) ;
#3937=VERTEX_POINT('',#195258) ;
#3938=VERTEX_POINT('',#195262) ;
#3939=VERTEX_POINT('',#195264) ;
#3940=VERTEX_POINT('',#195277) ;
#3941=VERTEX_POINT('',#195279) ;
#3942=VERTEX_POINT('',#195283) ;
#3943=VERTEX_POINT('',#195285) ;
#3944=VERTEX_POINT('',#195289) ;
#3945=VERTEX_POINT('',#195291) ;
#3946=VERTEX_POINT('',#195304) ;
#3947=VERTEX_POINT('',#195306) ;
#3948=VERTEX_POINT('',#195310) ;
#3949=VERTEX_POINT('',#195312) ;
#3950=VERTEX_POINT('',#195316) ;
#3951=VERTEX_POINT('',#195318) ;
#3952=VERTEX_POINT('',#195331) ;
#3953=VERTEX_POINT('',#195333) ;
#3954=VERTEX_POINT('',#195337) ;
#3955=VERTEX_POINT('',#195339) ;
#3956=VERTEX_POINT('',#195343) ;
#3957=VERTEX_POINT('',#195345) ;
#3958=VERTEX_POINT('',#195358) ;
#3959=VERTEX_POINT('',#195360) ;
#3960=VERTEX_POINT('',#195364) ;
#3961=VERTEX_POINT('',#195366) ;
#3962=VERTEX_POINT('',#195370) ;
#3963=VERTEX_POINT('',#195372) ;
#3964=VERTEX_POINT('',#195385) ;
#3965=VERTEX_POINT('',#195387) ;
#3966=VERTEX_POINT('',#195391) ;
#3967=VERTEX_POINT('',#195393) ;
#3968=VERTEX_POINT('',#195397) ;
#3969=VERTEX_POINT('',#195399) ;
#3970=VERTEX_POINT('',#195412) ;
#3971=VERTEX_POINT('',#195414) ;
#3972=VERTEX_POINT('',#195418) ;
#3973=VERTEX_POINT('',#195420) ;
#3974=VERTEX_POINT('',#195424) ;
#3975=VERTEX_POINT('',#195426) ;
#3976=VERTEX_POINT('',#195439) ;
#3977=VERTEX_POINT('',#195441) ;
#3978=VERTEX_POINT('',#195445) ;
#3979=VERTEX_POINT('',#195447) ;
#3980=VERTEX_POINT('',#195451) ;
#3981=VERTEX_POINT('',#195453) ;
#3982=VERTEX_POINT('',#195466) ;
#3983=VERTEX_POINT('',#195468) ;
#3984=VERTEX_POINT('',#195472) ;
#3985=VERTEX_POINT('',#195474) ;
#3986=VERTEX_POINT('',#195478) ;
#3987=VERTEX_POINT('',#195480) ;
#3988=VERTEX_POINT('',#195493) ;
#3989=VERTEX_POINT('',#195495) ;
#3990=VERTEX_POINT('',#195499) ;
#3991=VERTEX_POINT('',#195501) ;
#3992=VERTEX_POINT('',#195505) ;
#3993=VERTEX_POINT('',#195507) ;
#3994=VERTEX_POINT('',#195520) ;
#3995=VERTEX_POINT('',#195522) ;
#3996=VERTEX_POINT('',#195526) ;
#3997=VERTEX_POINT('',#195528) ;
#3998=VERTEX_POINT('',#195532) ;
#3999=VERTEX_POINT('',#195534) ;
#4000=VERTEX_POINT('',#195547) ;
#4001=VERTEX_POINT('',#195549) ;
#4002=VERTEX_POINT('',#195553) ;
#4003=VERTEX_POINT('',#195555) ;
#4004=VERTEX_POINT('',#195559) ;
#4005=VERTEX_POINT('',#195561) ;
#4006=VERTEX_POINT('',#195574) ;
#4007=VERTEX_POINT('',#195576) ;
#4008=VERTEX_POINT('',#195580) ;
#4009=VERTEX_POINT('',#195582) ;
#4010=VERTEX_POINT('',#195586) ;
#4011=VERTEX_POINT('',#195588) ;
#4012=VERTEX_POINT('',#195601) ;
#4013=VERTEX_POINT('',#195603) ;
#4014=VERTEX_POINT('',#195607) ;
#4015=VERTEX_POINT('',#195609) ;
#4016=VERTEX_POINT('',#195613) ;
#4017=VERTEX_POINT('',#195615) ;
#4018=VERTEX_POINT('',#195628) ;
#4019=VERTEX_POINT('',#195630) ;
#4020=VERTEX_POINT('',#195634) ;
#4021=VERTEX_POINT('',#195636) ;
#4022=VERTEX_POINT('',#195640) ;
#4023=VERTEX_POINT('',#195642) ;
#4024=VERTEX_POINT('',#195655) ;
#4025=VERTEX_POINT('',#195657) ;
#4026=VERTEX_POINT('',#195661) ;
#4027=VERTEX_POINT('',#195663) ;
#4028=VERTEX_POINT('',#195667) ;
#4029=VERTEX_POINT('',#195669) ;
#4030=VERTEX_POINT('',#195682) ;
#4031=VERTEX_POINT('',#195684) ;
#4032=VERTEX_POINT('',#195688) ;
#4033=VERTEX_POINT('',#195690) ;
#4034=VERTEX_POINT('',#195694) ;
#4035=VERTEX_POINT('',#195696) ;
#4036=VERTEX_POINT('',#195709) ;
#4037=VERTEX_POINT('',#195711) ;
#4038=VERTEX_POINT('',#195715) ;
#4039=VERTEX_POINT('',#195717) ;
#4040=VERTEX_POINT('',#195721) ;
#4041=VERTEX_POINT('',#195723) ;
#4042=VERTEX_POINT('',#195736) ;
#4043=VERTEX_POINT('',#195738) ;
#4044=VERTEX_POINT('',#195742) ;
#4045=VERTEX_POINT('',#195744) ;
#4046=VERTEX_POINT('',#195748) ;
#4047=VERTEX_POINT('',#195750) ;
#4048=VERTEX_POINT('',#195763) ;
#4049=VERTEX_POINT('',#195765) ;
#4050=VERTEX_POINT('',#195769) ;
#4051=VERTEX_POINT('',#195771) ;
#4052=VERTEX_POINT('',#195775) ;
#4053=VERTEX_POINT('',#195777) ;
#4054=VERTEX_POINT('',#195790) ;
#4055=VERTEX_POINT('',#195792) ;
#4056=VERTEX_POINT('',#195796) ;
#4057=VERTEX_POINT('',#195798) ;
#4058=VERTEX_POINT('',#195802) ;
#4059=VERTEX_POINT('',#195804) ;
#4060=VERTEX_POINT('',#195817) ;
#4061=VERTEX_POINT('',#195819) ;
#4062=VERTEX_POINT('',#195823) ;
#4063=VERTEX_POINT('',#195825) ;
#4064=VERTEX_POINT('',#195829) ;
#4065=VERTEX_POINT('',#195831) ;
#4066=VERTEX_POINT('',#195844) ;
#4067=VERTEX_POINT('',#195846) ;
#4068=VERTEX_POINT('',#195850) ;
#4069=VERTEX_POINT('',#195852) ;
#4070=VERTEX_POINT('',#195856) ;
#4071=VERTEX_POINT('',#195858) ;
#4072=VERTEX_POINT('',#195871) ;
#4073=VERTEX_POINT('',#195873) ;
#4074=VERTEX_POINT('',#195877) ;
#4075=VERTEX_POINT('',#195879) ;
#4076=VERTEX_POINT('',#195883) ;
#4077=VERTEX_POINT('',#195885) ;
#4078=VERTEX_POINT('',#195898) ;
#4079=VERTEX_POINT('',#195900) ;
#4080=VERTEX_POINT('',#195904) ;
#4081=VERTEX_POINT('',#195906) ;
#4082=VERTEX_POINT('',#195910) ;
#4083=VERTEX_POINT('',#195912) ;
#4084=VERTEX_POINT('',#195925) ;
#4085=VERTEX_POINT('',#195927) ;
#4086=VERTEX_POINT('',#195931) ;
#4087=VERTEX_POINT('',#195933) ;
#4088=VERTEX_POINT('',#195937) ;
#4089=VERTEX_POINT('',#195939) ;
#4090=VERTEX_POINT('',#195952) ;
#4091=VERTEX_POINT('',#195954) ;
#4092=VERTEX_POINT('',#195958) ;
#4093=VERTEX_POINT('',#195960) ;
#4094=VERTEX_POINT('',#195964) ;
#4095=VERTEX_POINT('',#195966) ;
#4096=VERTEX_POINT('',#195979) ;
#4097=VERTEX_POINT('',#195981) ;
#4098=VERTEX_POINT('',#195985) ;
#4099=VERTEX_POINT('',#195987) ;
#4100=VERTEX_POINT('',#195991) ;
#4101=VERTEX_POINT('',#195993) ;
#4102=VERTEX_POINT('',#196006) ;
#4103=VERTEX_POINT('',#196008) ;
#4104=VERTEX_POINT('',#196012) ;
#4105=VERTEX_POINT('',#196014) ;
#4106=VERTEX_POINT('',#196018) ;
#4107=VERTEX_POINT('',#196020) ;
#4108=VERTEX_POINT('',#196033) ;
#4109=VERTEX_POINT('',#196035) ;
#4110=VERTEX_POINT('',#196039) ;
#4111=VERTEX_POINT('',#196041) ;
#4112=VERTEX_POINT('',#196045) ;
#4113=VERTEX_POINT('',#196047) ;
#4114=VERTEX_POINT('',#196060) ;
#4115=VERTEX_POINT('',#196062) ;
#4116=VERTEX_POINT('',#196066) ;
#4117=VERTEX_POINT('',#196068) ;
#4118=VERTEX_POINT('',#196072) ;
#4119=VERTEX_POINT('',#196074) ;
#4120=VERTEX_POINT('',#196087) ;
#4121=VERTEX_POINT('',#196089) ;
#4122=VERTEX_POINT('',#196093) ;
#4123=VERTEX_POINT('',#196095) ;
#4124=VERTEX_POINT('',#196099) ;
#4125=VERTEX_POINT('',#196101) ;
#4126=VERTEX_POINT('',#196114) ;
#4127=VERTEX_POINT('',#196116) ;
#4128=VERTEX_POINT('',#196120) ;
#4129=VERTEX_POINT('',#196122) ;
#4130=VERTEX_POINT('',#196126) ;
#4131=VERTEX_POINT('',#196128) ;
#4132=VERTEX_POINT('',#196141) ;
#4133=VERTEX_POINT('',#196143) ;
#4134=VERTEX_POINT('',#196147) ;
#4135=VERTEX_POINT('',#196149) ;
#4136=VERTEX_POINT('',#196153) ;
#4137=VERTEX_POINT('',#196155) ;
#4138=VERTEX_POINT('',#196168) ;
#4139=VERTEX_POINT('',#196170) ;
#4140=VERTEX_POINT('',#196174) ;
#4141=VERTEX_POINT('',#196176) ;
#4142=VERTEX_POINT('',#196180) ;
#4143=VERTEX_POINT('',#196182) ;
#4144=VERTEX_POINT('',#196195) ;
#4145=VERTEX_POINT('',#196197) ;
#4146=VERTEX_POINT('',#196201) ;
#4147=VERTEX_POINT('',#196203) ;
#4148=VERTEX_POINT('',#196207) ;
#4149=VERTEX_POINT('',#196209) ;
#4150=VERTEX_POINT('',#196222) ;
#4151=VERTEX_POINT('',#196224) ;
#4152=VERTEX_POINT('',#196228) ;
#4153=VERTEX_POINT('',#196230) ;
#4154=VERTEX_POINT('',#196234) ;
#4155=VERTEX_POINT('',#196236) ;
#4156=VERTEX_POINT('',#196249) ;
#4157=VERTEX_POINT('',#196251) ;
#4158=VERTEX_POINT('',#196255) ;
#4159=VERTEX_POINT('',#196257) ;
#4160=VERTEX_POINT('',#196261) ;
#4161=VERTEX_POINT('',#196263) ;
#4162=VERTEX_POINT('',#196276) ;
#4163=VERTEX_POINT('',#196278) ;
#4164=VERTEX_POINT('',#196282) ;
#4165=VERTEX_POINT('',#196284) ;
#4166=VERTEX_POINT('',#196288) ;
#4167=VERTEX_POINT('',#196290) ;
#4168=VERTEX_POINT('',#196303) ;
#4169=VERTEX_POINT('',#196305) ;
#4170=VERTEX_POINT('',#196309) ;
#4171=VERTEX_POINT('',#196311) ;
#4172=VERTEX_POINT('',#196315) ;
#4173=VERTEX_POINT('',#196317) ;
#4174=VERTEX_POINT('',#196330) ;
#4175=VERTEX_POINT('',#196332) ;
#4176=VERTEX_POINT('',#196336) ;
#4177=VERTEX_POINT('',#196338) ;
#4178=VERTEX_POINT('',#196342) ;
#4179=VERTEX_POINT('',#196344) ;
#4180=VERTEX_POINT('',#196357) ;
#4181=VERTEX_POINT('',#196359) ;
#4182=VERTEX_POINT('',#196363) ;
#4183=VERTEX_POINT('',#196365) ;
#4184=VERTEX_POINT('',#196369) ;
#4185=VERTEX_POINT('',#196371) ;
#4186=VERTEX_POINT('',#196384) ;
#4187=VERTEX_POINT('',#196386) ;
#4188=VERTEX_POINT('',#196390) ;
#4189=VERTEX_POINT('',#196392) ;
#4190=VERTEX_POINT('',#196396) ;
#4191=VERTEX_POINT('',#196398) ;
#4192=VERTEX_POINT('',#196411) ;
#4193=VERTEX_POINT('',#196413) ;
#4194=VERTEX_POINT('',#196417) ;
#4195=VERTEX_POINT('',#196419) ;
#4196=VERTEX_POINT('',#196423) ;
#4197=VERTEX_POINT('',#196425) ;
#4198=VERTEX_POINT('',#196438) ;
#4199=VERTEX_POINT('',#196440) ;
#4200=VERTEX_POINT('',#196444) ;
#4201=VERTEX_POINT('',#196446) ;
#4202=VERTEX_POINT('',#196450) ;
#4203=VERTEX_POINT('',#196452) ;
#4204=VERTEX_POINT('',#196465) ;
#4205=VERTEX_POINT('',#196467) ;
#4206=VERTEX_POINT('',#196474) ;
#4207=VERTEX_POINT('',#196475) ;
#4208=VERTEX_POINT('',#196477) ;
#4209=VERTEX_POINT('',#196479) ;
#4210=VERTEX_POINT('',#196481) ;
#4211=VERTEX_POINT('',#196483) ;
#4212=VERTEX_POINT('',#196485) ;
#4213=VERTEX_POINT('',#196487) ;
#4214=VERTEX_POINT('',#196490) ;
#4215=VERTEX_POINT('',#196492) ;
#4216=VERTEX_POINT('',#196493) ;
#4217=VERTEX_POINT('',#196495) ;
#4218=VERTEX_POINT('',#196497) ;
#4219=VERTEX_POINT('',#196499) ;
#4220=VERTEX_POINT('',#196501) ;
#4221=VERTEX_POINT('',#196503) ;
#4222=VERTEX_POINT('',#196505) ;
#4223=VERTEX_POINT('',#196508) ;
#4224=VERTEX_POINT('',#196509) ;
#4225=VERTEX_POINT('',#196511) ;
#4226=VERTEX_POINT('',#196513) ;
#4227=VERTEX_POINT('',#196515) ;
#4228=VERTEX_POINT('',#196517) ;
#4229=VERTEX_POINT('',#196519) ;
#4230=VERTEX_POINT('',#196521) ;
#4231=VERTEX_POINT('',#196524) ;
#4232=VERTEX_POINT('',#196525) ;
#4233=VERTEX_POINT('',#196527) ;
#4234=VERTEX_POINT('',#196529) ;
#4235=VERTEX_POINT('',#196531) ;
#4236=VERTEX_POINT('',#196533) ;
#4237=VERTEX_POINT('',#196535) ;
#4238=VERTEX_POINT('',#196537) ;
#4239=VERTEX_POINT('',#196540) ;
#4240=VERTEX_POINT('',#196541) ;
#4241=VERTEX_POINT('',#196543) ;
#4242=VERTEX_POINT('',#196545) ;
#4243=VERTEX_POINT('',#196547) ;
#4244=VERTEX_POINT('',#196549) ;
#4245=VERTEX_POINT('',#196551) ;
#4246=VERTEX_POINT('',#196553) ;
#4247=VERTEX_POINT('',#196557) ;
#4248=VERTEX_POINT('',#196560) ;
#4249=VERTEX_POINT('',#196562) ;
#4250=VERTEX_POINT('',#196566) ;
#4251=VERTEX_POINT('',#196570) ;
#4252=VERTEX_POINT('',#196574) ;
#4253=VERTEX_POINT('',#196578) ;
#4254=VERTEX_POINT('',#196582) ;
#4255=VERTEX_POINT('',#196586) ;
#4256=VERTEX_POINT('',#196592) ;
#4257=VERTEX_POINT('',#196596) ;
#4258=VERTEX_POINT('',#196598) ;
#4259=VERTEX_POINT('',#196602) ;
#4260=VERTEX_POINT('',#196606) ;
#4261=VERTEX_POINT('',#196610) ;
#4262=VERTEX_POINT('',#196614) ;
#4263=VERTEX_POINT('',#196618) ;
#4264=VERTEX_POINT('',#196622) ;
#4265=VERTEX_POINT('',#196628) ;
#4266=VERTEX_POINT('',#196630) ;
#4267=VERTEX_POINT('',#196634) ;
#4268=VERTEX_POINT('',#196638) ;
#4269=VERTEX_POINT('',#196642) ;
#4270=VERTEX_POINT('',#196646) ;
#4271=VERTEX_POINT('',#196650) ;
#4272=VERTEX_POINT('',#196654) ;
#4273=VERTEX_POINT('',#196660) ;
#4274=VERTEX_POINT('',#196662) ;
#4275=VERTEX_POINT('',#196666) ;
#4276=VERTEX_POINT('',#196670) ;
#4277=VERTEX_POINT('',#196674) ;
#4278=VERTEX_POINT('',#196678) ;
#4279=VERTEX_POINT('',#196682) ;
#4280=VERTEX_POINT('',#196686) ;
#4281=VERTEX_POINT('',#196692) ;
#4282=VERTEX_POINT('',#196694) ;
#4283=VERTEX_POINT('',#196698) ;
#4284=VERTEX_POINT('',#196702) ;
#4285=VERTEX_POINT('',#196706) ;
#4286=VERTEX_POINT('',#196710) ;
#4287=VERTEX_POINT('',#196714) ;
#4288=VERTEX_POINT('',#196718) ;
#4289=VERTEX_POINT('',#196724) ;
#4290=VERTEX_POINT('',#196728) ;
#4291=VERTEX_POINT('',#196730) ;
#4899=EDGE_CURVE('',#3846,#3847,#2083,.T.) ;
#4900=EDGE_CURVE('',#3847,#3848,#2084,.T.) ;
#4901=EDGE_CURVE('',#3849,#3848,#2085,.T.) ;
#4902=EDGE_CURVE('',#3846,#3849,#2086,.T.) ;
#4903=EDGE_CURVE('',#3847,#3850,#191,.T.) ;
#4904=EDGE_CURVE('',#3850,#3851,#2087,.T.) ;
#4905=EDGE_CURVE('',#3848,#3851,#192,.T.) ;
#4906=EDGE_CURVE('',#3850,#3852,#2088,.T.) ;
#4907=EDGE_CURVE('',#3852,#3853,#2089,.T.) ;
#4908=EDGE_CURVE('',#3851,#3853,#2090,.T.) ;
#4909=EDGE_CURVE('',#3852,#3854,#2091,.T.) ;
#4910=EDGE_CURVE('',#3854,#3855,#2092,.T.) ;
#4911=EDGE_CURVE('',#3853,#3855,#2093,.T.) ;
#4912=EDGE_CURVE('',#3854,#3856,#193,.T.) ;
#4913=EDGE_CURVE('',#3856,#3857,#2094,.T.) ;
#4914=EDGE_CURVE('',#3855,#3857,#194,.T.) ;
#4915=EDGE_CURVE('',#3856,#3858,#2095,.T.) ;
#4916=EDGE_CURVE('',#3858,#3859,#2096,.T.) ;
#4917=EDGE_CURVE('',#3857,#3859,#2097,.T.) ;
#4918=EDGE_CURVE('',#3858,#3860,#2098,.T.) ;
#4919=EDGE_CURVE('',#3860,#3861,#2099,.T.) ;
#4920=EDGE_CURVE('',#3859,#3861,#2100,.T.) ;
#4921=EDGE_CURVE('',#3860,#3862,#195,.T.) ;
#4922=EDGE_CURVE('',#3862,#3863,#2101,.T.) ;
#4923=EDGE_CURVE('',#3861,#3863,#196,.T.) ;
#4924=EDGE_CURVE('',#3862,#3864,#2102,.T.) ;
#4925=EDGE_CURVE('',#3864,#3865,#2103,.T.) ;
#4926=EDGE_CURVE('',#3863,#3865,#2104,.T.) ;
#4927=EDGE_CURVE('',#3864,#3866,#2105,.T.) ;
#4928=EDGE_CURVE('',#3866,#3867,#2106,.T.) ;
#4929=EDGE_CURVE('',#3865,#3867,#2107,.T.) ;
#4930=EDGE_CURVE('',#3866,#3868,#197,.T.) ;
#4931=EDGE_CURVE('',#3868,#3869,#2108,.T.) ;
#4932=EDGE_CURVE('',#3867,#3869,#198,.T.) ;
#4933=EDGE_CURVE('',#3868,#3870,#2109,.T.) ;
#4934=EDGE_CURVE('',#3870,#3871,#2110,.T.) ;
#4935=EDGE_CURVE('',#3869,#3871,#2111,.T.) ;
#4936=EDGE_CURVE('',#3870,#3872,#2112,.T.) ;
#4937=EDGE_CURVE('',#3872,#3873,#2113,.T.) ;
#4938=EDGE_CURVE('',#3871,#3873,#2114,.T.) ;
#4939=EDGE_CURVE('',#3872,#3874,#199,.T.) ;
#4940=EDGE_CURVE('',#3874,#3875,#2115,.T.) ;
#4941=EDGE_CURVE('',#3873,#3875,#200,.T.) ;
#4942=EDGE_CURVE('',#3874,#3876,#2116,.T.) ;
#4943=EDGE_CURVE('',#3876,#3877,#2117,.T.) ;
#4944=EDGE_CURVE('',#3875,#3877,#2118,.T.) ;
#4945=EDGE_CURVE('',#3876,#3878,#2119,.T.) ;
#4946=EDGE_CURVE('',#3878,#3879,#2120,.T.) ;
#4947=EDGE_CURVE('',#3877,#3879,#2121,.T.) ;
#4948=EDGE_CURVE('',#3878,#3880,#201,.T.) ;
#4949=EDGE_CURVE('',#3880,#3881,#2122,.T.) ;
#4950=EDGE_CURVE('',#3879,#3881,#202,.T.) ;
#4951=EDGE_CURVE('',#3880,#3882,#2123,.T.) ;
#4952=EDGE_CURVE('',#3882,#3883,#2124,.T.) ;
#4953=EDGE_CURVE('',#3881,#3883,#2125,.T.) ;
#4954=EDGE_CURVE('',#3882,#3884,#2126,.T.) ;
#4955=EDGE_CURVE('',#3884,#3885,#2127,.T.) ;
#4956=EDGE_CURVE('',#3883,#3885,#2128,.T.) ;
#4957=EDGE_CURVE('',#3884,#3886,#203,.T.) ;
#4958=EDGE_CURVE('',#3886,#3887,#2129,.T.) ;
#4959=EDGE_CURVE('',#3885,#3887,#204,.T.) ;
#4960=EDGE_CURVE('',#3886,#3888,#2130,.T.) ;
#4961=EDGE_CURVE('',#3888,#3889,#2131,.T.) ;
#4962=EDGE_CURVE('',#3887,#3889,#2132,.T.) ;
#4963=EDGE_CURVE('',#3888,#3890,#2133,.T.) ;
#4964=EDGE_CURVE('',#3890,#3891,#2134,.T.) ;
#4965=EDGE_CURVE('',#3889,#3891,#2135,.T.) ;
#4966=EDGE_CURVE('',#3890,#3892,#205,.T.) ;
#4967=EDGE_CURVE('',#3892,#3893,#2136,.T.) ;
#4968=EDGE_CURVE('',#3891,#3893,#206,.T.) ;
#4969=EDGE_CURVE('',#3892,#3894,#2137,.T.) ;
#4970=EDGE_CURVE('',#3894,#3895,#2138,.T.) ;
#4971=EDGE_CURVE('',#3893,#3895,#2139,.T.) ;
#4972=EDGE_CURVE('',#3894,#3896,#2140,.T.) ;
#4973=EDGE_CURVE('',#3896,#3897,#2141,.T.) ;
#4974=EDGE_CURVE('',#3895,#3897,#2142,.T.) ;
#4975=EDGE_CURVE('',#3896,#3898,#207,.T.) ;
#4976=EDGE_CURVE('',#3898,#3899,#2143,.T.) ;
#4977=EDGE_CURVE('',#3897,#3899,#208,.T.) ;
#4978=EDGE_CURVE('',#3898,#3900,#2144,.T.) ;
#4979=EDGE_CURVE('',#3900,#3901,#2145,.T.) ;
#4980=EDGE_CURVE('',#3899,#3901,#2146,.T.) ;
#4981=EDGE_CURVE('',#3900,#3902,#2147,.T.) ;
#4982=EDGE_CURVE('',#3902,#3903,#2148,.T.) ;
#4983=EDGE_CURVE('',#3901,#3903,#2149,.T.) ;
#4984=EDGE_CURVE('',#3902,#3904,#209,.T.) ;
#4985=EDGE_CURVE('',#3904,#3905,#2150,.T.) ;
#4986=EDGE_CURVE('',#3903,#3905,#210,.T.) ;
#4987=EDGE_CURVE('',#3904,#3906,#2151,.T.) ;
#4988=EDGE_CURVE('',#3906,#3907,#2152,.T.) ;
#4989=EDGE_CURVE('',#3905,#3907,#2153,.T.) ;
#4990=EDGE_CURVE('',#3906,#3908,#2154,.T.) ;
#4991=EDGE_CURVE('',#3908,#3909,#2155,.T.) ;
#4992=EDGE_CURVE('',#3907,#3909,#2156,.T.) ;
#4993=EDGE_CURVE('',#3908,#3910,#211,.T.) ;
#4994=EDGE_CURVE('',#3910,#3911,#2157,.T.) ;
#4995=EDGE_CURVE('',#3909,#3911,#212,.T.) ;
#4996=EDGE_CURVE('',#3910,#3912,#2158,.T.) ;
#4997=EDGE_CURVE('',#3912,#3913,#2159,.T.) ;
#4998=EDGE_CURVE('',#3911,#3913,#2160,.T.) ;
#4999=EDGE_CURVE('',#3912,#3914,#2161,.T.) ;
#5000=EDGE_CURVE('',#3914,#3915,#2162,.T.) ;
#5001=EDGE_CURVE('',#3913,#3915,#2163,.T.) ;
#5002=EDGE_CURVE('',#3914,#3916,#213,.T.) ;
#5003=EDGE_CURVE('',#3916,#3917,#2164,.T.) ;
#5004=EDGE_CURVE('',#3915,#3917,#214,.T.) ;
#5005=EDGE_CURVE('',#3916,#3918,#2165,.T.) ;
#5006=EDGE_CURVE('',#3918,#3919,#2166,.T.) ;
#5007=EDGE_CURVE('',#3917,#3919,#2167,.T.) ;
#5008=EDGE_CURVE('',#3918,#3920,#2168,.T.) ;
#5009=EDGE_CURVE('',#3920,#3921,#2169,.T.) ;
#5010=EDGE_CURVE('',#3919,#3921,#2170,.T.) ;
#5011=EDGE_CURVE('',#3920,#3922,#215,.T.) ;
#5012=EDGE_CURVE('',#3922,#3923,#2171,.T.) ;
#5013=EDGE_CURVE('',#3921,#3923,#216,.T.) ;
#5014=EDGE_CURVE('',#3922,#3924,#2172,.T.) ;
#5015=EDGE_CURVE('',#3924,#3925,#2173,.T.) ;
#5016=EDGE_CURVE('',#3923,#3925,#2174,.T.) ;
#5017=EDGE_CURVE('',#3924,#3926,#2175,.T.) ;
#5018=EDGE_CURVE('',#3926,#3927,#2176,.T.) ;
#5019=EDGE_CURVE('',#3925,#3927,#2177,.T.) ;
#5020=EDGE_CURVE('',#3926,#3928,#217,.T.) ;
#5021=EDGE_CURVE('',#3928,#3929,#2178,.T.) ;
#5022=EDGE_CURVE('',#3927,#3929,#218,.T.) ;
#5023=EDGE_CURVE('',#3928,#3930,#2179,.T.) ;
#5024=EDGE_CURVE('',#3930,#3931,#2180,.T.) ;
#5025=EDGE_CURVE('',#3929,#3931,#2181,.T.) ;
#5026=EDGE_CURVE('',#3930,#3932,#2182,.T.) ;
#5027=EDGE_CURVE('',#3932,#3933,#2183,.T.) ;
#5028=EDGE_CURVE('',#3931,#3933,#2184,.T.) ;
#5029=EDGE_CURVE('',#3932,#3934,#219,.T.) ;
#5030=EDGE_CURVE('',#3934,#3935,#2185,.T.) ;
#5031=EDGE_CURVE('',#3933,#3935,#220,.T.) ;
#5032=EDGE_CURVE('',#3934,#3936,#2186,.T.) ;
#5033=EDGE_CURVE('',#3936,#3937,#2187,.T.) ;
#5034=EDGE_CURVE('',#3935,#3937,#2188,.T.) ;
#5035=EDGE_CURVE('',#3936,#3938,#2189,.T.) ;
#5036=EDGE_CURVE('',#3938,#3939,#2190,.T.) ;
#5037=EDGE_CURVE('',#3937,#3939,#2191,.T.) ;
#5038=EDGE_CURVE('',#3938,#3940,#221,.T.) ;
#5039=EDGE_CURVE('',#3940,#3941,#2192,.T.) ;
#5040=EDGE_CURVE('',#3939,#3941,#222,.T.) ;
#5041=EDGE_CURVE('',#3940,#3942,#2193,.T.) ;
#5042=EDGE_CURVE('',#3942,#3943,#2194,.T.) ;
#5043=EDGE_CURVE('',#3941,#3943,#2195,.T.) ;
#5044=EDGE_CURVE('',#3942,#3944,#2196,.T.) ;
#5045=EDGE_CURVE('',#3944,#3945,#2197,.T.) ;
#5046=EDGE_CURVE('',#3943,#3945,#2198,.T.) ;
#5047=EDGE_CURVE('',#3944,#3946,#223,.T.) ;
#5048=EDGE_CURVE('',#3946,#3947,#2199,.T.) ;
#5049=EDGE_CURVE('',#3945,#3947,#224,.T.) ;
#5050=EDGE_CURVE('',#3946,#3948,#2200,.T.) ;
#5051=EDGE_CURVE('',#3948,#3949,#2201,.T.) ;
#5052=EDGE_CURVE('',#3947,#3949,#2202,.T.) ;
#5053=EDGE_CURVE('',#3948,#3950,#2203,.T.) ;
#5054=EDGE_CURVE('',#3950,#3951,#2204,.T.) ;
#5055=EDGE_CURVE('',#3949,#3951,#2205,.T.) ;
#5056=EDGE_CURVE('',#3950,#3952,#225,.T.) ;
#5057=EDGE_CURVE('',#3952,#3953,#2206,.T.) ;
#5058=EDGE_CURVE('',#3951,#3953,#226,.T.) ;
#5059=EDGE_CURVE('',#3952,#3954,#2207,.T.) ;
#5060=EDGE_CURVE('',#3954,#3955,#2208,.T.) ;
#5061=EDGE_CURVE('',#3953,#3955,#2209,.T.) ;
#5062=EDGE_CURVE('',#3954,#3956,#2210,.T.) ;
#5063=EDGE_CURVE('',#3956,#3957,#2211,.T.) ;
#5064=EDGE_CURVE('',#3955,#3957,#2212,.T.) ;
#5065=EDGE_CURVE('',#3956,#3958,#227,.T.) ;
#5066=EDGE_CURVE('',#3958,#3959,#2213,.T.) ;
#5067=EDGE_CURVE('',#3957,#3959,#228,.T.) ;
#5068=EDGE_CURVE('',#3958,#3960,#2214,.T.) ;
#5069=EDGE_CURVE('',#3960,#3961,#2215,.T.) ;
#5070=EDGE_CURVE('',#3959,#3961,#2216,.T.) ;
#5071=EDGE_CURVE('',#3960,#3962,#2217,.T.) ;
#5072=EDGE_CURVE('',#3962,#3963,#2218,.T.) ;
#5073=EDGE_CURVE('',#3961,#3963,#2219,.T.) ;
#5074=EDGE_CURVE('',#3962,#3964,#229,.T.) ;
#5075=EDGE_CURVE('',#3964,#3965,#2220,.T.) ;
#5076=EDGE_CURVE('',#3963,#3965,#230,.T.) ;
#5077=EDGE_CURVE('',#3964,#3966,#2221,.T.) ;
#5078=EDGE_CURVE('',#3966,#3967,#2222,.T.) ;
#5079=EDGE_CURVE('',#3965,#3967,#2223,.T.) ;
#5080=EDGE_CURVE('',#3966,#3968,#2224,.T.) ;
#5081=EDGE_CURVE('',#3968,#3969,#2225,.T.) ;
#5082=EDGE_CURVE('',#3967,#3969,#2226,.T.) ;
#5083=EDGE_CURVE('',#3968,#3970,#231,.T.) ;
#5084=EDGE_CURVE('',#3970,#3971,#2227,.T.) ;
#5085=EDGE_CURVE('',#3969,#3971,#232,.T.) ;
#5086=EDGE_CURVE('',#3970,#3972,#2228,.T.) ;
#5087=EDGE_CURVE('',#3972,#3973,#2229,.T.) ;
#5088=EDGE_CURVE('',#3971,#3973,#2230,.T.) ;
#5089=EDGE_CURVE('',#3972,#3974,#2231,.T.) ;
#5090=EDGE_CURVE('',#3974,#3975,#2232,.T.) ;
#5091=EDGE_CURVE('',#3973,#3975,#2233,.T.) ;
#5092=EDGE_CURVE('',#3974,#3976,#233,.T.) ;
#5093=EDGE_CURVE('',#3976,#3977,#2234,.T.) ;
#5094=EDGE_CURVE('',#3975,#3977,#234,.T.) ;
#5095=EDGE_CURVE('',#3976,#3978,#2235,.T.) ;
#5096=EDGE_CURVE('',#3978,#3979,#2236,.T.) ;
#5097=EDGE_CURVE('',#3977,#3979,#2237,.T.) ;
#5098=EDGE_CURVE('',#3978,#3980,#2238,.T.) ;
#5099=EDGE_CURVE('',#3980,#3981,#2239,.T.) ;
#5100=EDGE_CURVE('',#3979,#3981,#2240,.T.) ;
#5101=EDGE_CURVE('',#3980,#3982,#235,.T.) ;
#5102=EDGE_CURVE('',#3982,#3983,#2241,.T.) ;
#5103=EDGE_CURVE('',#3981,#3983,#236,.T.) ;
#5104=EDGE_CURVE('',#3982,#3984,#2242,.T.) ;
#5105=EDGE_CURVE('',#3984,#3985,#2243,.T.) ;
#5106=EDGE_CURVE('',#3983,#3985,#2244,.T.) ;
#5107=EDGE_CURVE('',#3984,#3986,#2245,.T.) ;
#5108=EDGE_CURVE('',#3986,#3987,#2246,.T.) ;
#5109=EDGE_CURVE('',#3985,#3987,#2247,.T.) ;
#5110=EDGE_CURVE('',#3986,#3988,#237,.T.) ;
#5111=EDGE_CURVE('',#3988,#3989,#2248,.T.) ;
#5112=EDGE_CURVE('',#3987,#3989,#238,.T.) ;
#5113=EDGE_CURVE('',#3988,#3990,#2249,.T.) ;
#5114=EDGE_CURVE('',#3990,#3991,#2250,.T.) ;
#5115=EDGE_CURVE('',#3989,#3991,#2251,.T.) ;
#5116=EDGE_CURVE('',#3990,#3992,#2252,.T.) ;
#5117=EDGE_CURVE('',#3992,#3993,#2253,.T.) ;
#5118=EDGE_CURVE('',#3991,#3993,#2254,.T.) ;
#5119=EDGE_CURVE('',#3992,#3994,#239,.T.) ;
#5120=EDGE_CURVE('',#3994,#3995,#2255,.T.) ;
#5121=EDGE_CURVE('',#3993,#3995,#240,.T.) ;
#5122=EDGE_CURVE('',#3994,#3996,#2256,.T.) ;
#5123=EDGE_CURVE('',#3996,#3997,#2257,.T.) ;
#5124=EDGE_CURVE('',#3995,#3997,#2258,.T.) ;
#5125=EDGE_CURVE('',#3996,#3998,#2259,.T.) ;
#5126=EDGE_CURVE('',#3998,#3999,#2260,.T.) ;
#5127=EDGE_CURVE('',#3997,#3999,#2261,.T.) ;
#5128=EDGE_CURVE('',#3998,#4000,#241,.T.) ;
#5129=EDGE_CURVE('',#4000,#4001,#2262,.T.) ;
#5130=EDGE_CURVE('',#3999,#4001,#242,.T.) ;
#5131=EDGE_CURVE('',#4000,#4002,#2263,.T.) ;
#5132=EDGE_CURVE('',#4002,#4003,#2264,.T.) ;
#5133=EDGE_CURVE('',#4001,#4003,#2265,.T.) ;
#5134=EDGE_CURVE('',#4002,#4004,#2266,.T.) ;
#5135=EDGE_CURVE('',#4004,#4005,#2267,.T.) ;
#5136=EDGE_CURVE('',#4003,#4005,#2268,.T.) ;
#5137=EDGE_CURVE('',#4004,#4006,#243,.T.) ;
#5138=EDGE_CURVE('',#4006,#4007,#2269,.T.) ;
#5139=EDGE_CURVE('',#4005,#4007,#244,.T.) ;
#5140=EDGE_CURVE('',#4006,#4008,#2270,.T.) ;
#5141=EDGE_CURVE('',#4008,#4009,#2271,.T.) ;
#5142=EDGE_CURVE('',#4007,#4009,#2272,.T.) ;
#5143=EDGE_CURVE('',#4008,#4010,#2273,.T.) ;
#5144=EDGE_CURVE('',#4010,#4011,#2274,.T.) ;
#5145=EDGE_CURVE('',#4009,#4011,#2275,.T.) ;
#5146=EDGE_CURVE('',#4010,#4012,#245,.T.) ;
#5147=EDGE_CURVE('',#4012,#4013,#2276,.T.) ;
#5148=EDGE_CURVE('',#4011,#4013,#246,.T.) ;
#5149=EDGE_CURVE('',#4012,#4014,#2277,.T.) ;
#5150=EDGE_CURVE('',#4014,#4015,#2278,.T.) ;
#5151=EDGE_CURVE('',#4013,#4015,#2279,.T.) ;
#5152=EDGE_CURVE('',#4014,#4016,#2280,.T.) ;
#5153=EDGE_CURVE('',#4016,#4017,#2281,.T.) ;
#5154=EDGE_CURVE('',#4015,#4017,#2282,.T.) ;
#5155=EDGE_CURVE('',#4016,#4018,#247,.T.) ;
#5156=EDGE_CURVE('',#4018,#4019,#2283,.T.) ;
#5157=EDGE_CURVE('',#4017,#4019,#248,.T.) ;
#5158=EDGE_CURVE('',#4018,#4020,#2284,.T.) ;
#5159=EDGE_CURVE('',#4020,#4021,#2285,.T.) ;
#5160=EDGE_CURVE('',#4019,#4021,#2286,.T.) ;
#5161=EDGE_CURVE('',#4020,#4022,#2287,.T.) ;
#5162=EDGE_CURVE('',#4022,#4023,#2288,.T.) ;
#5163=EDGE_CURVE('',#4021,#4023,#2289,.T.) ;
#5164=EDGE_CURVE('',#4022,#4024,#249,.T.) ;
#5165=EDGE_CURVE('',#4024,#4025,#2290,.T.) ;
#5166=EDGE_CURVE('',#4023,#4025,#250,.T.) ;
#5167=EDGE_CURVE('',#4024,#4026,#2291,.T.) ;
#5168=EDGE_CURVE('',#4026,#4027,#2292,.T.) ;
#5169=EDGE_CURVE('',#4025,#4027,#2293,.T.) ;
#5170=EDGE_CURVE('',#4026,#4028,#2294,.T.) ;
#5171=EDGE_CURVE('',#4028,#4029,#2295,.T.) ;
#5172=EDGE_CURVE('',#4027,#4029,#2296,.T.) ;
#5173=EDGE_CURVE('',#4028,#4030,#251,.T.) ;
#5174=EDGE_CURVE('',#4030,#4031,#2297,.T.) ;
#5175=EDGE_CURVE('',#4029,#4031,#252,.T.) ;
#5176=EDGE_CURVE('',#4030,#4032,#2298,.T.) ;
#5177=EDGE_CURVE('',#4032,#4033,#2299,.T.) ;
#5178=EDGE_CURVE('',#4031,#4033,#2300,.T.) ;
#5179=EDGE_CURVE('',#4032,#4034,#2301,.T.) ;
#5180=EDGE_CURVE('',#4034,#4035,#2302,.T.) ;
#5181=EDGE_CURVE('',#4033,#4035,#2303,.T.) ;
#5182=EDGE_CURVE('',#4034,#4036,#253,.T.) ;
#5183=EDGE_CURVE('',#4036,#4037,#2304,.T.) ;
#5184=EDGE_CURVE('',#4035,#4037,#254,.T.) ;
#5185=EDGE_CURVE('',#4036,#4038,#2305,.T.) ;
#5186=EDGE_CURVE('',#4038,#4039,#2306,.T.) ;
#5187=EDGE_CURVE('',#4037,#4039,#2307,.T.) ;
#5188=EDGE_CURVE('',#4038,#4040,#2308,.T.) ;
#5189=EDGE_CURVE('',#4040,#4041,#2309,.T.) ;
#5190=EDGE_CURVE('',#4039,#4041,#2310,.T.) ;
#5191=EDGE_CURVE('',#4040,#4042,#255,.T.) ;
#5192=EDGE_CURVE('',#4042,#4043,#2311,.T.) ;
#5193=EDGE_CURVE('',#4041,#4043,#256,.T.) ;
#5194=EDGE_CURVE('',#4042,#4044,#2312,.T.) ;
#5195=EDGE_CURVE('',#4044,#4045,#2313,.T.) ;
#5196=EDGE_CURVE('',#4043,#4045,#2314,.T.) ;
#5197=EDGE_CURVE('',#4044,#4046,#2315,.T.) ;
#5198=EDGE_CURVE('',#4046,#4047,#2316,.T.) ;
#5199=EDGE_CURVE('',#4045,#4047,#2317,.T.) ;
#5200=EDGE_CURVE('',#4046,#4048,#257,.T.) ;
#5201=EDGE_CURVE('',#4048,#4049,#2318,.T.) ;
#5202=EDGE_CURVE('',#4047,#4049,#258,.T.) ;
#5203=EDGE_CURVE('',#4048,#4050,#2319,.T.) ;
#5204=EDGE_CURVE('',#4050,#4051,#2320,.T.) ;
#5205=EDGE_CURVE('',#4049,#4051,#2321,.T.) ;
#5206=EDGE_CURVE('',#4050,#4052,#2322,.T.) ;
#5207=EDGE_CURVE('',#4052,#4053,#2323,.T.) ;
#5208=EDGE_CURVE('',#4051,#4053,#2324,.T.) ;
#5209=EDGE_CURVE('',#4052,#4054,#259,.T.) ;
#5210=EDGE_CURVE('',#4054,#4055,#2325,.T.) ;
#5211=EDGE_CURVE('',#4053,#4055,#260,.T.) ;
#5212=EDGE_CURVE('',#4054,#4056,#2326,.T.) ;
#5213=EDGE_CURVE('',#4056,#4057,#2327,.T.) ;
#5214=EDGE_CURVE('',#4055,#4057,#2328,.T.) ;
#5215=EDGE_CURVE('',#4056,#4058,#2329,.T.) ;
#5216=EDGE_CURVE('',#4058,#4059,#2330,.T.) ;
#5217=EDGE_CURVE('',#4057,#4059,#2331,.T.) ;
#5218=EDGE_CURVE('',#4058,#4060,#261,.T.) ;
#5219=EDGE_CURVE('',#4060,#4061,#2332,.T.) ;
#5220=EDGE_CURVE('',#4059,#4061,#262,.T.) ;
#5221=EDGE_CURVE('',#4060,#4062,#2333,.T.) ;
#5222=EDGE_CURVE('',#4062,#4063,#2334,.T.) ;
#5223=EDGE_CURVE('',#4061,#4063,#2335,.T.) ;
#5224=EDGE_CURVE('',#4062,#4064,#2336,.T.) ;
#5225=EDGE_CURVE('',#4064,#4065,#2337,.T.) ;
#5226=EDGE_CURVE('',#4063,#4065,#2338,.T.) ;
#5227=EDGE_CURVE('',#4064,#4066,#263,.T.) ;
#5228=EDGE_CURVE('',#4066,#4067,#2339,.T.) ;
#5229=EDGE_CURVE('',#4065,#4067,#264,.T.) ;
#5230=EDGE_CURVE('',#4066,#4068,#2340,.T.) ;
#5231=EDGE_CURVE('',#4068,#4069,#2341,.T.) ;
#5232=EDGE_CURVE('',#4067,#4069,#2342,.T.) ;
#5233=EDGE_CURVE('',#4068,#4070,#2343,.T.) ;
#5234=EDGE_CURVE('',#4070,#4071,#2344,.T.) ;
#5235=EDGE_CURVE('',#4069,#4071,#2345,.T.) ;
#5236=EDGE_CURVE('',#4070,#4072,#265,.T.) ;
#5237=EDGE_CURVE('',#4072,#4073,#2346,.T.) ;
#5238=EDGE_CURVE('',#4071,#4073,#266,.T.) ;
#5239=EDGE_CURVE('',#4072,#4074,#2347,.T.) ;
#5240=EDGE_CURVE('',#4074,#4075,#2348,.T.) ;
#5241=EDGE_CURVE('',#4073,#4075,#2349,.T.) ;
#5242=EDGE_CURVE('',#4074,#4076,#2350,.T.) ;
#5243=EDGE_CURVE('',#4076,#4077,#2351,.T.) ;
#5244=EDGE_CURVE('',#4075,#4077,#2352,.T.) ;
#5245=EDGE_CURVE('',#4076,#4078,#267,.T.) ;
#5246=EDGE_CURVE('',#4078,#4079,#2353,.T.) ;
#5247=EDGE_CURVE('',#4077,#4079,#268,.T.) ;
#5248=EDGE_CURVE('',#4078,#4080,#2354,.T.) ;
#5249=EDGE_CURVE('',#4080,#4081,#2355,.T.) ;
#5250=EDGE_CURVE('',#4079,#4081,#2356,.T.) ;
#5251=EDGE_CURVE('',#4080,#4082,#2357,.T.) ;
#5252=EDGE_CURVE('',#4082,#4083,#2358,.T.) ;
#5253=EDGE_CURVE('',#4081,#4083,#2359,.T.) ;
#5254=EDGE_CURVE('',#4082,#4084,#269,.T.) ;
#5255=EDGE_CURVE('',#4084,#4085,#2360,.T.) ;
#5256=EDGE_CURVE('',#4083,#4085,#270,.T.) ;
#5257=EDGE_CURVE('',#4084,#4086,#2361,.T.) ;
#5258=EDGE_CURVE('',#4086,#4087,#2362,.T.) ;
#5259=EDGE_CURVE('',#4085,#4087,#2363,.T.) ;
#5260=EDGE_CURVE('',#4086,#4088,#2364,.T.) ;
#5261=EDGE_CURVE('',#4088,#4089,#2365,.T.) ;
#5262=EDGE_CURVE('',#4087,#4089,#2366,.T.) ;
#5263=EDGE_CURVE('',#4088,#4090,#271,.T.) ;
#5264=EDGE_CURVE('',#4090,#4091,#2367,.T.) ;
#5265=EDGE_CURVE('',#4089,#4091,#272,.T.) ;
#5266=EDGE_CURVE('',#4090,#4092,#2368,.T.) ;
#5267=EDGE_CURVE('',#4092,#4093,#2369,.T.) ;
#5268=EDGE_CURVE('',#4091,#4093,#2370,.T.) ;
#5269=EDGE_CURVE('',#4092,#4094,#2371,.T.) ;
#5270=EDGE_CURVE('',#4094,#4095,#2372,.T.) ;
#5271=EDGE_CURVE('',#4093,#4095,#2373,.T.) ;
#5272=EDGE_CURVE('',#4094,#4096,#273,.T.) ;
#5273=EDGE_CURVE('',#4096,#4097,#2374,.T.) ;
#5274=EDGE_CURVE('',#4095,#4097,#274,.T.) ;
#5275=EDGE_CURVE('',#4096,#4098,#2375,.T.) ;
#5276=EDGE_CURVE('',#4098,#4099,#2376,.T.) ;
#5277=EDGE_CURVE('',#4097,#4099,#2377,.T.) ;
#5278=EDGE_CURVE('',#4098,#4100,#2378,.T.) ;
#5279=EDGE_CURVE('',#4100,#4101,#2379,.T.) ;
#5280=EDGE_CURVE('',#4099,#4101,#2380,.T.) ;
#5281=EDGE_CURVE('',#4100,#4102,#275,.T.) ;
#5282=EDGE_CURVE('',#4102,#4103,#2381,.T.) ;
#5283=EDGE_CURVE('',#4101,#4103,#276,.T.) ;
#5284=EDGE_CURVE('',#4102,#4104,#2382,.T.) ;
#5285=EDGE_CURVE('',#4104,#4105,#2383,.T.) ;
#5286=EDGE_CURVE('',#4103,#4105,#2384,.T.) ;
#5287=EDGE_CURVE('',#4104,#4106,#2385,.T.) ;
#5288=EDGE_CURVE('',#4106,#4107,#2386,.T.) ;
#5289=EDGE_CURVE('',#4105,#4107,#2387,.T.) ;
#5290=EDGE_CURVE('',#4106,#4108,#277,.T.) ;
#5291=EDGE_CURVE('',#4108,#4109,#2388,.T.) ;
#5292=EDGE_CURVE('',#4107,#4109,#278,.T.) ;
#5293=EDGE_CURVE('',#4108,#4110,#2389,.T.) ;
#5294=EDGE_CURVE('',#4110,#4111,#2390,.T.) ;
#5295=EDGE_CURVE('',#4109,#4111,#2391,.T.) ;
#5296=EDGE_CURVE('',#4110,#4112,#2392,.T.) ;
#5297=EDGE_CURVE('',#4112,#4113,#2393,.T.) ;
#5298=EDGE_CURVE('',#4111,#4113,#2394,.T.) ;
#5299=EDGE_CURVE('',#4112,#4114,#279,.T.) ;
#5300=EDGE_CURVE('',#4114,#4115,#2395,.T.) ;
#5301=EDGE_CURVE('',#4113,#4115,#280,.T.) ;
#5302=EDGE_CURVE('',#4114,#4116,#2396,.T.) ;
#5303=EDGE_CURVE('',#4116,#4117,#2397,.T.) ;
#5304=EDGE_CURVE('',#4115,#4117,#2398,.T.) ;
#5305=EDGE_CURVE('',#4116,#4118,#2399,.T.) ;
#5306=EDGE_CURVE('',#4118,#4119,#2400,.T.) ;
#5307=EDGE_CURVE('',#4117,#4119,#2401,.T.) ;
#5308=EDGE_CURVE('',#4118,#4120,#281,.T.) ;
#5309=EDGE_CURVE('',#4120,#4121,#2402,.T.) ;
#5310=EDGE_CURVE('',#4119,#4121,#282,.T.) ;
#5311=EDGE_CURVE('',#4120,#4122,#2403,.T.) ;
#5312=EDGE_CURVE('',#4122,#4123,#2404,.T.) ;
#5313=EDGE_CURVE('',#4121,#4123,#2405,.T.) ;
#5314=EDGE_CURVE('',#4122,#4124,#2406,.T.) ;
#5315=EDGE_CURVE('',#4124,#4125,#2407,.T.) ;
#5316=EDGE_CURVE('',#4123,#4125,#2408,.T.) ;
#5317=EDGE_CURVE('',#4124,#4126,#283,.T.) ;
#5318=EDGE_CURVE('',#4126,#4127,#2409,.T.) ;
#5319=EDGE_CURVE('',#4125,#4127,#284,.T.) ;
#5320=EDGE_CURVE('',#4126,#4128,#2410,.T.) ;
#5321=EDGE_CURVE('',#4128,#4129,#2411,.T.) ;
#5322=EDGE_CURVE('',#4127,#4129,#2412,.T.) ;
#5323=EDGE_CURVE('',#4128,#4130,#2413,.T.) ;
#5324=EDGE_CURVE('',#4130,#4131,#2414,.T.) ;
#5325=EDGE_CURVE('',#4129,#4131,#2415,.T.) ;
#5326=EDGE_CURVE('',#4130,#4132,#285,.T.) ;
#5327=EDGE_CURVE('',#4132,#4133,#2416,.T.) ;
#5328=EDGE_CURVE('',#4131,#4133,#286,.T.) ;
#5329=EDGE_CURVE('',#4132,#4134,#2417,.T.) ;
#5330=EDGE_CURVE('',#4134,#4135,#2418,.T.) ;
#5331=EDGE_CURVE('',#4133,#4135,#2419,.T.) ;
#5332=EDGE_CURVE('',#4134,#4136,#2420,.T.) ;
#5333=EDGE_CURVE('',#4136,#4137,#2421,.T.) ;
#5334=EDGE_CURVE('',#4135,#4137,#2422,.T.) ;
#5335=EDGE_CURVE('',#4136,#4138,#287,.T.) ;
#5336=EDGE_CURVE('',#4138,#4139,#2423,.T.) ;
#5337=EDGE_CURVE('',#4137,#4139,#288,.T.) ;
#5338=EDGE_CURVE('',#4138,#4140,#2424,.T.) ;
#5339=EDGE_CURVE('',#4140,#4141,#2425,.T.) ;
#5340=EDGE_CURVE('',#4139,#4141,#2426,.T.) ;
#5341=EDGE_CURVE('',#4140,#4142,#2427,.T.) ;
#5342=EDGE_CURVE('',#4142,#4143,#2428,.T.) ;
#5343=EDGE_CURVE('',#4141,#4143,#2429,.T.) ;
#5344=EDGE_CURVE('',#4142,#4144,#289,.T.) ;
#5345=EDGE_CURVE('',#4144,#4145,#2430,.T.) ;
#5346=EDGE_CURVE('',#4143,#4145,#290,.T.) ;
#5347=EDGE_CURVE('',#4144,#4146,#2431,.T.) ;
#5348=EDGE_CURVE('',#4146,#4147,#2432,.T.) ;
#5349=EDGE_CURVE('',#4145,#4147,#2433,.T.) ;
#5350=EDGE_CURVE('',#4146,#4148,#2434,.T.) ;
#5351=EDGE_CURVE('',#4148,#4149,#2435,.T.) ;
#5352=EDGE_CURVE('',#4147,#4149,#2436,.T.) ;
#5353=EDGE_CURVE('',#4148,#4150,#291,.T.) ;
#5354=EDGE_CURVE('',#4150,#4151,#2437,.T.) ;
#5355=EDGE_CURVE('',#4149,#4151,#292,.T.) ;
#5356=EDGE_CURVE('',#4150,#4152,#2438,.T.) ;
#5357=EDGE_CURVE('',#4152,#4153,#2439,.T.) ;
#5358=EDGE_CURVE('',#4151,#4153,#2440,.T.) ;
#5359=EDGE_CURVE('',#4152,#4154,#2441,.T.) ;
#5360=EDGE_CURVE('',#4154,#4155,#2442,.T.) ;
#5361=EDGE_CURVE('',#4153,#4155,#2443,.T.) ;
#5362=EDGE_CURVE('',#4154,#4156,#293,.T.) ;
#5363=EDGE_CURVE('',#4156,#4157,#2444,.T.) ;
#5364=EDGE_CURVE('',#4155,#4157,#294,.T.) ;
#5365=EDGE_CURVE('',#4156,#4158,#2445,.T.) ;
#5366=EDGE_CURVE('',#4158,#4159,#2446,.T.) ;
#5367=EDGE_CURVE('',#4157,#4159,#2447,.T.) ;
#5368=EDGE_CURVE('',#4158,#4160,#2448,.T.) ;
#5369=EDGE_CURVE('',#4160,#4161,#2449,.T.) ;
#5370=EDGE_CURVE('',#4159,#4161,#2450,.T.) ;
#5371=EDGE_CURVE('',#4160,#4162,#295,.T.) ;
#5372=EDGE_CURVE('',#4162,#4163,#2451,.T.) ;
#5373=EDGE_CURVE('',#4161,#4163,#296,.T.) ;
#5374=EDGE_CURVE('',#4162,#4164,#2452,.T.) ;
#5375=EDGE_CURVE('',#4164,#4165,#2453,.T.) ;
#5376=EDGE_CURVE('',#4163,#4165,#2454,.T.) ;
#5377=EDGE_CURVE('',#4164,#4166,#2455,.T.) ;
#5378=EDGE_CURVE('',#4166,#4167,#2456,.T.) ;
#5379=EDGE_CURVE('',#4165,#4167,#2457,.T.) ;
#5380=EDGE_CURVE('',#4166,#4168,#297,.T.) ;
#5381=EDGE_CURVE('',#4168,#4169,#2458,.T.) ;
#5382=EDGE_CURVE('',#4167,#4169,#298,.T.) ;
#5383=EDGE_CURVE('',#4168,#4170,#2459,.T.) ;
#5384=EDGE_CURVE('',#4170,#4171,#2460,.T.) ;
#5385=EDGE_CURVE('',#4169,#4171,#2461,.T.) ;
#5386=EDGE_CURVE('',#4170,#4172,#2462,.T.) ;
#5387=EDGE_CURVE('',#4172,#4173,#2463,.T.) ;
#5388=EDGE_CURVE('',#4171,#4173,#2464,.T.) ;
#5389=EDGE_CURVE('',#4172,#4174,#299,.T.) ;
#5390=EDGE_CURVE('',#4174,#4175,#2465,.T.) ;
#5391=EDGE_CURVE('',#4173,#4175,#300,.T.) ;
#5392=EDGE_CURVE('',#4174,#4176,#2466,.T.) ;
#5393=EDGE_CURVE('',#4176,#4177,#2467,.T.) ;
#5394=EDGE_CURVE('',#4175,#4177,#2468,.T.) ;
#5395=EDGE_CURVE('',#4176,#4178,#2469,.T.) ;
#5396=EDGE_CURVE('',#4178,#4179,#2470,.T.) ;
#5397=EDGE_CURVE('',#4177,#4179,#2471,.T.) ;
#5398=EDGE_CURVE('',#4178,#4180,#301,.T.) ;
#5399=EDGE_CURVE('',#4180,#4181,#2472,.T.) ;
#5400=EDGE_CURVE('',#4179,#4181,#302,.T.) ;
#5401=EDGE_CURVE('',#4180,#4182,#2473,.T.) ;
#5402=EDGE_CURVE('',#4182,#4183,#2474,.T.) ;
#5403=EDGE_CURVE('',#4181,#4183,#2475,.T.) ;
#5404=EDGE_CURVE('',#4182,#4184,#2476,.T.) ;
#5405=EDGE_CURVE('',#4184,#4185,#2477,.T.) ;
#5406=EDGE_CURVE('',#4183,#4185,#2478,.T.) ;
#5407=EDGE_CURVE('',#4184,#4186,#303,.T.) ;
#5408=EDGE_CURVE('',#4186,#4187,#2479,.T.) ;
#5409=EDGE_CURVE('',#4185,#4187,#304,.T.) ;
#5410=EDGE_CURVE('',#4186,#4188,#2480,.T.) ;
#5411=EDGE_CURVE('',#4188,#4189,#2481,.T.) ;
#5412=EDGE_CURVE('',#4187,#4189,#2482,.T.) ;
#5413=EDGE_CURVE('',#4188,#4190,#2483,.T.) ;
#5414=EDGE_CURVE('',#4190,#4191,#2484,.T.) ;
#5415=EDGE_CURVE('',#4189,#4191,#2485,.T.) ;
#5416=EDGE_CURVE('',#4190,#4192,#305,.T.) ;
#5417=EDGE_CURVE('',#4192,#4193,#2486,.T.) ;
#5418=EDGE_CURVE('',#4191,#4193,#306,.T.) ;
#5419=EDGE_CURVE('',#4192,#4194,#2487,.T.) ;
#5420=EDGE_CURVE('',#4194,#4195,#2488,.T.) ;
#5421=EDGE_CURVE('',#4193,#4195,#2489,.T.) ;
#5422=EDGE_CURVE('',#4194,#4196,#2490,.T.) ;
#5423=EDGE_CURVE('',#4196,#4197,#2491,.T.) ;
#5424=EDGE_CURVE('',#4195,#4197,#2492,.T.) ;
#5425=EDGE_CURVE('',#4196,#4198,#307,.T.) ;
#5426=EDGE_CURVE('',#4198,#4199,#2493,.T.) ;
#5427=EDGE_CURVE('',#4197,#4199,#308,.T.) ;
#5428=EDGE_CURVE('',#4198,#4200,#2494,.T.) ;
#5429=EDGE_CURVE('',#4200,#4201,#2495,.T.) ;
#5430=EDGE_CURVE('',#4199,#4201,#2496,.T.) ;
#5431=EDGE_CURVE('',#4200,#4202,#2497,.T.) ;
#5432=EDGE_CURVE('',#4202,#4203,#2498,.T.) ;
#5433=EDGE_CURVE('',#4201,#4203,#2499,.T.) ;
#5434=EDGE_CURVE('',#4202,#4204,#309,.T.) ;
#5435=EDGE_CURVE('',#4204,#4205,#2500,.T.) ;
#5436=EDGE_CURVE('',#4203,#4205,#310,.T.) ;
#5437=EDGE_CURVE('',#4204,#3846,#2501,.T.) ;
#5438=EDGE_CURVE('',#4205,#3849,#2502,.T.) ;
#5439=EDGE_CURVE('',#4206,#4207,#2503,.T.) ;
#5440=EDGE_CURVE('',#4208,#4206,#745,.T.) ;
#5441=EDGE_CURVE('',#4209,#4208,#746,.T.) ;
#5442=EDGE_CURVE('',#4210,#4209,#747,.T.) ;
#5443=EDGE_CURVE('',#4211,#4210,#2504,.T.) ;
#5444=EDGE_CURVE('',#4212,#4211,#748,.T.) ;
#5445=EDGE_CURVE('',#4213,#4212,#749,.T.) ;
#5446=EDGE_CURVE('',#4207,#4213,#750,.T.) ;
#5447=EDGE_CURVE('',#4214,#4214,#751,.T.) ;
#5448=EDGE_CURVE('',#4215,#4216,#2505,.T.) ;
#5449=EDGE_CURVE('',#4217,#4215,#752,.T.) ;
#5450=EDGE_CURVE('',#4218,#4217,#753,.T.) ;
#5451=EDGE_CURVE('',#4219,#4218,#754,.T.) ;
#5452=EDGE_CURVE('',#4220,#4219,#2506,.T.) ;
#5453=EDGE_CURVE('',#4221,#4220,#755,.T.) ;
#5454=EDGE_CURVE('',#4222,#4221,#756,.T.) ;
#5455=EDGE_CURVE('',#4216,#4222,#757,.T.) ;
#5456=EDGE_CURVE('',#4223,#4224,#2507,.T.) ;
#5457=EDGE_CURVE('',#4225,#4223,#758,.T.) ;
#5458=EDGE_CURVE('',#4226,#4225,#759,.T.) ;
#5459=EDGE_CURVE('',#4227,#4226,#760,.T.) ;
#5460=EDGE_CURVE('',#4228,#4227,#2508,.T.) ;
#5461=EDGE_CURVE('',#4229,#4228,#761,.T.) ;
#5462=EDGE_CURVE('',#4230,#4229,#762,.T.) ;
#5463=EDGE_CURVE('',#4224,#4230,#763,.T.) ;
#5464=EDGE_CURVE('',#4231,#4232,#2509,.T.) ;
#5465=EDGE_CURVE('',#4233,#4231,#764,.T.) ;
#5466=EDGE_CURVE('',#4234,#4233,#765,.T.) ;
#5467=EDGE_CURVE('',#4235,#4234,#766,.T.) ;
#5468=EDGE_CURVE('',#4236,#4235,#2510,.T.) ;
#5469=EDGE_CURVE('',#4237,#4236,#767,.T.) ;
#5470=EDGE_CURVE('',#4238,#4237,#768,.T.) ;
#5471=EDGE_CURVE('',#4232,#4238,#769,.T.) ;
#5472=EDGE_CURVE('',#4239,#4240,#2511,.T.) ;
#5473=EDGE_CURVE('',#4241,#4239,#770,.T.) ;
#5474=EDGE_CURVE('',#4242,#4241,#771,.T.) ;
#5475=EDGE_CURVE('',#4243,#4242,#772,.T.) ;
#5476=EDGE_CURVE('',#4244,#4243,#2512,.T.) ;
#5477=EDGE_CURVE('',#4245,#4244,#773,.T.) ;
#5478=EDGE_CURVE('',#4246,#4245,#774,.T.) ;
#5479=EDGE_CURVE('',#4240,#4246,#775,.T.) ;
#5480=EDGE_CURVE('',#4247,#4247,#776,.T.) ;
#5481=EDGE_CURVE('',#4212,#4248,#2513,.T.) ;
#5482=EDGE_CURVE('',#4249,#4248,#777,.T.) ;
#5483=EDGE_CURVE('',#4213,#4249,#2514,.T.) ;
#5484=EDGE_CURVE('',#4250,#4249,#778,.T.) ;
#5485=EDGE_CURVE('',#4207,#4250,#2515,.T.) ;
#5486=EDGE_CURVE('',#4206,#4251,#2516,.T.) ;
#5487=EDGE_CURVE('',#4251,#4250,#2517,.T.) ;
#5488=EDGE_CURVE('',#4252,#4251,#779,.T.) ;
#5489=EDGE_CURVE('',#4208,#4252,#2518,.T.) ;
#5490=EDGE_CURVE('',#4253,#4252,#780,.T.) ;
#5491=EDGE_CURVE('',#4209,#4253,#2519,.T.) ;
#5492=EDGE_CURVE('',#4254,#4253,#781,.T.) ;
#5493=EDGE_CURVE('',#4210,#4254,#2520,.T.) ;
#5494=EDGE_CURVE('',#4255,#4254,#2521,.T.) ;
#5495=EDGE_CURVE('',#4211,#4255,#2522,.T.) ;
#5496=EDGE_CURVE('',#4248,#4255,#782,.T.) ;
#5497=EDGE_CURVE('',#4256,#4256,#783,.T.) ;
#5498=EDGE_CURVE('',#4256,#4214,#2523,.T.) ;
#5499=EDGE_CURVE('',#4221,#4257,#2524,.T.) ;
#5500=EDGE_CURVE('',#4258,#4257,#784,.T.) ;
#5501=EDGE_CURVE('',#4222,#4258,#2525,.T.) ;
#5502=EDGE_CURVE('',#4259,#4258,#785,.T.) ;
#5503=EDGE_CURVE('',#4216,#4259,#2526,.T.) ;
#5504=EDGE_CURVE('',#4215,#4260,#2527,.T.) ;
#5505=EDGE_CURVE('',#4260,#4259,#2528,.T.) ;
#5506=EDGE_CURVE('',#4261,#4260,#786,.T.) ;
#5507=EDGE_CURVE('',#4217,#4261,#2529,.T.) ;
#5508=EDGE_CURVE('',#4262,#4261,#787,.T.) ;
#5509=EDGE_CURVE('',#4218,#4262,#2530,.T.) ;
#5510=EDGE_CURVE('',#4263,#4262,#788,.T.) ;
#5511=EDGE_CURVE('',#4219,#4263,#2531,.T.) ;
#5512=EDGE_CURVE('',#4264,#4263,#2532,.T.) ;
#5513=EDGE_CURVE('',#4220,#4264,#2533,.T.) ;
#5514=EDGE_CURVE('',#4257,#4264,#789,.T.) ;
#5515=EDGE_CURVE('',#4229,#4265,#2534,.T.) ;
#5516=EDGE_CURVE('',#4266,#4265,#790,.T.) ;
#5517=EDGE_CURVE('',#4230,#4266,#2535,.T.) ;
#5518=EDGE_CURVE('',#4267,#4266,#791,.T.) ;
#5519=EDGE_CURVE('',#4224,#4267,#2536,.T.) ;
#5520=EDGE_CURVE('',#4223,#4268,#2537,.T.) ;
#5521=EDGE_CURVE('',#4268,#4267,#2538,.T.) ;
#5522=EDGE_CURVE('',#4269,#4268,#792,.T.) ;
#5523=EDGE_CURVE('',#4225,#4269,#2539,.T.) ;
#5524=EDGE_CURVE('',#4270,#4269,#793,.T.) ;
#5525=EDGE_CURVE('',#4226,#4270,#2540,.T.) ;
#5526=EDGE_CURVE('',#4271,#4270,#794,.T.) ;
#5527=EDGE_CURVE('',#4227,#4271,#2541,.T.) ;
#5528=EDGE_CURVE('',#4272,#4271,#2542,.T.) ;
#5529=EDGE_CURVE('',#4228,#4272,#2543,.T.) ;
#5530=EDGE_CURVE('',#4265,#4272,#795,.T.) ;
#5531=EDGE_CURVE('',#4237,#4273,#2544,.T.) ;
#5532=EDGE_CURVE('',#4274,#4273,#796,.T.) ;
#5533=EDGE_CURVE('',#4238,#4274,#2545,.T.) ;
#5534=EDGE_CURVE('',#4275,#4274,#797,.T.) ;
#5535=EDGE_CURVE('',#4232,#4275,#2546,.T.) ;
#5536=EDGE_CURVE('',#4231,#4276,#2547,.T.) ;
#5537=EDGE_CURVE('',#4276,#4275,#2548,.T.) ;
#5538=EDGE_CURVE('',#4277,#4276,#798,.T.) ;
#5539=EDGE_CURVE('',#4233,#4277,#2549,.T.) ;
#5540=EDGE_CURVE('',#4278,#4277,#799,.T.) ;
#5541=EDGE_CURVE('',#4234,#4278,#2550,.T.) ;
#5542=EDGE_CURVE('',#4279,#4278,#800,.T.) ;
#5543=EDGE_CURVE('',#4235,#4279,#2551,.T.) ;
#5544=EDGE_CURVE('',#4280,#4279,#2552,.T.) ;
#5545=EDGE_CURVE('',#4236,#4280,#2553,.T.) ;
#5546=EDGE_CURVE('',#4273,#4280,#801,.T.) ;
#5547=EDGE_CURVE('',#4245,#4281,#2554,.T.) ;
#5548=EDGE_CURVE('',#4282,#4281,#802,.T.) ;
#5549=EDGE_CURVE('',#4246,#4282,#2555,.T.) ;
#5550=EDGE_CURVE('',#4283,#4282,#803,.T.) ;
#5551=EDGE_CURVE('',#4240,#4283,#2556,.T.) ;
#5552=EDGE_CURVE('',#4239,#4284,#2557,.T.) ;
#5553=EDGE_CURVE('',#4284,#4283,#2558,.T.) ;
#5554=EDGE_CURVE('',#4285,#4284,#804,.T.) ;
#5555=EDGE_CURVE('',#4241,#4285,#2559,.T.) ;
#5556=EDGE_CURVE('',#4286,#4285,#805,.T.) ;
#5557=EDGE_CURVE('',#4242,#4286,#2560,.T.) ;
#5558=EDGE_CURVE('',#4287,#4286,#806,.T.) ;
#5559=EDGE_CURVE('',#4243,#4287,#2561,.T.) ;
#5560=EDGE_CURVE('',#4288,#4287,#2562,.T.) ;
#5561=EDGE_CURVE('',#4244,#4288,#2563,.T.) ;
#5562=EDGE_CURVE('',#4281,#4288,#807,.T.) ;
#5563=EDGE_CURVE('',#4247,#4289,#2564,.T.) ;
#5564=EDGE_CURVE('',#4289,#4289,#808,.T.) ;
#5565=EDGE_CURVE('',#4290,#4290,#809,.T.) ;
#5566=EDGE_CURVE('',#4290,#4291,#2565,.T.) ;
#5567=EDGE_CURVE('',#4291,#4291,#810,.T.) ;
#6782=ORIENTED_EDGE('',*,*,#4899,.T.) ;
#6783=ORIENTED_EDGE('',*,*,#4900,.T.) ;
#6784=ORIENTED_EDGE('',*,*,#4901,.F.) ;
#6785=ORIENTED_EDGE('',*,*,#4902,.F.) ;
#6786=ORIENTED_EDGE('',*,*,#4903,.T.) ;
#6787=ORIENTED_EDGE('',*,*,#4904,.T.) ;
#6788=ORIENTED_EDGE('',*,*,#4905,.F.) ;
#6789=ORIENTED_EDGE('',*,*,#4900,.F.) ;
#6790=ORIENTED_EDGE('',*,*,#4906,.T.) ;
#6791=ORIENTED_EDGE('',*,*,#4907,.T.) ;
#6792=ORIENTED_EDGE('',*,*,#4908,.F.) ;
#6793=ORIENTED_EDGE('',*,*,#4904,.F.) ;
#6794=ORIENTED_EDGE('',*,*,#4909,.T.) ;
#6795=ORIENTED_EDGE('',*,*,#4910,.T.) ;
#6796=ORIENTED_EDGE('',*,*,#4911,.F.) ;
#6797=ORIENTED_EDGE('',*,*,#4907,.F.) ;
#6798=ORIENTED_EDGE('',*,*,#4912,.T.) ;
#6799=ORIENTED_EDGE('',*,*,#4913,.T.) ;
#6800=ORIENTED_EDGE('',*,*,#4914,.F.) ;
#6801=ORIENTED_EDGE('',*,*,#4910,.F.) ;
#6802=ORIENTED_EDGE('',*,*,#4915,.T.) ;
#6803=ORIENTED_EDGE('',*,*,#4916,.T.) ;
#6804=ORIENTED_EDGE('',*,*,#4917,.F.) ;
#6805=ORIENTED_EDGE('',*,*,#4913,.F.) ;
#6806=ORIENTED_EDGE('',*,*,#4918,.T.) ;
#6807=ORIENTED_EDGE('',*,*,#4919,.T.) ;
#6808=ORIENTED_EDGE('',*,*,#4920,.F.) ;
#6809=ORIENTED_EDGE('',*,*,#4916,.F.) ;
#6810=ORIENTED_EDGE('',*,*,#4921,.T.) ;
#6811=ORIENTED_EDGE('',*,*,#4922,.T.) ;
#6812=ORIENTED_EDGE('',*,*,#4923,.F.) ;
#6813=ORIENTED_EDGE('',*,*,#4919,.F.) ;
#6814=ORIENTED_EDGE('',*,*,#4924,.T.) ;
#6815=ORIENTED_EDGE('',*,*,#4925,.T.) ;
#6816=ORIENTED_EDGE('',*,*,#4926,.F.) ;
#6817=ORIENTED_EDGE('',*,*,#4922,.F.) ;
#6818=ORIENTED_EDGE('',*,*,#4927,.T.) ;
#6819=ORIENTED_EDGE('',*,*,#4928,.T.) ;
#6820=ORIENTED_EDGE('',*,*,#4929,.F.) ;
#6821=ORIENTED_EDGE('',*,*,#4925,.F.) ;
#6822=ORIENTED_EDGE('',*,*,#4930,.T.) ;
#6823=ORIENTED_EDGE('',*,*,#4931,.T.) ;
#6824=ORIENTED_EDGE('',*,*,#4932,.F.) ;
#6825=ORIENTED_EDGE('',*,*,#4928,.F.) ;
#6826=ORIENTED_EDGE('',*,*,#4933,.T.) ;
#6827=ORIENTED_EDGE('',*,*,#4934,.T.) ;
#6828=ORIENTED_EDGE('',*,*,#4935,.F.) ;
#6829=ORIENTED_EDGE('',*,*,#4931,.F.) ;
#6830=ORIENTED_EDGE('',*,*,#4936,.T.) ;
#6831=ORIENTED_EDGE('',*,*,#4937,.T.) ;
#6832=ORIENTED_EDGE('',*,*,#4938,.F.) ;
#6833=ORIENTED_EDGE('',*,*,#4934,.F.) ;
#6834=ORIENTED_EDGE('',*,*,#4939,.T.) ;
#6835=ORIENTED_EDGE('',*,*,#4940,.T.) ;
#6836=ORIENTED_EDGE('',*,*,#4941,.F.) ;
#6837=ORIENTED_EDGE('',*,*,#4937,.F.) ;
#6838=ORIENTED_EDGE('',*,*,#4942,.T.) ;
#6839=ORIENTED_EDGE('',*,*,#4943,.T.) ;
#6840=ORIENTED_EDGE('',*,*,#4944,.F.) ;
#6841=ORIENTED_EDGE('',*,*,#4940,.F.) ;
#6842=ORIENTED_EDGE('',*,*,#4945,.T.) ;
#6843=ORIENTED_EDGE('',*,*,#4946,.T.) ;
#6844=ORIENTED_EDGE('',*,*,#4947,.F.) ;
#6845=ORIENTED_EDGE('',*,*,#4943,.F.) ;
#6846=ORIENTED_EDGE('',*,*,#4948,.T.) ;
#6847=ORIENTED_EDGE('',*,*,#4949,.T.) ;
#6848=ORIENTED_EDGE('',*,*,#4950,.F.) ;
#6849=ORIENTED_EDGE('',*,*,#4946,.F.) ;
#6850=ORIENTED_EDGE('',*,*,#4951,.T.) ;
#6851=ORIENTED_EDGE('',*,*,#4952,.T.) ;
#6852=ORIENTED_EDGE('',*,*,#4953,.F.) ;
#6853=ORIENTED_EDGE('',*,*,#4949,.F.) ;
#6854=ORIENTED_EDGE('',*,*,#4954,.T.) ;
#6855=ORIENTED_EDGE('',*,*,#4955,.T.) ;
#6856=ORIENTED_EDGE('',*,*,#4956,.F.) ;
#6857=ORIENTED_EDGE('',*,*,#4952,.F.) ;
#6858=ORIENTED_EDGE('',*,*,#4957,.T.) ;
#6859=ORIENTED_EDGE('',*,*,#4958,.T.) ;
#6860=ORIENTED_EDGE('',*,*,#4959,.F.) ;
#6861=ORIENTED_EDGE('',*,*,#4955,.F.) ;
#6862=ORIENTED_EDGE('',*,*,#4960,.T.) ;
#6863=ORIENTED_EDGE('',*,*,#4961,.T.) ;
#6864=ORIENTED_EDGE('',*,*,#4962,.F.) ;
#6865=ORIENTED_EDGE('',*,*,#4958,.F.) ;
#6866=ORIENTED_EDGE('',*,*,#4963,.T.) ;
#6867=ORIENTED_EDGE('',*,*,#4964,.T.) ;
#6868=ORIENTED_EDGE('',*,*,#4965,.F.) ;
#6869=ORIENTED_EDGE('',*,*,#4961,.F.) ;
#6870=ORIENTED_EDGE('',*,*,#4966,.T.) ;
#6871=ORIENTED_EDGE('',*,*,#4967,.T.) ;
#6872=ORIENTED_EDGE('',*,*,#4968,.F.) ;
#6873=ORIENTED_EDGE('',*,*,#4964,.F.) ;
#6874=ORIENTED_EDGE('',*,*,#4969,.T.) ;
#6875=ORIENTED_EDGE('',*,*,#4970,.T.) ;
#6876=ORIENTED_EDGE('',*,*,#4971,.F.) ;
#6877=ORIENTED_EDGE('',*,*,#4967,.F.) ;
#6878=ORIENTED_EDGE('',*,*,#4972,.T.) ;
#6879=ORIENTED_EDGE('',*,*,#4973,.T.) ;
#6880=ORIENTED_EDGE('',*,*,#4974,.F.) ;
#6881=ORIENTED_EDGE('',*,*,#4970,.F.) ;
#6882=ORIENTED_EDGE('',*,*,#4975,.T.) ;
#6883=ORIENTED_EDGE('',*,*,#4976,.T.) ;
#6884=ORIENTED_EDGE('',*,*,#4977,.F.) ;
#6885=ORIENTED_EDGE('',*,*,#4973,.F.) ;
#6886=ORIENTED_EDGE('',*,*,#4978,.T.) ;
#6887=ORIENTED_EDGE('',*,*,#4979,.T.) ;
#6888=ORIENTED_EDGE('',*,*,#4980,.F.) ;
#6889=ORIENTED_EDGE('',*,*,#4976,.F.) ;
#6890=ORIENTED_EDGE('',*,*,#4981,.T.) ;
#6891=ORIENTED_EDGE('',*,*,#4982,.T.) ;
#6892=ORIENTED_EDGE('',*,*,#4983,.F.) ;
#6893=ORIENTED_EDGE('',*,*,#4979,.F.) ;
#6894=ORIENTED_EDGE('',*,*,#4984,.T.) ;
#6895=ORIENTED_EDGE('',*,*,#4985,.T.) ;
#6896=ORIENTED_EDGE('',*,*,#4986,.F.) ;
#6897=ORIENTED_EDGE('',*,*,#4982,.F.) ;
#6898=ORIENTED_EDGE('',*,*,#4987,.T.) ;
#6899=ORIENTED_EDGE('',*,*,#4988,.T.) ;
#6900=ORIENTED_EDGE('',*,*,#4989,.F.) ;
#6901=ORIENTED_EDGE('',*,*,#4985,.F.) ;
#6902=ORIENTED_EDGE('',*,*,#4990,.T.) ;
#6903=ORIENTED_EDGE('',*,*,#4991,.T.) ;
#6904=ORIENTED_EDGE('',*,*,#4992,.F.) ;
#6905=ORIENTED_EDGE('',*,*,#4988,.F.) ;
#6906=ORIENTED_EDGE('',*,*,#4993,.T.) ;
#6907=ORIENTED_EDGE('',*,*,#4994,.T.) ;
#6908=ORIENTED_EDGE('',*,*,#4995,.F.) ;
#6909=ORIENTED_EDGE('',*,*,#4991,.F.) ;
#6910=ORIENTED_EDGE('',*,*,#4996,.T.) ;
#6911=ORIENTED_EDGE('',*,*,#4997,.T.) ;
#6912=ORIENTED_EDGE('',*,*,#4998,.F.) ;
#6913=ORIENTED_EDGE('',*,*,#4994,.F.) ;
#6914=ORIENTED_EDGE('',*,*,#4999,.T.) ;
#6915=ORIENTED_EDGE('',*,*,#5000,.T.) ;
#6916=ORIENTED_EDGE('',*,*,#5001,.F.) ;
#6917=ORIENTED_EDGE('',*,*,#4997,.F.) ;
#6918=ORIENTED_EDGE('',*,*,#5002,.T.) ;
#6919=ORIENTED_EDGE('',*,*,#5003,.T.) ;
#6920=ORIENTED_EDGE('',*,*,#5004,.F.) ;
#6921=ORIENTED_EDGE('',*,*,#5000,.F.) ;
#6922=ORIENTED_EDGE('',*,*,#5005,.T.) ;
#6923=ORIENTED_EDGE('',*,*,#5006,.T.) ;
#6924=ORIENTED_EDGE('',*,*,#5007,.F.) ;
#6925=ORIENTED_EDGE('',*,*,#5003,.F.) ;
#6926=ORIENTED_EDGE('',*,*,#5008,.T.) ;
#6927=ORIENTED_EDGE('',*,*,#5009,.T.) ;
#6928=ORIENTED_EDGE('',*,*,#5010,.F.) ;
#6929=ORIENTED_EDGE('',*,*,#5006,.F.) ;
#6930=ORIENTED_EDGE('',*,*,#5011,.T.) ;
#6931=ORIENTED_EDGE('',*,*,#5012,.T.) ;
#6932=ORIENTED_EDGE('',*,*,#5013,.F.) ;
#6933=ORIENTED_EDGE('',*,*,#5009,.F.) ;
#6934=ORIENTED_EDGE('',*,*,#5014,.T.) ;
#6935=ORIENTED_EDGE('',*,*,#5015,.T.) ;
#6936=ORIENTED_EDGE('',*,*,#5016,.F.) ;
#6937=ORIENTED_EDGE('',*,*,#5012,.F.) ;
#6938=ORIENTED_EDGE('',*,*,#5017,.T.) ;
#6939=ORIENTED_EDGE('',*,*,#5018,.T.) ;
#6940=ORIENTED_EDGE('',*,*,#5019,.F.) ;
#6941=ORIENTED_EDGE('',*,*,#5015,.F.) ;
#6942=ORIENTED_EDGE('',*,*,#5020,.T.) ;
#6943=ORIENTED_EDGE('',*,*,#5021,.T.) ;
#6944=ORIENTED_EDGE('',*,*,#5022,.F.) ;
#6945=ORIENTED_EDGE('',*,*,#5018,.F.) ;
#6946=ORIENTED_EDGE('',*,*,#5023,.T.) ;
#6947=ORIENTED_EDGE('',*,*,#5024,.T.) ;
#6948=ORIENTED_EDGE('',*,*,#5025,.F.) ;
#6949=ORIENTED_EDGE('',*,*,#5021,.F.) ;
#6950=ORIENTED_EDGE('',*,*,#5026,.T.) ;
#6951=ORIENTED_EDGE('',*,*,#5027,.T.) ;
#6952=ORIENTED_EDGE('',*,*,#5028,.F.) ;
#6953=ORIENTED_EDGE('',*,*,#5024,.F.) ;
#6954=ORIENTED_EDGE('',*,*,#5029,.T.) ;
#6955=ORIENTED_EDGE('',*,*,#5030,.T.) ;
#6956=ORIENTED_EDGE('',*,*,#5031,.F.) ;
#6957=ORIENTED_EDGE('',*,*,#5027,.F.) ;
#6958=ORIENTED_EDGE('',*,*,#5032,.T.) ;
#6959=ORIENTED_EDGE('',*,*,#5033,.T.) ;
#6960=ORIENTED_EDGE('',*,*,#5034,.F.) ;
#6961=ORIENTED_EDGE('',*,*,#5030,.F.) ;
#6962=ORIENTED_EDGE('',*,*,#5035,.T.) ;
#6963=ORIENTED_EDGE('',*,*,#5036,.T.) ;
#6964=ORIENTED_EDGE('',*,*,#5037,.F.) ;
#6965=ORIENTED_EDGE('',*,*,#5033,.F.) ;
#6966=ORIENTED_EDGE('',*,*,#5038,.T.) ;
#6967=ORIENTED_EDGE('',*,*,#5039,.T.) ;
#6968=ORIENTED_EDGE('',*,*,#5040,.F.) ;
#6969=ORIENTED_EDGE('',*,*,#5036,.F.) ;
#6970=ORIENTED_EDGE('',*,*,#5041,.T.) ;
#6971=ORIENTED_EDGE('',*,*,#5042,.T.) ;
#6972=ORIENTED_EDGE('',*,*,#5043,.F.) ;
#6973=ORIENTED_EDGE('',*,*,#5039,.F.) ;
#6974=ORIENTED_EDGE('',*,*,#5044,.T.) ;
#6975=ORIENTED_EDGE('',*,*,#5045,.T.) ;
#6976=ORIENTED_EDGE('',*,*,#5046,.F.) ;
#6977=ORIENTED_EDGE('',*,*,#5042,.F.) ;
#6978=ORIENTED_EDGE('',*,*,#5047,.T.) ;
#6979=ORIENTED_EDGE('',*,*,#5048,.T.) ;
#6980=ORIENTED_EDGE('',*,*,#5049,.F.) ;
#6981=ORIENTED_EDGE('',*,*,#5045,.F.) ;
#6982=ORIENTED_EDGE('',*,*,#5050,.T.) ;
#6983=ORIENTED_EDGE('',*,*,#5051,.T.) ;
#6984=ORIENTED_EDGE('',*,*,#5052,.F.) ;
#6985=ORIENTED_EDGE('',*,*,#5048,.F.) ;
#6986=ORIENTED_EDGE('',*,*,#5053,.T.) ;
#6987=ORIENTED_EDGE('',*,*,#5054,.T.) ;
#6988=ORIENTED_EDGE('',*,*,#5055,.F.) ;
#6989=ORIENTED_EDGE('',*,*,#5051,.F.) ;
#6990=ORIENTED_EDGE('',*,*,#5056,.T.) ;
#6991=ORIENTED_EDGE('',*,*,#5057,.T.) ;
#6992=ORIENTED_EDGE('',*,*,#5058,.F.) ;
#6993=ORIENTED_EDGE('',*,*,#5054,.F.) ;
#6994=ORIENTED_EDGE('',*,*,#5059,.T.) ;
#6995=ORIENTED_EDGE('',*,*,#5060,.T.) ;
#6996=ORIENTED_EDGE('',*,*,#5061,.F.) ;
#6997=ORIENTED_EDGE('',*,*,#5057,.F.) ;
#6998=ORIENTED_EDGE('',*,*,#5062,.T.) ;
#6999=ORIENTED_EDGE('',*,*,#5063,.T.) ;
#7000=ORIENTED_EDGE('',*,*,#5064,.F.) ;
#7001=ORIENTED_EDGE('',*,*,#5060,.F.) ;
#7002=ORIENTED_EDGE('',*,*,#5065,.T.) ;
#7003=ORIENTED_EDGE('',*,*,#5066,.T.) ;
#7004=ORIENTED_EDGE('',*,*,#5067,.F.) ;
#7005=ORIENTED_EDGE('',*,*,#5063,.F.) ;
#7006=ORIENTED_EDGE('',*,*,#5068,.T.) ;
#7007=ORIENTED_EDGE('',*,*,#5069,.T.) ;
#7008=ORIENTED_EDGE('',*,*,#5070,.F.) ;
#7009=ORIENTED_EDGE('',*,*,#5066,.F.) ;
#7010=ORIENTED_EDGE('',*,*,#5071,.T.) ;
#7011=ORIENTED_EDGE('',*,*,#5072,.T.) ;
#7012=ORIENTED_EDGE('',*,*,#5073,.F.) ;
#7013=ORIENTED_EDGE('',*,*,#5069,.F.) ;
#7014=ORIENTED_EDGE('',*,*,#5074,.T.) ;
#7015=ORIENTED_EDGE('',*,*,#5075,.T.) ;
#7016=ORIENTED_EDGE('',*,*,#5076,.F.) ;
#7017=ORIENTED_EDGE('',*,*,#5072,.F.) ;
#7018=ORIENTED_EDGE('',*,*,#5077,.T.) ;
#7019=ORIENTED_EDGE('',*,*,#5078,.T.) ;
#7020=ORIENTED_EDGE('',*,*,#5079,.F.) ;
#7021=ORIENTED_EDGE('',*,*,#5075,.F.) ;
#7022=ORIENTED_EDGE('',*,*,#5080,.T.) ;
#7023=ORIENTED_EDGE('',*,*,#5081,.T.) ;
#7024=ORIENTED_EDGE('',*,*,#5082,.F.) ;
#7025=ORIENTED_EDGE('',*,*,#5078,.F.) ;
#7026=ORIENTED_EDGE('',*,*,#5083,.T.) ;
#7027=ORIENTED_EDGE('',*,*,#5084,.T.) ;
#7028=ORIENTED_EDGE('',*,*,#5085,.F.) ;
#7029=ORIENTED_EDGE('',*,*,#5081,.F.) ;
#7030=ORIENTED_EDGE('',*,*,#5086,.T.) ;
#7031=ORIENTED_EDGE('',*,*,#5087,.T.) ;
#7032=ORIENTED_EDGE('',*,*,#5088,.F.) ;
#7033=ORIENTED_EDGE('',*,*,#5084,.F.) ;
#7034=ORIENTED_EDGE('',*,*,#5089,.T.) ;
#7035=ORIENTED_EDGE('',*,*,#5090,.T.) ;
#7036=ORIENTED_EDGE('',*,*,#5091,.F.) ;
#7037=ORIENTED_EDGE('',*,*,#5087,.F.) ;
#7038=ORIENTED_EDGE('',*,*,#5092,.T.) ;
#7039=ORIENTED_EDGE('',*,*,#5093,.T.) ;
#7040=ORIENTED_EDGE('',*,*,#5094,.F.) ;
#7041=ORIENTED_EDGE('',*,*,#5090,.F.) ;
#7042=ORIENTED_EDGE('',*,*,#5095,.T.) ;
#7043=ORIENTED_EDGE('',*,*,#5096,.T.) ;
#7044=ORIENTED_EDGE('',*,*,#5097,.F.) ;
#7045=ORIENTED_EDGE('',*,*,#5093,.F.) ;
#7046=ORIENTED_EDGE('',*,*,#5098,.T.) ;
#7047=ORIENTED_EDGE('',*,*,#5099,.T.) ;
#7048=ORIENTED_EDGE('',*,*,#5100,.F.) ;
#7049=ORIENTED_EDGE('',*,*,#5096,.F.) ;
#7050=ORIENTED_EDGE('',*,*,#5101,.T.) ;
#7051=ORIENTED_EDGE('',*,*,#5102,.T.) ;
#7052=ORIENTED_EDGE('',*,*,#5103,.F.) ;
#7053=ORIENTED_EDGE('',*,*,#5099,.F.) ;
#7054=ORIENTED_EDGE('',*,*,#5104,.T.) ;
#7055=ORIENTED_EDGE('',*,*,#5105,.T.) ;
#7056=ORIENTED_EDGE('',*,*,#5106,.F.) ;
#7057=ORIENTED_EDGE('',*,*,#5102,.F.) ;
#7058=ORIENTED_EDGE('',*,*,#5107,.T.) ;
#7059=ORIENTED_EDGE('',*,*,#5108,.T.) ;
#7060=ORIENTED_EDGE('',*,*,#5109,.F.) ;
#7061=ORIENTED_EDGE('',*,*,#5105,.F.) ;
#7062=ORIENTED_EDGE('',*,*,#5110,.T.) ;
#7063=ORIENTED_EDGE('',*,*,#5111,.T.) ;
#7064=ORIENTED_EDGE('',*,*,#5112,.F.) ;
#7065=ORIENTED_EDGE('',*,*,#5108,.F.) ;
#7066=ORIENTED_EDGE('',*,*,#5113,.T.) ;
#7067=ORIENTED_EDGE('',*,*,#5114,.T.) ;
#7068=ORIENTED_EDGE('',*,*,#5115,.F.) ;
#7069=ORIENTED_EDGE('',*,*,#5111,.F.) ;
#7070=ORIENTED_EDGE('',*,*,#5116,.T.) ;
#7071=ORIENTED_EDGE('',*,*,#5117,.T.) ;
#7072=ORIENTED_EDGE('',*,*,#5118,.F.) ;
#7073=ORIENTED_EDGE('',*,*,#5114,.F.) ;
#7074=ORIENTED_EDGE('',*,*,#5119,.T.) ;
#7075=ORIENTED_EDGE('',*,*,#5120,.T.) ;
#7076=ORIENTED_EDGE('',*,*,#5121,.F.) ;
#7077=ORIENTED_EDGE('',*,*,#5117,.F.) ;
#7078=ORIENTED_EDGE('',*,*,#5122,.T.) ;
#7079=ORIENTED_EDGE('',*,*,#5123,.T.) ;
#7080=ORIENTED_EDGE('',*,*,#5124,.F.) ;
#7081=ORIENTED_EDGE('',*,*,#5120,.F.) ;
#7082=ORIENTED_EDGE('',*,*,#5125,.T.) ;
#7083=ORIENTED_EDGE('',*,*,#5126,.T.) ;
#7084=ORIENTED_EDGE('',*,*,#5127,.F.) ;
#7085=ORIENTED_EDGE('',*,*,#5123,.F.) ;
#7086=ORIENTED_EDGE('',*,*,#5128,.T.) ;
#7087=ORIENTED_EDGE('',*,*,#5129,.T.) ;
#7088=ORIENTED_EDGE('',*,*,#5130,.F.) ;
#7089=ORIENTED_EDGE('',*,*,#5126,.F.) ;
#7090=ORIENTED_EDGE('',*,*,#5131,.T.) ;
#7091=ORIENTED_EDGE('',*,*,#5132,.T.) ;
#7092=ORIENTED_EDGE('',*,*,#5133,.F.) ;
#7093=ORIENTED_EDGE('',*,*,#5129,.F.) ;
#7094=ORIENTED_EDGE('',*,*,#5134,.T.) ;
#7095=ORIENTED_EDGE('',*,*,#5135,.T.) ;
#7096=ORIENTED_EDGE('',*,*,#5136,.F.) ;
#7097=ORIENTED_EDGE('',*,*,#5132,.F.) ;
#7098=ORIENTED_EDGE('',*,*,#5137,.T.) ;
#7099=ORIENTED_EDGE('',*,*,#5138,.T.) ;
#7100=ORIENTED_EDGE('',*,*,#5139,.F.) ;
#7101=ORIENTED_EDGE('',*,*,#5135,.F.) ;
#7102=ORIENTED_EDGE('',*,*,#5140,.T.) ;
#7103=ORIENTED_EDGE('',*,*,#5141,.T.) ;
#7104=ORIENTED_EDGE('',*,*,#5142,.F.) ;
#7105=ORIENTED_EDGE('',*,*,#5138,.F.) ;
#7106=ORIENTED_EDGE('',*,*,#5143,.T.) ;
#7107=ORIENTED_EDGE('',*,*,#5144,.T.) ;
#7108=ORIENTED_EDGE('',*,*,#5145,.F.) ;
#7109=ORIENTED_EDGE('',*,*,#5141,.F.) ;
#7110=ORIENTED_EDGE('',*,*,#5146,.T.) ;
#7111=ORIENTED_EDGE('',*,*,#5147,.T.) ;
#7112=ORIENTED_EDGE('',*,*,#5148,.F.) ;
#7113=ORIENTED_EDGE('',*,*,#5144,.F.) ;
#7114=ORIENTED_EDGE('',*,*,#5149,.T.) ;
#7115=ORIENTED_EDGE('',*,*,#5150,.T.) ;
#7116=ORIENTED_EDGE('',*,*,#5151,.F.) ;
#7117=ORIENTED_EDGE('',*,*,#5147,.F.) ;
#7118=ORIENTED_EDGE('',*,*,#5152,.T.) ;
#7119=ORIENTED_EDGE('',*,*,#5153,.T.) ;
#7120=ORIENTED_EDGE('',*,*,#5154,.F.) ;
#7121=ORIENTED_EDGE('',*,*,#5150,.F.) ;
#7122=ORIENTED_EDGE('',*,*,#5155,.T.) ;
#7123=ORIENTED_EDGE('',*,*,#5156,.T.) ;
#7124=ORIENTED_EDGE('',*,*,#5157,.F.) ;
#7125=ORIENTED_EDGE('',*,*,#5153,.F.) ;
#7126=ORIENTED_EDGE('',*,*,#5158,.T.) ;
#7127=ORIENTED_EDGE('',*,*,#5159,.T.) ;
#7128=ORIENTED_EDGE('',*,*,#5160,.F.) ;
#7129=ORIENTED_EDGE('',*,*,#5156,.F.) ;
#7130=ORIENTED_EDGE('',*,*,#5161,.T.) ;
#7131=ORIENTED_EDGE('',*,*,#5162,.T.) ;
#7132=ORIENTED_EDGE('',*,*,#5163,.F.) ;
#7133=ORIENTED_EDGE('',*,*,#5159,.F.) ;
#7134=ORIENTED_EDGE('',*,*,#5164,.T.) ;
#7135=ORIENTED_EDGE('',*,*,#5165,.T.) ;
#7136=ORIENTED_EDGE('',*,*,#5166,.F.) ;
#7137=ORIENTED_EDGE('',*,*,#5162,.F.) ;
#7138=ORIENTED_EDGE('',*,*,#5167,.T.) ;
#7139=ORIENTED_EDGE('',*,*,#5168,.T.) ;
#7140=ORIENTED_EDGE('',*,*,#5169,.F.) ;
#7141=ORIENTED_EDGE('',*,*,#5165,.F.) ;
#7142=ORIENTED_EDGE('',*,*,#5170,.T.) ;
#7143=ORIENTED_EDGE('',*,*,#5171,.T.) ;
#7144=ORIENTED_EDGE('',*,*,#5172,.F.) ;
#7145=ORIENTED_EDGE('',*,*,#5168,.F.) ;
#7146=ORIENTED_EDGE('',*,*,#5173,.T.) ;
#7147=ORIENTED_EDGE('',*,*,#5174,.T.) ;
#7148=ORIENTED_EDGE('',*,*,#5175,.F.) ;
#7149=ORIENTED_EDGE('',*,*,#5171,.F.) ;
#7150=ORIENTED_EDGE('',*,*,#5176,.T.) ;
#7151=ORIENTED_EDGE('',*,*,#5177,.T.) ;
#7152=ORIENTED_EDGE('',*,*,#5178,.F.) ;
#7153=ORIENTED_EDGE('',*,*,#5174,.F.) ;
#7154=ORIENTED_EDGE('',*,*,#5179,.T.) ;
#7155=ORIENTED_EDGE('',*,*,#5180,.T.) ;
#7156=ORIENTED_EDGE('',*,*,#5181,.F.) ;
#7157=ORIENTED_EDGE('',*,*,#5177,.F.) ;
#7158=ORIENTED_EDGE('',*,*,#5182,.T.) ;
#7159=ORIENTED_EDGE('',*,*,#5183,.T.) ;
#7160=ORIENTED_EDGE('',*,*,#5184,.F.) ;
#7161=ORIENTED_EDGE('',*,*,#5180,.F.) ;
#7162=ORIENTED_EDGE('',*,*,#5185,.T.) ;
#7163=ORIENTED_EDGE('',*,*,#5186,.T.) ;
#7164=ORIENTED_EDGE('',*,*,#5187,.F.) ;
#7165=ORIENTED_EDGE('',*,*,#5183,.F.) ;
#7166=ORIENTED_EDGE('',*,*,#5188,.T.) ;
#7167=ORIENTED_EDGE('',*,*,#5189,.T.) ;
#7168=ORIENTED_EDGE('',*,*,#5190,.F.) ;
#7169=ORIENTED_EDGE('',*,*,#5186,.F.) ;
#7170=ORIENTED_EDGE('',*,*,#5191,.T.) ;
#7171=ORIENTED_EDGE('',*,*,#5192,.T.) ;
#7172=ORIENTED_EDGE('',*,*,#5193,.F.) ;
#7173=ORIENTED_EDGE('',*,*,#5189,.F.) ;
#7174=ORIENTED_EDGE('',*,*,#5194,.T.) ;
#7175=ORIENTED_EDGE('',*,*,#5195,.T.) ;
#7176=ORIENTED_EDGE('',*,*,#5196,.F.) ;
#7177=ORIENTED_EDGE('',*,*,#5192,.F.) ;
#7178=ORIENTED_EDGE('',*,*,#5197,.T.) ;
#7179=ORIENTED_EDGE('',*,*,#5198,.T.) ;
#7180=ORIENTED_EDGE('',*,*,#5199,.F.) ;
#7181=ORIENTED_EDGE('',*,*,#5195,.F.) ;
#7182=ORIENTED_EDGE('',*,*,#5200,.T.) ;
#7183=ORIENTED_EDGE('',*,*,#5201,.T.) ;
#7184=ORIENTED_EDGE('',*,*,#5202,.F.) ;
#7185=ORIENTED_EDGE('',*,*,#5198,.F.) ;
#7186=ORIENTED_EDGE('',*,*,#5203,.T.) ;
#7187=ORIENTED_EDGE('',*,*,#5204,.T.) ;
#7188=ORIENTED_EDGE('',*,*,#5205,.F.) ;
#7189=ORIENTED_EDGE('',*,*,#5201,.F.) ;
#7190=ORIENTED_EDGE('',*,*,#5206,.T.) ;
#7191=ORIENTED_EDGE('',*,*,#5207,.T.) ;
#7192=ORIENTED_EDGE('',*,*,#5208,.F.) ;
#7193=ORIENTED_EDGE('',*,*,#5204,.F.) ;
#7194=ORIENTED_EDGE('',*,*,#5209,.T.) ;
#7195=ORIENTED_EDGE('',*,*,#5210,.T.) ;
#7196=ORIENTED_EDGE('',*,*,#5211,.F.) ;
#7197=ORIENTED_EDGE('',*,*,#5207,.F.) ;
#7198=ORIENTED_EDGE('',*,*,#5212,.T.) ;
#7199=ORIENTED_EDGE('',*,*,#5213,.T.) ;
#7200=ORIENTED_EDGE('',*,*,#5214,.F.) ;
#7201=ORIENTED_EDGE('',*,*,#5210,.F.) ;
#7202=ORIENTED_EDGE('',*,*,#5215,.T.) ;
#7203=ORIENTED_EDGE('',*,*,#5216,.T.) ;
#7204=ORIENTED_EDGE('',*,*,#5217,.F.) ;
#7205=ORIENTED_EDGE('',*,*,#5213,.F.) ;
#7206=ORIENTED_EDGE('',*,*,#5218,.T.) ;
#7207=ORIENTED_EDGE('',*,*,#5219,.T.) ;
#7208=ORIENTED_EDGE('',*,*,#5220,.F.) ;
#7209=ORIENTED_EDGE('',*,*,#5216,.F.) ;
#7210=ORIENTED_EDGE('',*,*,#5221,.T.) ;
#7211=ORIENTED_EDGE('',*,*,#5222,.T.) ;
#7212=ORIENTED_EDGE('',*,*,#5223,.F.) ;
#7213=ORIENTED_EDGE('',*,*,#5219,.F.) ;
#7214=ORIENTED_EDGE('',*,*,#5224,.T.) ;
#7215=ORIENTED_EDGE('',*,*,#5225,.T.) ;
#7216=ORIENTED_EDGE('',*,*,#5226,.F.) ;
#7217=ORIENTED_EDGE('',*,*,#5222,.F.) ;
#7218=ORIENTED_EDGE('',*,*,#5227,.T.) ;
#7219=ORIENTED_EDGE('',*,*,#5228,.T.) ;
#7220=ORIENTED_EDGE('',*,*,#5229,.F.) ;
#7221=ORIENTED_EDGE('',*,*,#5225,.F.) ;
#7222=ORIENTED_EDGE('',*,*,#5230,.T.) ;
#7223=ORIENTED_EDGE('',*,*,#5231,.T.) ;
#7224=ORIENTED_EDGE('',*,*,#5232,.F.) ;
#7225=ORIENTED_EDGE('',*,*,#5228,.F.) ;
#7226=ORIENTED_EDGE('',*,*,#5233,.T.) ;
#7227=ORIENTED_EDGE('',*,*,#5234,.T.) ;
#7228=ORIENTED_EDGE('',*,*,#5235,.F.) ;
#7229=ORIENTED_EDGE('',*,*,#5231,.F.) ;
#7230=ORIENTED_EDGE('',*,*,#5236,.T.) ;
#7231=ORIENTED_EDGE('',*,*,#5237,.T.) ;
#7232=ORIENTED_EDGE('',*,*,#5238,.F.) ;
#7233=ORIENTED_EDGE('',*,*,#5234,.F.) ;
#7234=ORIENTED_EDGE('',*,*,#5239,.T.) ;
#7235=ORIENTED_EDGE('',*,*,#5240,.T.) ;
#7236=ORIENTED_EDGE('',*,*,#5241,.F.) ;
#7237=ORIENTED_EDGE('',*,*,#5237,.F.) ;
#7238=ORIENTED_EDGE('',*,*,#5242,.T.) ;
#7239=ORIENTED_EDGE('',*,*,#5243,.T.) ;
#7240=ORIENTED_EDGE('',*,*,#5244,.F.) ;
#7241=ORIENTED_EDGE('',*,*,#5240,.F.) ;
#7242=ORIENTED_EDGE('',*,*,#5245,.T.) ;
#7243=ORIENTED_EDGE('',*,*,#5246,.T.) ;
#7244=ORIENTED_EDGE('',*,*,#5247,.F.) ;
#7245=ORIENTED_EDGE('',*,*,#5243,.F.) ;
#7246=ORIENTED_EDGE('',*,*,#5248,.T.) ;
#7247=ORIENTED_EDGE('',*,*,#5249,.T.) ;
#7248=ORIENTED_EDGE('',*,*,#5250,.F.) ;
#7249=ORIENTED_EDGE('',*,*,#5246,.F.) ;
#7250=ORIENTED_EDGE('',*,*,#5251,.T.) ;
#7251=ORIENTED_EDGE('',*,*,#5252,.T.) ;
#7252=ORIENTED_EDGE('',*,*,#5253,.F.) ;
#7253=ORIENTED_EDGE('',*,*,#5249,.F.) ;
#7254=ORIENTED_EDGE('',*,*,#5254,.T.) ;
#7255=ORIENTED_EDGE('',*,*,#5255,.T.) ;
#7256=ORIENTED_EDGE('',*,*,#5256,.F.) ;
#7257=ORIENTED_EDGE('',*,*,#5252,.F.) ;
#7258=ORIENTED_EDGE('',*,*,#5257,.T.) ;
#7259=ORIENTED_EDGE('',*,*,#5258,.T.) ;
#7260=ORIENTED_EDGE('',*,*,#5259,.F.) ;
#7261=ORIENTED_EDGE('',*,*,#5255,.F.) ;
#7262=ORIENTED_EDGE('',*,*,#5260,.T.) ;
#7263=ORIENTED_EDGE('',*,*,#5261,.T.) ;
#7264=ORIENTED_EDGE('',*,*,#5262,.F.) ;
#7265=ORIENTED_EDGE('',*,*,#5258,.F.) ;
#7266=ORIENTED_EDGE('',*,*,#5263,.T.) ;
#7267=ORIENTED_EDGE('',*,*,#5264,.T.) ;
#7268=ORIENTED_EDGE('',*,*,#5265,.F.) ;
#7269=ORIENTED_EDGE('',*,*,#5261,.F.) ;
#7270=ORIENTED_EDGE('',*,*,#5266,.T.) ;
#7271=ORIENTED_EDGE('',*,*,#5267,.T.) ;
#7272=ORIENTED_EDGE('',*,*,#5268,.F.) ;
#7273=ORIENTED_EDGE('',*,*,#5264,.F.) ;
#7274=ORIENTED_EDGE('',*,*,#5269,.T.) ;
#7275=ORIENTED_EDGE('',*,*,#5270,.T.) ;
#7276=ORIENTED_EDGE('',*,*,#5271,.F.) ;
#7277=ORIENTED_EDGE('',*,*,#5267,.F.) ;
#7278=ORIENTED_EDGE('',*,*,#5272,.T.) ;
#7279=ORIENTED_EDGE('',*,*,#5273,.T.) ;
#7280=ORIENTED_EDGE('',*,*,#5274,.F.) ;
#7281=ORIENTED_EDGE('',*,*,#5270,.F.) ;
#7282=ORIENTED_EDGE('',*,*,#5275,.T.) ;
#7283=ORIENTED_EDGE('',*,*,#5276,.T.) ;
#7284=ORIENTED_EDGE('',*,*,#5277,.F.) ;
#7285=ORIENTED_EDGE('',*,*,#5273,.F.) ;
#7286=ORIENTED_EDGE('',*,*,#5278,.T.) ;
#7287=ORIENTED_EDGE('',*,*,#5279,.T.) ;
#7288=ORIENTED_EDGE('',*,*,#5280,.F.) ;
#7289=ORIENTED_EDGE('',*,*,#5276,.F.) ;
#7290=ORIENTED_EDGE('',*,*,#5281,.T.) ;
#7291=ORIENTED_EDGE('',*,*,#5282,.T.) ;
#7292=ORIENTED_EDGE('',*,*,#5283,.F.) ;
#7293=ORIENTED_EDGE('',*,*,#5279,.F.) ;
#7294=ORIENTED_EDGE('',*,*,#5284,.T.) ;
#7295=ORIENTED_EDGE('',*,*,#5285,.T.) ;
#7296=ORIENTED_EDGE('',*,*,#5286,.F.) ;
#7297=ORIENTED_EDGE('',*,*,#5282,.F.) ;
#7298=ORIENTED_EDGE('',*,*,#5287,.T.) ;
#7299=ORIENTED_EDGE('',*,*,#5288,.T.) ;
#7300=ORIENTED_EDGE('',*,*,#5289,.F.) ;
#7301=ORIENTED_EDGE('',*,*,#5285,.F.) ;
#7302=ORIENTED_EDGE('',*,*,#5290,.T.) ;
#7303=ORIENTED_EDGE('',*,*,#5291,.T.) ;
#7304=ORIENTED_EDGE('',*,*,#5292,.F.) ;
#7305=ORIENTED_EDGE('',*,*,#5288,.F.) ;
#7306=ORIENTED_EDGE('',*,*,#5293,.T.) ;
#7307=ORIENTED_EDGE('',*,*,#5294,.T.) ;
#7308=ORIENTED_EDGE('',*,*,#5295,.F.) ;
#7309=ORIENTED_EDGE('',*,*,#5291,.F.) ;
#7310=ORIENTED_EDGE('',*,*,#5296,.T.) ;
#7311=ORIENTED_EDGE('',*,*,#5297,.T.) ;
#7312=ORIENTED_EDGE('',*,*,#5298,.F.) ;
#7313=ORIENTED_EDGE('',*,*,#5294,.F.) ;
#7314=ORIENTED_EDGE('',*,*,#5299,.T.) ;
#7315=ORIENTED_EDGE('',*,*,#5300,.T.) ;
#7316=ORIENTED_EDGE('',*,*,#5301,.F.) ;
#7317=ORIENTED_EDGE('',*,*,#5297,.F.) ;
#7318=ORIENTED_EDGE('',*,*,#5302,.T.) ;
#7319=ORIENTED_EDGE('',*,*,#5303,.T.) ;
#7320=ORIENTED_EDGE('',*,*,#5304,.F.) ;
#7321=ORIENTED_EDGE('',*,*,#5300,.F.) ;
#7322=ORIENTED_EDGE('',*,*,#5305,.T.) ;
#7323=ORIENTED_EDGE('',*,*,#5306,.T.) ;
#7324=ORIENTED_EDGE('',*,*,#5307,.F.) ;
#7325=ORIENTED_EDGE('',*,*,#5303,.F.) ;
#7326=ORIENTED_EDGE('',*,*,#5308,.T.) ;
#7327=ORIENTED_EDGE('',*,*,#5309,.T.) ;
#7328=ORIENTED_EDGE('',*,*,#5310,.F.) ;
#7329=ORIENTED_EDGE('',*,*,#5306,.F.) ;
#7330=ORIENTED_EDGE('',*,*,#5311,.T.) ;
#7331=ORIENTED_EDGE('',*,*,#5312,.T.) ;
#7332=ORIENTED_EDGE('',*,*,#5313,.F.) ;
#7333=ORIENTED_EDGE('',*,*,#5309,.F.) ;
#7334=ORIENTED_EDGE('',*,*,#5314,.T.) ;
#7335=ORIENTED_EDGE('',*,*,#5315,.T.) ;
#7336=ORIENTED_EDGE('',*,*,#5316,.F.) ;
#7337=ORIENTED_EDGE('',*,*,#5312,.F.) ;
#7338=ORIENTED_EDGE('',*,*,#5317,.T.) ;
#7339=ORIENTED_EDGE('',*,*,#5318,.T.) ;
#7340=ORIENTED_EDGE('',*,*,#5319,.F.) ;
#7341=ORIENTED_EDGE('',*,*,#5315,.F.) ;
#7342=ORIENTED_EDGE('',*,*,#5320,.T.) ;
#7343=ORIENTED_EDGE('',*,*,#5321,.T.) ;
#7344=ORIENTED_EDGE('',*,*,#5322,.F.) ;
#7345=ORIENTED_EDGE('',*,*,#5318,.F.) ;
#7346=ORIENTED_EDGE('',*,*,#5323,.T.) ;
#7347=ORIENTED_EDGE('',*,*,#5324,.T.) ;
#7348=ORIENTED_EDGE('',*,*,#5325,.F.) ;
#7349=ORIENTED_EDGE('',*,*,#5321,.F.) ;
#7350=ORIENTED_EDGE('',*,*,#5326,.T.) ;
#7351=ORIENTED_EDGE('',*,*,#5327,.T.) ;
#7352=ORIENTED_EDGE('',*,*,#5328,.F.) ;
#7353=ORIENTED_EDGE('',*,*,#5324,.F.) ;
#7354=ORIENTED_EDGE('',*,*,#5329,.T.) ;
#7355=ORIENTED_EDGE('',*,*,#5330,.T.) ;
#7356=ORIENTED_EDGE('',*,*,#5331,.F.) ;
#7357=ORIENTED_EDGE('',*,*,#5327,.F.) ;
#7358=ORIENTED_EDGE('',*,*,#5332,.T.) ;
#7359=ORIENTED_EDGE('',*,*,#5333,.T.) ;
#7360=ORIENTED_EDGE('',*,*,#5334,.F.) ;
#7361=ORIENTED_EDGE('',*,*,#5330,.F.) ;
#7362=ORIENTED_EDGE('',*,*,#5335,.T.) ;
#7363=ORIENTED_EDGE('',*,*,#5336,.T.) ;
#7364=ORIENTED_EDGE('',*,*,#5337,.F.) ;
#7365=ORIENTED_EDGE('',*,*,#5333,.F.) ;
#7366=ORIENTED_EDGE('',*,*,#5338,.T.) ;
#7367=ORIENTED_EDGE('',*,*,#5339,.T.) ;
#7368=ORIENTED_EDGE('',*,*,#5340,.F.) ;
#7369=ORIENTED_EDGE('',*,*,#5336,.F.) ;
#7370=ORIENTED_EDGE('',*,*,#5341,.T.) ;
#7371=ORIENTED_EDGE('',*,*,#5342,.T.) ;
#7372=ORIENTED_EDGE('',*,*,#5343,.F.) ;
#7373=ORIENTED_EDGE('',*,*,#5339,.F.) ;
#7374=ORIENTED_EDGE('',*,*,#5344,.T.) ;
#7375=ORIENTED_EDGE('',*,*,#5345,.T.) ;
#7376=ORIENTED_EDGE('',*,*,#5346,.F.) ;
#7377=ORIENTED_EDGE('',*,*,#5342,.F.) ;
#7378=ORIENTED_EDGE('',*,*,#5347,.T.) ;
#7379=ORIENTED_EDGE('',*,*,#5348,.T.) ;
#7380=ORIENTED_EDGE('',*,*,#5349,.F.) ;
#7381=ORIENTED_EDGE('',*,*,#5345,.F.) ;
#7382=ORIENTED_EDGE('',*,*,#5350,.T.) ;
#7383=ORIENTED_EDGE('',*,*,#5351,.T.) ;
#7384=ORIENTED_EDGE('',*,*,#5352,.F.) ;
#7385=ORIENTED_EDGE('',*,*,#5348,.F.) ;
#7386=ORIENTED_EDGE('',*,*,#5353,.T.) ;
#7387=ORIENTED_EDGE('',*,*,#5354,.T.) ;
#7388=ORIENTED_EDGE('',*,*,#5355,.F.) ;
#7389=ORIENTED_EDGE('',*,*,#5351,.F.) ;
#7390=ORIENTED_EDGE('',*,*,#5356,.T.) ;
#7391=ORIENTED_EDGE('',*,*,#5357,.T.) ;
#7392=ORIENTED_EDGE('',*,*,#5358,.F.) ;
#7393=ORIENTED_EDGE('',*,*,#5354,.F.) ;
#7394=ORIENTED_EDGE('',*,*,#5359,.T.) ;
#7395=ORIENTED_EDGE('',*,*,#5360,.T.) ;
#7396=ORIENTED_EDGE('',*,*,#5361,.F.) ;
#7397=ORIENTED_EDGE('',*,*,#5357,.F.) ;
#7398=ORIENTED_EDGE('',*,*,#5362,.T.) ;
#7399=ORIENTED_EDGE('',*,*,#5363,.T.) ;
#7400=ORIENTED_EDGE('',*,*,#5364,.F.) ;
#7401=ORIENTED_EDGE('',*,*,#5360,.F.) ;
#7402=ORIENTED_EDGE('',*,*,#5365,.T.) ;
#7403=ORIENTED_EDGE('',*,*,#5366,.T.) ;
#7404=ORIENTED_EDGE('',*,*,#5367,.F.) ;
#7405=ORIENTED_EDGE('',*,*,#5363,.F.) ;
#7406=ORIENTED_EDGE('',*,*,#5368,.T.) ;
#7407=ORIENTED_EDGE('',*,*,#5369,.T.) ;
#7408=ORIENTED_EDGE('',*,*,#5370,.F.) ;
#7409=ORIENTED_EDGE('',*,*,#5366,.F.) ;
#7410=ORIENTED_EDGE('',*,*,#5371,.T.) ;
#7411=ORIENTED_EDGE('',*,*,#5372,.T.) ;
#7412=ORIENTED_EDGE('',*,*,#5373,.F.) ;
#7413=ORIENTED_EDGE('',*,*,#5369,.F.) ;
#7414=ORIENTED_EDGE('',*,*,#5374,.T.) ;
#7415=ORIENTED_EDGE('',*,*,#5375,.T.) ;
#7416=ORIENTED_EDGE('',*,*,#5376,.F.) ;
#7417=ORIENTED_EDGE('',*,*,#5372,.F.) ;
#7418=ORIENTED_EDGE('',*,*,#5377,.T.) ;
#7419=ORIENTED_EDGE('',*,*,#5378,.T.) ;
#7420=ORIENTED_EDGE('',*,*,#5379,.F.) ;
#7421=ORIENTED_EDGE('',*,*,#5375,.F.) ;
#7422=ORIENTED_EDGE('',*,*,#5380,.T.) ;
#7423=ORIENTED_EDGE('',*,*,#5381,.T.) ;
#7424=ORIENTED_EDGE('',*,*,#5382,.F.) ;
#7425=ORIENTED_EDGE('',*,*,#5378,.F.) ;
#7426=ORIENTED_EDGE('',*,*,#5383,.T.) ;
#7427=ORIENTED_EDGE('',*,*,#5384,.T.) ;
#7428=ORIENTED_EDGE('',*,*,#5385,.F.) ;
#7429=ORIENTED_EDGE('',*,*,#5381,.F.) ;
#7430=ORIENTED_EDGE('',*,*,#5386,.T.) ;
#7431=ORIENTED_EDGE('',*,*,#5387,.T.) ;
#7432=ORIENTED_EDGE('',*,*,#5388,.F.) ;
#7433=ORIENTED_EDGE('',*,*,#5384,.F.) ;
#7434=ORIENTED_EDGE('',*,*,#5389,.T.) ;
#7435=ORIENTED_EDGE('',*,*,#5390,.T.) ;
#7436=ORIENTED_EDGE('',*,*,#5391,.F.) ;
#7437=ORIENTED_EDGE('',*,*,#5387,.F.) ;
#7438=ORIENTED_EDGE('',*,*,#5392,.T.) ;
#7439=ORIENTED_EDGE('',*,*,#5393,.T.) ;
#7440=ORIENTED_EDGE('',*,*,#5394,.F.) ;
#7441=ORIENTED_EDGE('',*,*,#5390,.F.) ;
#7442=ORIENTED_EDGE('',*,*,#5395,.T.) ;
#7443=ORIENTED_EDGE('',*,*,#5396,.T.) ;
#7444=ORIENTED_EDGE('',*,*,#5397,.F.) ;
#7445=ORIENTED_EDGE('',*,*,#5393,.F.) ;
#7446=ORIENTED_EDGE('',*,*,#5398,.T.) ;
#7447=ORIENTED_EDGE('',*,*,#5399,.T.) ;
#7448=ORIENTED_EDGE('',*,*,#5400,.F.) ;
#7449=ORIENTED_EDGE('',*,*,#5396,.F.) ;
#7450=ORIENTED_EDGE('',*,*,#5401,.T.) ;
#7451=ORIENTED_EDGE('',*,*,#5402,.T.) ;
#7452=ORIENTED_EDGE('',*,*,#5403,.F.) ;
#7453=ORIENTED_EDGE('',*,*,#5399,.F.) ;
#7454=ORIENTED_EDGE('',*,*,#5404,.T.) ;
#7455=ORIENTED_EDGE('',*,*,#5405,.T.) ;
#7456=ORIENTED_EDGE('',*,*,#5406,.F.) ;
#7457=ORIENTED_EDGE('',*,*,#5402,.F.) ;
#7458=ORIENTED_EDGE('',*,*,#5407,.T.) ;
#7459=ORIENTED_EDGE('',*,*,#5408,.T.) ;
#7460=ORIENTED_EDGE('',*,*,#5409,.F.) ;
#7461=ORIENTED_EDGE('',*,*,#5405,.F.) ;
#7462=ORIENTED_EDGE('',*,*,#5410,.T.) ;
#7463=ORIENTED_EDGE('',*,*,#5411,.T.) ;
#7464=ORIENTED_EDGE('',*,*,#5412,.F.) ;
#7465=ORIENTED_EDGE('',*,*,#5408,.F.) ;
#7466=ORIENTED_EDGE('',*,*,#5413,.T.) ;
#7467=ORIENTED_EDGE('',*,*,#5414,.T.) ;
#7468=ORIENTED_EDGE('',*,*,#5415,.F.) ;
#7469=ORIENTED_EDGE('',*,*,#5411,.F.) ;
#7470=ORIENTED_EDGE('',*,*,#5416,.T.) ;
#7471=ORIENTED_EDGE('',*,*,#5417,.T.) ;
#7472=ORIENTED_EDGE('',*,*,#5418,.F.) ;
#7473=ORIENTED_EDGE('',*,*,#5414,.F.) ;
#7474=ORIENTED_EDGE('',*,*,#5419,.T.) ;
#7475=ORIENTED_EDGE('',*,*,#5420,.T.) ;
#7476=ORIENTED_EDGE('',*,*,#5421,.F.) ;
#7477=ORIENTED_EDGE('',*,*,#5417,.F.) ;
#7478=ORIENTED_EDGE('',*,*,#5422,.T.) ;
#7479=ORIENTED_EDGE('',*,*,#5423,.T.) ;
#7480=ORIENTED_EDGE('',*,*,#5424,.F.) ;
#7481=ORIENTED_EDGE('',*,*,#5420,.F.) ;
#7482=ORIENTED_EDGE('',*,*,#5425,.T.) ;
#7483=ORIENTED_EDGE('',*,*,#5426,.T.) ;
#7484=ORIENTED_EDGE('',*,*,#5427,.F.) ;
#7485=ORIENTED_EDGE('',*,*,#5423,.F.) ;
#7486=ORIENTED_EDGE('',*,*,#5428,.T.) ;
#7487=ORIENTED_EDGE('',*,*,#5429,.T.) ;
#7488=ORIENTED_EDGE('',*,*,#5430,.F.) ;
#7489=ORIENTED_EDGE('',*,*,#5426,.F.) ;
#7490=ORIENTED_EDGE('',*,*,#5431,.T.) ;
#7491=ORIENTED_EDGE('',*,*,#5432,.T.) ;
#7492=ORIENTED_EDGE('',*,*,#5433,.F.) ;
#7493=ORIENTED_EDGE('',*,*,#5429,.F.) ;
#7494=ORIENTED_EDGE('',*,*,#5434,.T.) ;
#7495=ORIENTED_EDGE('',*,*,#5435,.T.) ;
#7496=ORIENTED_EDGE('',*,*,#5436,.F.) ;
#7497=ORIENTED_EDGE('',*,*,#5432,.F.) ;
#7498=ORIENTED_EDGE('',*,*,#5437,.T.) ;
#7499=ORIENTED_EDGE('',*,*,#4902,.T.) ;
#7500=ORIENTED_EDGE('',*,*,#5438,.F.) ;
#7501=ORIENTED_EDGE('',*,*,#5435,.F.) ;
#7502=ORIENTED_EDGE('',*,*,#5437,.F.) ;
#7503=ORIENTED_EDGE('',*,*,#5434,.F.) ;
#7504=ORIENTED_EDGE('',*,*,#5431,.F.) ;
#7505=ORIENTED_EDGE('',*,*,#5428,.F.) ;
#7506=ORIENTED_EDGE('',*,*,#5425,.F.) ;
#7507=ORIENTED_EDGE('',*,*,#5422,.F.) ;
#7508=ORIENTED_EDGE('',*,*,#5419,.F.) ;
#7509=ORIENTED_EDGE('',*,*,#5416,.F.) ;
#7510=ORIENTED_EDGE('',*,*,#5413,.F.) ;
#7511=ORIENTED_EDGE('',*,*,#5410,.F.) ;
#7512=ORIENTED_EDGE('',*,*,#5407,.F.) ;
#7513=ORIENTED_EDGE('',*,*,#5404,.F.) ;
#7514=ORIENTED_EDGE('',*,*,#5401,.F.) ;
#7515=ORIENTED_EDGE('',*,*,#5398,.F.) ;
#7516=ORIENTED_EDGE('',*,*,#5395,.F.) ;
#7517=ORIENTED_EDGE('',*,*,#5392,.F.) ;
#7518=ORIENTED_EDGE('',*,*,#5389,.F.) ;
#7519=ORIENTED_EDGE('',*,*,#5386,.F.) ;
#7520=ORIENTED_EDGE('',*,*,#5383,.F.) ;
#7521=ORIENTED_EDGE('',*,*,#5380,.F.) ;
#7522=ORIENTED_EDGE('',*,*,#5377,.F.) ;
#7523=ORIENTED_EDGE('',*,*,#5374,.F.) ;
#7524=ORIENTED_EDGE('',*,*,#5371,.F.) ;
#7525=ORIENTED_EDGE('',*,*,#5368,.F.) ;
#7526=ORIENTED_EDGE('',*,*,#5365,.F.) ;
#7527=ORIENTED_EDGE('',*,*,#5362,.F.) ;
#7528=ORIENTED_EDGE('',*,*,#5359,.F.) ;
#7529=ORIENTED_EDGE('',*,*,#5356,.F.) ;
#7530=ORIENTED_EDGE('',*,*,#5353,.F.) ;
#7531=ORIENTED_EDGE('',*,*,#5350,.F.) ;
#7532=ORIENTED_EDGE('',*,*,#5347,.F.) ;
#7533=ORIENTED_EDGE('',*,*,#5344,.F.) ;
#7534=ORIENTED_EDGE('',*,*,#5341,.F.) ;
#7535=ORIENTED_EDGE('',*,*,#5338,.F.) ;
#7536=ORIENTED_EDGE('',*,*,#5335,.F.) ;
#7537=ORIENTED_EDGE('',*,*,#5332,.F.) ;
#7538=ORIENTED_EDGE('',*,*,#5329,.F.) ;
#7539=ORIENTED_EDGE('',*,*,#5326,.F.) ;
#7540=ORIENTED_EDGE('',*,*,#5323,.F.) ;
#7541=ORIENTED_EDGE('',*,*,#5320,.F.) ;
#7542=ORIENTED_EDGE('',*,*,#5317,.F.) ;
#7543=ORIENTED_EDGE('',*,*,#5314,.F.) ;
#7544=ORIENTED_EDGE('',*,*,#5311,.F.) ;
#7545=ORIENTED_EDGE('',*,*,#5308,.F.) ;
#7546=ORIENTED_EDGE('',*,*,#5305,.F.) ;
#7547=ORIENTED_EDGE('',*,*,#5302,.F.) ;
#7548=ORIENTED_EDGE('',*,*,#5299,.F.) ;
#7549=ORIENTED_EDGE('',*,*,#5296,.F.) ;
#7550=ORIENTED_EDGE('',*,*,#5293,.F.) ;
#7551=ORIENTED_EDGE('',*,*,#5290,.F.) ;
#7552=ORIENTED_EDGE('',*,*,#5287,.F.) ;
#7553=ORIENTED_EDGE('',*,*,#5284,.F.) ;
#7554=ORIENTED_EDGE('',*,*,#5281,.F.) ;
#7555=ORIENTED_EDGE('',*,*,#5278,.F.) ;
#7556=ORIENTED_EDGE('',*,*,#5275,.F.) ;
#7557=ORIENTED_EDGE('',*,*,#5272,.F.) ;
#7558=ORIENTED_EDGE('',*,*,#5269,.F.) ;
#7559=ORIENTED_EDGE('',*,*,#5266,.F.) ;
#7560=ORIENTED_EDGE('',*,*,#5263,.F.) ;
#7561=ORIENTED_EDGE('',*,*,#5260,.F.) ;
#7562=ORIENTED_EDGE('',*,*,#5257,.F.) ;
#7563=ORIENTED_EDGE('',*,*,#5254,.F.) ;
#7564=ORIENTED_EDGE('',*,*,#5251,.F.) ;
#7565=ORIENTED_EDGE('',*,*,#5248,.F.) ;
#7566=ORIENTED_EDGE('',*,*,#5245,.F.) ;
#7567=ORIENTED_EDGE('',*,*,#5242,.F.) ;
#7568=ORIENTED_EDGE('',*,*,#5239,.F.) ;
#7569=ORIENTED_EDGE('',*,*,#5236,.F.) ;
#7570=ORIENTED_EDGE('',*,*,#5233,.F.) ;
#7571=ORIENTED_EDGE('',*,*,#5230,.F.) ;
#7572=ORIENTED_EDGE('',*,*,#5227,.F.) ;
#7573=ORIENTED_EDGE('',*,*,#5224,.F.) ;
#7574=ORIENTED_EDGE('',*,*,#5221,.F.) ;
#7575=ORIENTED_EDGE('',*,*,#5218,.F.) ;
#7576=ORIENTED_EDGE('',*,*,#5215,.F.) ;
#7577=ORIENTED_EDGE('',*,*,#5212,.F.) ;
#7578=ORIENTED_EDGE('',*,*,#5209,.F.) ;
#7579=ORIENTED_EDGE('',*,*,#5206,.F.) ;
#7580=ORIENTED_EDGE('',*,*,#5203,.F.) ;
#7581=ORIENTED_EDGE('',*,*,#5200,.F.) ;
#7582=ORIENTED_EDGE('',*,*,#5197,.F.) ;
#7583=ORIENTED_EDGE('',*,*,#5194,.F.) ;
#7584=ORIENTED_EDGE('',*,*,#5191,.F.) ;
#7585=ORIENTED_EDGE('',*,*,#5188,.F.) ;
#7586=ORIENTED_EDGE('',*,*,#5185,.F.) ;
#7587=ORIENTED_EDGE('',*,*,#5182,.F.) ;
#7588=ORIENTED_EDGE('',*,*,#5179,.F.) ;
#7589=ORIENTED_EDGE('',*,*,#5176,.F.) ;
#7590=ORIENTED_EDGE('',*,*,#5173,.F.) ;
#7591=ORIENTED_EDGE('',*,*,#5170,.F.) ;
#7592=ORIENTED_EDGE('',*,*,#5167,.F.) ;
#7593=ORIENTED_EDGE('',*,*,#5164,.F.) ;
#7594=ORIENTED_EDGE('',*,*,#5161,.F.) ;
#7595=ORIENTED_EDGE('',*,*,#5158,.F.) ;
#7596=ORIENTED_EDGE('',*,*,#5155,.F.) ;
#7597=ORIENTED_EDGE('',*,*,#5152,.F.) ;
#7598=ORIENTED_EDGE('',*,*,#5149,.F.) ;
#7599=ORIENTED_EDGE('',*,*,#5146,.F.) ;
#7600=ORIENTED_EDGE('',*,*,#5143,.F.) ;
#7601=ORIENTED_EDGE('',*,*,#5140,.F.) ;
#7602=ORIENTED_EDGE('',*,*,#5137,.F.) ;
#7603=ORIENTED_EDGE('',*,*,#5134,.F.) ;
#7604=ORIENTED_EDGE('',*,*,#5131,.F.) ;
#7605=ORIENTED_EDGE('',*,*,#5128,.F.) ;
#7606=ORIENTED_EDGE('',*,*,#5125,.F.) ;
#7607=ORIENTED_EDGE('',*,*,#5122,.F.) ;
#7608=ORIENTED_EDGE('',*,*,#5119,.F.) ;
#7609=ORIENTED_EDGE('',*,*,#5116,.F.) ;
#7610=ORIENTED_EDGE('',*,*,#5113,.F.) ;
#7611=ORIENTED_EDGE('',*,*,#5110,.F.) ;
#7612=ORIENTED_EDGE('',*,*,#5107,.F.) ;
#7613=ORIENTED_EDGE('',*,*,#5104,.F.) ;
#7614=ORIENTED_EDGE('',*,*,#5101,.F.) ;
#7615=ORIENTED_EDGE('',*,*,#5098,.F.) ;
#7616=ORIENTED_EDGE('',*,*,#5095,.F.) ;
#7617=ORIENTED_EDGE('',*,*,#5092,.F.) ;
#7618=ORIENTED_EDGE('',*,*,#5089,.F.) ;
#7619=ORIENTED_EDGE('',*,*,#5086,.F.) ;
#7620=ORIENTED_EDGE('',*,*,#5083,.F.) ;
#7621=ORIENTED_EDGE('',*,*,#5080,.F.) ;
#7622=ORIENTED_EDGE('',*,*,#5077,.F.) ;
#7623=ORIENTED_EDGE('',*,*,#5074,.F.) ;
#7624=ORIENTED_EDGE('',*,*,#5071,.F.) ;
#7625=ORIENTED_EDGE('',*,*,#5068,.F.) ;
#7626=ORIENTED_EDGE('',*,*,#5065,.F.) ;
#7627=ORIENTED_EDGE('',*,*,#5062,.F.) ;
#7628=ORIENTED_EDGE('',*,*,#5059,.F.) ;
#7629=ORIENTED_EDGE('',*,*,#5056,.F.) ;
#7630=ORIENTED_EDGE('',*,*,#5053,.F.) ;
#7631=ORIENTED_EDGE('',*,*,#5050,.F.) ;
#7632=ORIENTED_EDGE('',*,*,#5047,.F.) ;
#7633=ORIENTED_EDGE('',*,*,#5044,.F.) ;
#7634=ORIENTED_EDGE('',*,*,#5041,.F.) ;
#7635=ORIENTED_EDGE('',*,*,#5038,.F.) ;
#7636=ORIENTED_EDGE('',*,*,#5035,.F.) ;
#7637=ORIENTED_EDGE('',*,*,#5032,.F.) ;
#7638=ORIENTED_EDGE('',*,*,#5029,.F.) ;
#7639=ORIENTED_EDGE('',*,*,#5026,.F.) ;
#7640=ORIENTED_EDGE('',*,*,#5023,.F.) ;
#7641=ORIENTED_EDGE('',*,*,#5020,.F.) ;
#7642=ORIENTED_EDGE('',*,*,#5017,.F.) ;
#7643=ORIENTED_EDGE('',*,*,#5014,.F.) ;
#7644=ORIENTED_EDGE('',*,*,#5011,.F.) ;
#7645=ORIENTED_EDGE('',*,*,#5008,.F.) ;
#7646=ORIENTED_EDGE('',*,*,#5005,.F.) ;
#7647=ORIENTED_EDGE('',*,*,#5002,.F.) ;
#7648=ORIENTED_EDGE('',*,*,#4999,.F.) ;
#7649=ORIENTED_EDGE('',*,*,#4996,.F.) ;
#7650=ORIENTED_EDGE('',*,*,#4993,.F.) ;
#7651=ORIENTED_EDGE('',*,*,#4990,.F.) ;
#7652=ORIENTED_EDGE('',*,*,#4987,.F.) ;
#7653=ORIENTED_EDGE('',*,*,#4984,.F.) ;
#7654=ORIENTED_EDGE('',*,*,#4981,.F.) ;
#7655=ORIENTED_EDGE('',*,*,#4978,.F.) ;
#7656=ORIENTED_EDGE('',*,*,#4975,.F.) ;
#7657=ORIENTED_EDGE('',*,*,#4972,.F.) ;
#7658=ORIENTED_EDGE('',*,*,#4969,.F.) ;
#7659=ORIENTED_EDGE('',*,*,#4966,.F.) ;
#7660=ORIENTED_EDGE('',*,*,#4963,.F.) ;
#7661=ORIENTED_EDGE('',*,*,#4960,.F.) ;
#7662=ORIENTED_EDGE('',*,*,#4957,.F.) ;
#7663=ORIENTED_EDGE('',*,*,#4954,.F.) ;
#7664=ORIENTED_EDGE('',*,*,#4951,.F.) ;
#7665=ORIENTED_EDGE('',*,*,#4948,.F.) ;
#7666=ORIENTED_EDGE('',*,*,#4945,.F.) ;
#7667=ORIENTED_EDGE('',*,*,#4942,.F.) ;
#7668=ORIENTED_EDGE('',*,*,#4939,.F.) ;
#7669=ORIENTED_EDGE('',*,*,#4936,.F.) ;
#7670=ORIENTED_EDGE('',*,*,#4933,.F.) ;
#7671=ORIENTED_EDGE('',*,*,#4930,.F.) ;
#7672=ORIENTED_EDGE('',*,*,#4927,.F.) ;
#7673=ORIENTED_EDGE('',*,*,#4924,.F.) ;
#7674=ORIENTED_EDGE('',*,*,#4921,.F.) ;
#7675=ORIENTED_EDGE('',*,*,#4918,.F.) ;
#7676=ORIENTED_EDGE('',*,*,#4915,.F.) ;
#7677=ORIENTED_EDGE('',*,*,#4912,.F.) ;
#7678=ORIENTED_EDGE('',*,*,#4909,.F.) ;
#7679=ORIENTED_EDGE('',*,*,#4906,.F.) ;
#7680=ORIENTED_EDGE('',*,*,#4903,.F.) ;
#7681=ORIENTED_EDGE('',*,*,#4899,.F.) ;
#7682=ORIENTED_EDGE('',*,*,#5439,.F.) ;
#7683=ORIENTED_EDGE('',*,*,#5440,.F.) ;
#7684=ORIENTED_EDGE('',*,*,#5441,.F.) ;
#7685=ORIENTED_EDGE('',*,*,#5442,.F.) ;
#7686=ORIENTED_EDGE('',*,*,#5443,.F.) ;
#7687=ORIENTED_EDGE('',*,*,#5444,.F.) ;
#7688=ORIENTED_EDGE('',*,*,#5445,.F.) ;
#7689=ORIENTED_EDGE('',*,*,#5446,.F.) ;
#7690=ORIENTED_EDGE('',*,*,#5447,.F.) ;
#7691=ORIENTED_EDGE('',*,*,#5448,.F.) ;
#7692=ORIENTED_EDGE('',*,*,#5449,.F.) ;
#7693=ORIENTED_EDGE('',*,*,#5450,.F.) ;
#7694=ORIENTED_EDGE('',*,*,#5451,.F.) ;
#7695=ORIENTED_EDGE('',*,*,#5452,.F.) ;
#7696=ORIENTED_EDGE('',*,*,#5453,.F.) ;
#7697=ORIENTED_EDGE('',*,*,#5454,.F.) ;
#7698=ORIENTED_EDGE('',*,*,#5455,.F.) ;
#7699=ORIENTED_EDGE('',*,*,#5456,.F.) ;
#7700=ORIENTED_EDGE('',*,*,#5457,.F.) ;
#7701=ORIENTED_EDGE('',*,*,#5458,.F.) ;
#7702=ORIENTED_EDGE('',*,*,#5459,.F.) ;
#7703=ORIENTED_EDGE('',*,*,#5460,.F.) ;
#7704=ORIENTED_EDGE('',*,*,#5461,.F.) ;
#7705=ORIENTED_EDGE('',*,*,#5462,.F.) ;
#7706=ORIENTED_EDGE('',*,*,#5463,.F.) ;
#7707=ORIENTED_EDGE('',*,*,#5464,.F.) ;
#7708=ORIENTED_EDGE('',*,*,#5465,.F.) ;
#7709=ORIENTED_EDGE('',*,*,#5466,.F.) ;
#7710=ORIENTED_EDGE('',*,*,#5467,.F.) ;
#7711=ORIENTED_EDGE('',*,*,#5468,.F.) ;
#7712=ORIENTED_EDGE('',*,*,#5469,.F.) ;
#7713=ORIENTED_EDGE('',*,*,#5470,.F.) ;
#7714=ORIENTED_EDGE('',*,*,#5471,.F.) ;
#7715=ORIENTED_EDGE('',*,*,#5472,.F.) ;
#7716=ORIENTED_EDGE('',*,*,#5473,.F.) ;
#7717=ORIENTED_EDGE('',*,*,#5474,.F.) ;
#7718=ORIENTED_EDGE('',*,*,#5475,.F.) ;
#7719=ORIENTED_EDGE('',*,*,#5476,.F.) ;
#7720=ORIENTED_EDGE('',*,*,#5477,.F.) ;
#7721=ORIENTED_EDGE('',*,*,#5478,.F.) ;
#7722=ORIENTED_EDGE('',*,*,#5479,.F.) ;
#7723=ORIENTED_EDGE('',*,*,#4901,.T.) ;
#7724=ORIENTED_EDGE('',*,*,#4905,.T.) ;
#7725=ORIENTED_EDGE('',*,*,#4908,.T.) ;
#7726=ORIENTED_EDGE('',*,*,#4911,.T.) ;
#7727=ORIENTED_EDGE('',*,*,#4914,.T.) ;
#7728=ORIENTED_EDGE('',*,*,#4917,.T.) ;
#7729=ORIENTED_EDGE('',*,*,#4920,.T.) ;
#7730=ORIENTED_EDGE('',*,*,#4923,.T.) ;
#7731=ORIENTED_EDGE('',*,*,#4926,.T.) ;
#7732=ORIENTED_EDGE('',*,*,#4929,.T.) ;
#7733=ORIENTED_EDGE('',*,*,#4932,.T.) ;
#7734=ORIENTED_EDGE('',*,*,#4935,.T.) ;
#7735=ORIENTED_EDGE('',*,*,#4938,.T.) ;
#7736=ORIENTED_EDGE('',*,*,#4941,.T.) ;
#7737=ORIENTED_EDGE('',*,*,#4944,.T.) ;
#7738=ORIENTED_EDGE('',*,*,#4947,.T.) ;
#7739=ORIENTED_EDGE('',*,*,#4950,.T.) ;
#7740=ORIENTED_EDGE('',*,*,#4953,.T.) ;
#7741=ORIENTED_EDGE('',*,*,#4956,.T.) ;
#7742=ORIENTED_EDGE('',*,*,#4959,.T.) ;
#7743=ORIENTED_EDGE('',*,*,#4962,.T.) ;
#7744=ORIENTED_EDGE('',*,*,#4965,.T.) ;
#7745=ORIENTED_EDGE('',*,*,#4968,.T.) ;
#7746=ORIENTED_EDGE('',*,*,#4971,.T.) ;
#7747=ORIENTED_EDGE('',*,*,#4974,.T.) ;
#7748=ORIENTED_EDGE('',*,*,#4977,.T.) ;
#7749=ORIENTED_EDGE('',*,*,#4980,.T.) ;
#7750=ORIENTED_EDGE('',*,*,#4983,.T.) ;
#7751=ORIENTED_EDGE('',*,*,#4986,.T.) ;
#7752=ORIENTED_EDGE('',*,*,#4989,.T.) ;
#7753=ORIENTED_EDGE('',*,*,#4992,.T.) ;
#7754=ORIENTED_EDGE('',*,*,#4995,.T.) ;
#7755=ORIENTED_EDGE('',*,*,#4998,.T.) ;
#7756=ORIENTED_EDGE('',*,*,#5001,.T.) ;
#7757=ORIENTED_EDGE('',*,*,#5004,.T.) ;
#7758=ORIENTED_EDGE('',*,*,#5007,.T.) ;
#7759=ORIENTED_EDGE('',*,*,#5010,.T.) ;
#7760=ORIENTED_EDGE('',*,*,#5013,.T.) ;
#7761=ORIENTED_EDGE('',*,*,#5016,.T.) ;
#7762=ORIENTED_EDGE('',*,*,#5019,.T.) ;
#7763=ORIENTED_EDGE('',*,*,#5022,.T.) ;
#7764=ORIENTED_EDGE('',*,*,#5025,.T.) ;
#7765=ORIENTED_EDGE('',*,*,#5028,.T.) ;
#7766=ORIENTED_EDGE('',*,*,#5031,.T.) ;
#7767=ORIENTED_EDGE('',*,*,#5034,.T.) ;
#7768=ORIENTED_EDGE('',*,*,#5037,.T.) ;
#7769=ORIENTED_EDGE('',*,*,#5040,.T.) ;
#7770=ORIENTED_EDGE('',*,*,#5043,.T.) ;
#7771=ORIENTED_EDGE('',*,*,#5046,.T.) ;
#7772=ORIENTED_EDGE('',*,*,#5049,.T.) ;
#7773=ORIENTED_EDGE('',*,*,#5052,.T.) ;
#7774=ORIENTED_EDGE('',*,*,#5055,.T.) ;
#7775=ORIENTED_EDGE('',*,*,#5058,.T.) ;
#7776=ORIENTED_EDGE('',*,*,#5061,.T.) ;
#7777=ORIENTED_EDGE('',*,*,#5064,.T.) ;
#7778=ORIENTED_EDGE('',*,*,#5067,.T.) ;
#7779=ORIENTED_EDGE('',*,*,#5070,.T.) ;
#7780=ORIENTED_EDGE('',*,*,#5073,.T.) ;
#7781=ORIENTED_EDGE('',*,*,#5076,.T.) ;
#7782=ORIENTED_EDGE('',*,*,#5079,.T.) ;
#7783=ORIENTED_EDGE('',*,*,#5082,.T.) ;
#7784=ORIENTED_EDGE('',*,*,#5085,.T.) ;
#7785=ORIENTED_EDGE('',*,*,#5088,.T.) ;
#7786=ORIENTED_EDGE('',*,*,#5091,.T.) ;
#7787=ORIENTED_EDGE('',*,*,#5094,.T.) ;
#7788=ORIENTED_EDGE('',*,*,#5097,.T.) ;
#7789=ORIENTED_EDGE('',*,*,#5100,.T.) ;
#7790=ORIENTED_EDGE('',*,*,#5103,.T.) ;
#7791=ORIENTED_EDGE('',*,*,#5106,.T.) ;
#7792=ORIENTED_EDGE('',*,*,#5109,.T.) ;
#7793=ORIENTED_EDGE('',*,*,#5112,.T.) ;
#7794=ORIENTED_EDGE('',*,*,#5115,.T.) ;
#7795=ORIENTED_EDGE('',*,*,#5118,.T.) ;
#7796=ORIENTED_EDGE('',*,*,#5121,.T.) ;
#7797=ORIENTED_EDGE('',*,*,#5124,.T.) ;
#7798=ORIENTED_EDGE('',*,*,#5127,.T.) ;
#7799=ORIENTED_EDGE('',*,*,#5130,.T.) ;
#7800=ORIENTED_EDGE('',*,*,#5133,.T.) ;
#7801=ORIENTED_EDGE('',*,*,#5136,.T.) ;
#7802=ORIENTED_EDGE('',*,*,#5139,.T.) ;
#7803=ORIENTED_EDGE('',*,*,#5142,.T.) ;
#7804=ORIENTED_EDGE('',*,*,#5145,.T.) ;
#7805=ORIENTED_EDGE('',*,*,#5148,.T.) ;
#7806=ORIENTED_EDGE('',*,*,#5151,.T.) ;
#7807=ORIENTED_EDGE('',*,*,#5154,.T.) ;
#7808=ORIENTED_EDGE('',*,*,#5157,.T.) ;
#7809=ORIENTED_EDGE('',*,*,#5160,.T.) ;
#7810=ORIENTED_EDGE('',*,*,#5163,.T.) ;
#7811=ORIENTED_EDGE('',*,*,#5166,.T.) ;
#7812=ORIENTED_EDGE('',*,*,#5169,.T.) ;
#7813=ORIENTED_EDGE('',*,*,#5172,.T.) ;
#7814=ORIENTED_EDGE('',*,*,#5175,.T.) ;
#7815=ORIENTED_EDGE('',*,*,#5178,.T.) ;
#7816=ORIENTED_EDGE('',*,*,#5181,.T.) ;
#7817=ORIENTED_EDGE('',*,*,#5184,.T.) ;
#7818=ORIENTED_EDGE('',*,*,#5187,.T.) ;
#7819=ORIENTED_EDGE('',*,*,#5190,.T.) ;
#7820=ORIENTED_EDGE('',*,*,#5193,.T.) ;
#7821=ORIENTED_EDGE('',*,*,#5196,.T.) ;
#7822=ORIENTED_EDGE('',*,*,#5199,.T.) ;
#7823=ORIENTED_EDGE('',*,*,#5202,.T.) ;
#7824=ORIENTED_EDGE('',*,*,#5205,.T.) ;
#7825=ORIENTED_EDGE('',*,*,#5208,.T.) ;
#7826=ORIENTED_EDGE('',*,*,#5211,.T.) ;
#7827=ORIENTED_EDGE('',*,*,#5214,.T.) ;
#7828=ORIENTED_EDGE('',*,*,#5217,.T.) ;
#7829=ORIENTED_EDGE('',*,*,#5220,.T.) ;
#7830=ORIENTED_EDGE('',*,*,#5223,.T.) ;
#7831=ORIENTED_EDGE('',*,*,#5226,.T.) ;
#7832=ORIENTED_EDGE('',*,*,#5229,.T.) ;
#7833=ORIENTED_EDGE('',*,*,#5232,.T.) ;
#7834=ORIENTED_EDGE('',*,*,#5235,.T.) ;
#7835=ORIENTED_EDGE('',*,*,#5238,.T.) ;
#7836=ORIENTED_EDGE('',*,*,#5241,.T.) ;
#7837=ORIENTED_EDGE('',*,*,#5244,.T.) ;
#7838=ORIENTED_EDGE('',*,*,#5247,.T.) ;
#7839=ORIENTED_EDGE('',*,*,#5250,.T.) ;
#7840=ORIENTED_EDGE('',*,*,#5253,.T.) ;
#7841=ORIENTED_EDGE('',*,*,#5256,.T.) ;
#7842=ORIENTED_EDGE('',*,*,#5259,.T.) ;
#7843=ORIENTED_EDGE('',*,*,#5262,.T.) ;
#7844=ORIENTED_EDGE('',*,*,#5265,.T.) ;
#7845=ORIENTED_EDGE('',*,*,#5268,.T.) ;
#7846=ORIENTED_EDGE('',*,*,#5271,.T.) ;
#7847=ORIENTED_EDGE('',*,*,#5274,.T.) ;
#7848=ORIENTED_EDGE('',*,*,#5277,.T.) ;
#7849=ORIENTED_EDGE('',*,*,#5280,.T.) ;
#7850=ORIENTED_EDGE('',*,*,#5283,.T.) ;
#7851=ORIENTED_EDGE('',*,*,#5286,.T.) ;
#7852=ORIENTED_EDGE('',*,*,#5289,.T.) ;
#7853=ORIENTED_EDGE('',*,*,#5292,.T.) ;
#7854=ORIENTED_EDGE('',*,*,#5295,.T.) ;
#7855=ORIENTED_EDGE('',*,*,#5298,.T.) ;
#7856=ORIENTED_EDGE('',*,*,#5301,.T.) ;
#7857=ORIENTED_EDGE('',*,*,#5304,.T.) ;
#7858=ORIENTED_EDGE('',*,*,#5307,.T.) ;
#7859=ORIENTED_EDGE('',*,*,#5310,.T.) ;
#7860=ORIENTED_EDGE('',*,*,#5313,.T.) ;
#7861=ORIENTED_EDGE('',*,*,#5316,.T.) ;
#7862=ORIENTED_EDGE('',*,*,#5319,.T.) ;
#7863=ORIENTED_EDGE('',*,*,#5322,.T.) ;
#7864=ORIENTED_EDGE('',*,*,#5325,.T.) ;
#7865=ORIENTED_EDGE('',*,*,#5328,.T.) ;
#7866=ORIENTED_EDGE('',*,*,#5331,.T.) ;
#7867=ORIENTED_EDGE('',*,*,#5334,.T.) ;
#7868=ORIENTED_EDGE('',*,*,#5337,.T.) ;
#7869=ORIENTED_EDGE('',*,*,#5340,.T.) ;
#7870=ORIENTED_EDGE('',*,*,#5343,.T.) ;
#7871=ORIENTED_EDGE('',*,*,#5346,.T.) ;
#7872=ORIENTED_EDGE('',*,*,#5349,.T.) ;
#7873=ORIENTED_EDGE('',*,*,#5352,.T.) ;
#7874=ORIENTED_EDGE('',*,*,#5355,.T.) ;
#7875=ORIENTED_EDGE('',*,*,#5358,.T.) ;
#7876=ORIENTED_EDGE('',*,*,#5361,.T.) ;
#7877=ORIENTED_EDGE('',*,*,#5364,.T.) ;
#7878=ORIENTED_EDGE('',*,*,#5367,.T.) ;
#7879=ORIENTED_EDGE('',*,*,#5370,.T.) ;
#7880=ORIENTED_EDGE('',*,*,#5373,.T.) ;
#7881=ORIENTED_EDGE('',*,*,#5376,.T.) ;
#7882=ORIENTED_EDGE('',*,*,#5379,.T.) ;
#7883=ORIENTED_EDGE('',*,*,#5382,.T.) ;
#7884=ORIENTED_EDGE('',*,*,#5385,.T.) ;
#7885=ORIENTED_EDGE('',*,*,#5388,.T.) ;
#7886=ORIENTED_EDGE('',*,*,#5391,.T.) ;
#7887=ORIENTED_EDGE('',*,*,#5394,.T.) ;
#7888=ORIENTED_EDGE('',*,*,#5397,.T.) ;
#7889=ORIENTED_EDGE('',*,*,#5400,.T.) ;
#7890=ORIENTED_EDGE('',*,*,#5403,.T.) ;
#7891=ORIENTED_EDGE('',*,*,#5406,.T.) ;
#7892=ORIENTED_EDGE('',*,*,#5409,.T.) ;
#7893=ORIENTED_EDGE('',*,*,#5412,.T.) ;
#7894=ORIENTED_EDGE('',*,*,#5415,.T.) ;
#7895=ORIENTED_EDGE('',*,*,#5418,.T.) ;
#7896=ORIENTED_EDGE('',*,*,#5421,.T.) ;
#7897=ORIENTED_EDGE('',*,*,#5424,.T.) ;
#7898=ORIENTED_EDGE('',*,*,#5427,.T.) ;
#7899=ORIENTED_EDGE('',*,*,#5430,.T.) ;
#7900=ORIENTED_EDGE('',*,*,#5433,.T.) ;
#7901=ORIENTED_EDGE('',*,*,#5436,.T.) ;
#7902=ORIENTED_EDGE('',*,*,#5438,.T.) ;
#7903=ORIENTED_EDGE('',*,*,#5480,.T.) ;
#7904=ORIENTED_EDGE('',*,*,#5445,.T.) ;
#7905=ORIENTED_EDGE('',*,*,#5481,.T.) ;
#7906=ORIENTED_EDGE('',*,*,#5482,.F.) ;
#7907=ORIENTED_EDGE('',*,*,#5483,.F.) ;
#7908=ORIENTED_EDGE('',*,*,#5446,.T.) ;
#7909=ORIENTED_EDGE('',*,*,#5483,.T.) ;
#7910=ORIENTED_EDGE('',*,*,#5484,.F.) ;
#7911=ORIENTED_EDGE('',*,*,#5485,.F.) ;
#7912=ORIENTED_EDGE('',*,*,#5486,.F.) ;
#7913=ORIENTED_EDGE('',*,*,#5439,.T.) ;
#7914=ORIENTED_EDGE('',*,*,#5485,.T.) ;
#7915=ORIENTED_EDGE('',*,*,#5487,.F.) ;
#7916=ORIENTED_EDGE('',*,*,#5440,.T.) ;
#7917=ORIENTED_EDGE('',*,*,#5486,.T.) ;
#7918=ORIENTED_EDGE('',*,*,#5488,.F.) ;
#7919=ORIENTED_EDGE('',*,*,#5489,.F.) ;
#7920=ORIENTED_EDGE('',*,*,#5441,.T.) ;
#7921=ORIENTED_EDGE('',*,*,#5489,.T.) ;
#7922=ORIENTED_EDGE('',*,*,#5490,.F.) ;
#7923=ORIENTED_EDGE('',*,*,#5491,.F.) ;
#7924=ORIENTED_EDGE('',*,*,#5442,.T.) ;
#7925=ORIENTED_EDGE('',*,*,#5491,.T.) ;
#7926=ORIENTED_EDGE('',*,*,#5492,.F.) ;
#7927=ORIENTED_EDGE('',*,*,#5493,.F.) ;
#7928=ORIENTED_EDGE('',*,*,#5443,.T.) ;
#7929=ORIENTED_EDGE('',*,*,#5493,.T.) ;
#7930=ORIENTED_EDGE('',*,*,#5494,.F.) ;
#7931=ORIENTED_EDGE('',*,*,#5495,.F.) ;
#7932=ORIENTED_EDGE('',*,*,#5444,.T.) ;
#7933=ORIENTED_EDGE('',*,*,#5495,.T.) ;
#7934=ORIENTED_EDGE('',*,*,#5496,.F.) ;
#7935=ORIENTED_EDGE('',*,*,#5481,.F.) ;
#7936=ORIENTED_EDGE('',*,*,#5497,.F.) ;
#7937=ORIENTED_EDGE('',*,*,#5498,.T.) ;
#7938=ORIENTED_EDGE('',*,*,#5447,.T.) ;
#7939=ORIENTED_EDGE('',*,*,#5498,.F.) ;
#7940=ORIENTED_EDGE('',*,*,#5454,.T.) ;
#7941=ORIENTED_EDGE('',*,*,#5499,.T.) ;
#7942=ORIENTED_EDGE('',*,*,#5500,.F.) ;
#7943=ORIENTED_EDGE('',*,*,#5501,.F.) ;
#7944=ORIENTED_EDGE('',*,*,#5455,.T.) ;
#7945=ORIENTED_EDGE('',*,*,#5501,.T.) ;
#7946=ORIENTED_EDGE('',*,*,#5502,.F.) ;
#7947=ORIENTED_EDGE('',*,*,#5503,.F.) ;
#7948=ORIENTED_EDGE('',*,*,#5504,.F.) ;
#7949=ORIENTED_EDGE('',*,*,#5448,.T.) ;
#7950=ORIENTED_EDGE('',*,*,#5503,.T.) ;
#7951=ORIENTED_EDGE('',*,*,#5505,.F.) ;
#7952=ORIENTED_EDGE('',*,*,#5449,.T.) ;
#7953=ORIENTED_EDGE('',*,*,#5504,.T.) ;
#7954=ORIENTED_EDGE('',*,*,#5506,.F.) ;
#7955=ORIENTED_EDGE('',*,*,#5507,.F.) ;
#7956=ORIENTED_EDGE('',*,*,#5450,.T.) ;
#7957=ORIENTED_EDGE('',*,*,#5507,.T.) ;
#7958=ORIENTED_EDGE('',*,*,#5508,.F.) ;
#7959=ORIENTED_EDGE('',*,*,#5509,.F.) ;
#7960=ORIENTED_EDGE('',*,*,#5451,.T.) ;
#7961=ORIENTED_EDGE('',*,*,#5509,.T.) ;
#7962=ORIENTED_EDGE('',*,*,#5510,.F.) ;
#7963=ORIENTED_EDGE('',*,*,#5511,.F.) ;
#7964=ORIENTED_EDGE('',*,*,#5452,.T.) ;
#7965=ORIENTED_EDGE('',*,*,#5511,.T.) ;
#7966=ORIENTED_EDGE('',*,*,#5512,.F.) ;
#7967=ORIENTED_EDGE('',*,*,#5513,.F.) ;
#7968=ORIENTED_EDGE('',*,*,#5453,.T.) ;
#7969=ORIENTED_EDGE('',*,*,#5513,.T.) ;
#7970=ORIENTED_EDGE('',*,*,#5514,.F.) ;
#7971=ORIENTED_EDGE('',*,*,#5499,.F.) ;
#7972=ORIENTED_EDGE('',*,*,#5462,.T.) ;
#7973=ORIENTED_EDGE('',*,*,#5515,.T.) ;
#7974=ORIENTED_EDGE('',*,*,#5516,.F.) ;
#7975=ORIENTED_EDGE('',*,*,#5517,.F.) ;
#7976=ORIENTED_EDGE('',*,*,#5463,.T.) ;
#7977=ORIENTED_EDGE('',*,*,#5517,.T.) ;
#7978=ORIENTED_EDGE('',*,*,#5518,.F.) ;
#7979=ORIENTED_EDGE('',*,*,#5519,.F.) ;
#7980=ORIENTED_EDGE('',*,*,#5520,.F.) ;
#7981=ORIENTED_EDGE('',*,*,#5456,.T.) ;
#7982=ORIENTED_EDGE('',*,*,#5519,.T.) ;
#7983=ORIENTED_EDGE('',*,*,#5521,.F.) ;
#7984=ORIENTED_EDGE('',*,*,#5457,.T.) ;
#7985=ORIENTED_EDGE('',*,*,#5520,.T.) ;
#7986=ORIENTED_EDGE('',*,*,#5522,.F.) ;
#7987=ORIENTED_EDGE('',*,*,#5523,.F.) ;
#7988=ORIENTED_EDGE('',*,*,#5458,.T.) ;
#7989=ORIENTED_EDGE('',*,*,#5523,.T.) ;
#7990=ORIENTED_EDGE('',*,*,#5524,.F.) ;
#7991=ORIENTED_EDGE('',*,*,#5525,.F.) ;
#7992=ORIENTED_EDGE('',*,*,#5459,.T.) ;
#7993=ORIENTED_EDGE('',*,*,#5525,.T.) ;
#7994=ORIENTED_EDGE('',*,*,#5526,.F.) ;
#7995=ORIENTED_EDGE('',*,*,#5527,.F.) ;
#7996=ORIENTED_EDGE('',*,*,#5460,.T.) ;
#7997=ORIENTED_EDGE('',*,*,#5527,.T.) ;
#7998=ORIENTED_EDGE('',*,*,#5528,.F.) ;
#7999=ORIENTED_EDGE('',*,*,#5529,.F.) ;
#8000=ORIENTED_EDGE('',*,*,#5461,.T.) ;
#8001=ORIENTED_EDGE('',*,*,#5529,.T.) ;
#8002=ORIENTED_EDGE('',*,*,#5530,.F.) ;
#8003=ORIENTED_EDGE('',*,*,#5515,.F.) ;
#8004=ORIENTED_EDGE('',*,*,#5470,.T.) ;
#8005=ORIENTED_EDGE('',*,*,#5531,.T.) ;
#8006=ORIENTED_EDGE('',*,*,#5532,.F.) ;
#8007=ORIENTED_EDGE('',*,*,#5533,.F.) ;
#8008=ORIENTED_EDGE('',*,*,#5471,.T.) ;
#8009=ORIENTED_EDGE('',*,*,#5533,.T.) ;
#8010=ORIENTED_EDGE('',*,*,#5534,.F.) ;
#8011=ORIENTED_EDGE('',*,*,#5535,.F.) ;
#8012=ORIENTED_EDGE('',*,*,#5536,.F.) ;
#8013=ORIENTED_EDGE('',*,*,#5464,.T.) ;
#8014=ORIENTED_EDGE('',*,*,#5535,.T.) ;
#8015=ORIENTED_EDGE('',*,*,#5537,.F.) ;
#8016=ORIENTED_EDGE('',*,*,#5465,.T.) ;
#8017=ORIENTED_EDGE('',*,*,#5536,.T.) ;
#8018=ORIENTED_EDGE('',*,*,#5538,.F.) ;
#8019=ORIENTED_EDGE('',*,*,#5539,.F.) ;
#8020=ORIENTED_EDGE('',*,*,#5466,.T.) ;
#8021=ORIENTED_EDGE('',*,*,#5539,.T.) ;
#8022=ORIENTED_EDGE('',*,*,#5540,.F.) ;
#8023=ORIENTED_EDGE('',*,*,#5541,.F.) ;
#8024=ORIENTED_EDGE('',*,*,#5467,.T.) ;
#8025=ORIENTED_EDGE('',*,*,#5541,.T.) ;
#8026=ORIENTED_EDGE('',*,*,#5542,.F.) ;
#8027=ORIENTED_EDGE('',*,*,#5543,.F.) ;
#8028=ORIENTED_EDGE('',*,*,#5468,.T.) ;
#8029=ORIENTED_EDGE('',*,*,#5543,.T.) ;
#8030=ORIENTED_EDGE('',*,*,#5544,.F.) ;
#8031=ORIENTED_EDGE('',*,*,#5545,.F.) ;
#8032=ORIENTED_EDGE('',*,*,#5469,.T.) ;
#8033=ORIENTED_EDGE('',*,*,#5545,.T.) ;
#8034=ORIENTED_EDGE('',*,*,#5546,.F.) ;
#8035=ORIENTED_EDGE('',*,*,#5531,.F.) ;
#8036=ORIENTED_EDGE('',*,*,#5478,.T.) ;
#8037=ORIENTED_EDGE('',*,*,#5547,.T.) ;
#8038=ORIENTED_EDGE('',*,*,#5548,.F.) ;
#8039=ORIENTED_EDGE('',*,*,#5549,.F.) ;
#8040=ORIENTED_EDGE('',*,*,#5479,.T.) ;
#8041=ORIENTED_EDGE('',*,*,#5549,.T.) ;
#8042=ORIENTED_EDGE('',*,*,#5550,.F.) ;
#8043=ORIENTED_EDGE('',*,*,#5551,.F.) ;
#8044=ORIENTED_EDGE('',*,*,#5552,.F.) ;
#8045=ORIENTED_EDGE('',*,*,#5472,.T.) ;
#8046=ORIENTED_EDGE('',*,*,#5551,.T.) ;
#8047=ORIENTED_EDGE('',*,*,#5553,.F.) ;
#8048=ORIENTED_EDGE('',*,*,#5473,.T.) ;
#8049=ORIENTED_EDGE('',*,*,#5552,.T.) ;
#8050=ORIENTED_EDGE('',*,*,#5554,.F.) ;
#8051=ORIENTED_EDGE('',*,*,#5555,.F.) ;
#8052=ORIENTED_EDGE('',*,*,#5474,.T.) ;
#8053=ORIENTED_EDGE('',*,*,#5555,.T.) ;
#8054=ORIENTED_EDGE('',*,*,#5556,.F.) ;
#8055=ORIENTED_EDGE('',*,*,#5557,.F.) ;
#8056=ORIENTED_EDGE('',*,*,#5475,.T.) ;
#8057=ORIENTED_EDGE('',*,*,#5557,.T.) ;
#8058=ORIENTED_EDGE('',*,*,#5558,.F.) ;
#8059=ORIENTED_EDGE('',*,*,#5559,.F.) ;
#8060=ORIENTED_EDGE('',*,*,#5476,.T.) ;
#8061=ORIENTED_EDGE('',*,*,#5559,.T.) ;
#8062=ORIENTED_EDGE('',*,*,#5560,.F.) ;
#8063=ORIENTED_EDGE('',*,*,#5561,.F.) ;
#8064=ORIENTED_EDGE('',*,*,#5477,.T.) ;
#8065=ORIENTED_EDGE('',*,*,#5561,.T.) ;
#8066=ORIENTED_EDGE('',*,*,#5562,.F.) ;
#8067=ORIENTED_EDGE('',*,*,#5547,.F.) ;
#8068=ORIENTED_EDGE('',*,*,#5480,.F.) ;
#8069=ORIENTED_EDGE('',*,*,#5563,.T.) ;
#8070=ORIENTED_EDGE('',*,*,#5564,.F.) ;
#8071=ORIENTED_EDGE('',*,*,#5563,.F.) ;
#8072=ORIENTED_EDGE('',*,*,#5565,.F.) ;
#8073=ORIENTED_EDGE('',*,*,#5566,.T.) ;
#8074=ORIENTED_EDGE('',*,*,#5567,.F.) ;
#8075=ORIENTED_EDGE('',*,*,#5566,.F.) ;
#8076=ORIENTED_EDGE('',*,*,#5564,.T.) ;
#8077=ORIENTED_EDGE('',*,*,#5565,.T.) ;
#8078=ORIENTED_EDGE('',*,*,#5567,.T.) ;
#8079=ORIENTED_EDGE('',*,*,#5496,.T.) ;
#8080=ORIENTED_EDGE('',*,*,#5494,.T.) ;
#8081=ORIENTED_EDGE('',*,*,#5492,.T.) ;
#8082=ORIENTED_EDGE('',*,*,#5490,.T.) ;
#8083=ORIENTED_EDGE('',*,*,#5488,.T.) ;
#8084=ORIENTED_EDGE('',*,*,#5487,.T.) ;
#8085=ORIENTED_EDGE('',*,*,#5484,.T.) ;
#8086=ORIENTED_EDGE('',*,*,#5482,.T.) ;
#8087=ORIENTED_EDGE('',*,*,#5497,.T.) ;
#8088=ORIENTED_EDGE('',*,*,#5514,.T.) ;
#8089=ORIENTED_EDGE('',*,*,#5512,.T.) ;
#8090=ORIENTED_EDGE('',*,*,#5510,.T.) ;
#8091=ORIENTED_EDGE('',*,*,#5508,.T.) ;
#8092=ORIENTED_EDGE('',*,*,#5506,.T.) ;
#8093=ORIENTED_EDGE('',*,*,#5505,.T.) ;
#8094=ORIENTED_EDGE('',*,*,#5502,.T.) ;
#8095=ORIENTED_EDGE('',*,*,#5500,.T.) ;
#8096=ORIENTED_EDGE('',*,*,#5530,.T.) ;
#8097=ORIENTED_EDGE('',*,*,#5528,.T.) ;
#8098=ORIENTED_EDGE('',*,*,#5526,.T.) ;
#8099=ORIENTED_EDGE('',*,*,#5524,.T.) ;
#8100=ORIENTED_EDGE('',*,*,#5522,.T.) ;
#8101=ORIENTED_EDGE('',*,*,#5521,.T.) ;
#8102=ORIENTED_EDGE('',*,*,#5518,.T.) ;
#8103=ORIENTED_EDGE('',*,*,#5516,.T.) ;
#8104=ORIENTED_EDGE('',*,*,#5546,.T.) ;
#8105=ORIENTED_EDGE('',*,*,#5544,.T.) ;
#8106=ORIENTED_EDGE('',*,*,#5542,.T.) ;
#8107=ORIENTED_EDGE('',*,*,#5540,.T.) ;
#8108=ORIENTED_EDGE('',*,*,#5538,.T.) ;
#8109=ORIENTED_EDGE('',*,*,#5537,.T.) ;
#8110=ORIENTED_EDGE('',*,*,#5534,.T.) ;
#8111=ORIENTED_EDGE('',*,*,#5532,.T.) ;
#8112=ORIENTED_EDGE('',*,*,#5562,.T.) ;
#8113=ORIENTED_EDGE('',*,*,#5560,.T.) ;
#8114=ORIENTED_EDGE('',*,*,#5558,.T.) ;
#8115=ORIENTED_EDGE('',*,*,#5556,.T.) ;
#8116=ORIENTED_EDGE('',*,*,#5554,.T.) ;
#8117=ORIENTED_EDGE('',*,*,#5553,.T.) ;
#8118=ORIENTED_EDGE('',*,*,#5550,.T.) ;
#8119=ORIENTED_EDGE('',*,*,#5548,.T.) ;
#8209=CYLINDRICAL_SURFACE('',#9375,17.4999999999914) ;
#8210=CYLINDRICAL_SURFACE('',#9377,2.49999999999958) ;
#8211=CYLINDRICAL_SURFACE('',#9380,2.50000000000016) ;
#8212=CYLINDRICAL_SURFACE('',#9382,78.9146368237) ;
#8213=CYLINDRICAL_SURFACE('',#9384,2.50000000000029) ;
#8214=CYLINDRICAL_SURFACE('',#9387,2.50000000000002) ;
#8215=CYLINDRICAL_SURFACE('',#9389,8.00000000000007) ;
#8216=CYLINDRICAL_SURFACE('',#9391,17.4999999999863) ;
#8217=CYLINDRICAL_SURFACE('',#9393,2.50000000000002) ;
#8218=CYLINDRICAL_SURFACE('',#9396,2.50000000000046) ;
#8219=CYLINDRICAL_SURFACE('',#9398,78.9146368237003) ;
#8220=CYLINDRICAL_SURFACE('',#9400,2.50000000000052) ;
#8221=CYLINDRICAL_SURFACE('',#9403,2.49999999999964) ;
#8222=CYLINDRICAL_SURFACE('',#9405,17.4999999999883) ;
#8223=CYLINDRICAL_SURFACE('',#9407,2.49999999999957) ;
#8224=CYLINDRICAL_SURFACE('',#9410,2.50000000000006) ;
#8225=CYLINDRICAL_SURFACE('',#9412,78.9146368237002) ;
#8226=CYLINDRICAL_SURFACE('',#9414,2.50000000000021) ;
#8227=CYLINDRICAL_SURFACE('',#9417,2.49999999999936) ;
#8228=CYLINDRICAL_SURFACE('',#9419,17.4999999999923) ;
#8229=CYLINDRICAL_SURFACE('',#9421,2.49999999999936) ;
#8230=CYLINDRICAL_SURFACE('',#9424,2.5000000000007) ;
#8231=CYLINDRICAL_SURFACE('',#9426,78.9146368237008) ;
#8232=CYLINDRICAL_SURFACE('',#9428,2.50000000000029) ;
#8233=CYLINDRICAL_SURFACE('',#9431,2.49999999999924) ;
#8234=CYLINDRICAL_SURFACE('',#9433,17.4999999999921) ;
#8235=CYLINDRICAL_SURFACE('',#9435,2.49999999999967) ;
#8236=CYLINDRICAL_SURFACE('',#9438,2.50000000000017) ;
#8237=CYLINDRICAL_SURFACE('',#9440,78.9146368237003) ;
#8238=CYLINDRICAL_SURFACE('',#9442,2.49999999999996) ;
#8239=CYLINDRICAL_SURFACE('',#9445,2.499999999999) ;
#8240=CYLINDRICAL_SURFACE('',#9447,83.3146368237019) ;
#8241=CYLINDRICAL_SURFACE('',#9449,81.1146368237021) ;
#8488=ADVANCED_FACE('',(#1105),#420,.T.) ;
#8489=ADVANCED_FACE('',(#1106),#71,.T.) ;
#8490=ADVANCED_FACE('',(#1107),#421,.T.) ;
#8491=ADVANCED_FACE('',(#1108),#422,.T.) ;
#8492=ADVANCED_FACE('',(#1109),#72,.T.) ;
#8493=ADVANCED_FACE('',(#1110),#423,.T.) ;
#8494=ADVANCED_FACE('',(#1111),#424,.T.) ;
#8495=ADVANCED_FACE('',(#1112),#73,.T.) ;
#8496=ADVANCED_FACE('',(#1113),#425,.T.) ;
#8497=ADVANCED_FACE('',(#1114),#426,.T.) ;
#8498=ADVANCED_FACE('',(#1115),#74,.T.) ;
#8499=ADVANCED_FACE('',(#1116),#427,.T.) ;
#8500=ADVANCED_FACE('',(#1117),#428,.T.) ;
#8501=ADVANCED_FACE('',(#1118),#75,.T.) ;
#8502=ADVANCED_FACE('',(#1119),#429,.T.) ;
#8503=ADVANCED_FACE('',(#1120),#430,.T.) ;
#8504=ADVANCED_FACE('',(#1121),#76,.T.) ;
#8505=ADVANCED_FACE('',(#1122),#431,.T.) ;
#8506=ADVANCED_FACE('',(#1123),#432,.T.) ;
#8507=ADVANCED_FACE('',(#1124),#77,.T.) ;
#8508=ADVANCED_FACE('',(#1125),#433,.T.) ;
#8509=ADVANCED_FACE('',(#1126),#434,.T.) ;
#8510=ADVANCED_FACE('',(#1127),#78,.T.) ;
#8511=ADVANCED_FACE('',(#1128),#435,.T.) ;
#8512=ADVANCED_FACE('',(#1129),#436,.T.) ;
#8513=ADVANCED_FACE('',(#1130),#79,.T.) ;
#8514=ADVANCED_FACE('',(#1131),#437,.T.) ;
#8515=ADVANCED_FACE('',(#1132),#438,.T.) ;
#8516=ADVANCED_FACE('',(#1133),#80,.T.) ;
#8517=ADVANCED_FACE('',(#1134),#439,.T.) ;
#8518=ADVANCED_FACE('',(#1135),#440,.T.) ;
#8519=ADVANCED_FACE('',(#1136),#81,.T.) ;
#8520=ADVANCED_FACE('',(#1137),#441,.T.) ;
#8521=ADVANCED_FACE('',(#1138),#442,.T.) ;
#8522=ADVANCED_FACE('',(#1139),#82,.T.) ;
#8523=ADVANCED_FACE('',(#1140),#443,.T.) ;
#8524=ADVANCED_FACE('',(#1141),#444,.T.) ;
#8525=ADVANCED_FACE('',(#1142),#83,.T.) ;
#8526=ADVANCED_FACE('',(#1143),#445,.T.) ;
#8527=ADVANCED_FACE('',(#1144),#446,.T.) ;
#8528=ADVANCED_FACE('',(#1145),#84,.T.) ;
#8529=ADVANCED_FACE('',(#1146),#447,.T.) ;
#8530=ADVANCED_FACE('',(#1147),#448,.T.) ;
#8531=ADVANCED_FACE('',(#1148),#85,.T.) ;
#8532=ADVANCED_FACE('',(#1149),#449,.T.) ;
#8533=ADVANCED_FACE('',(#1150),#450,.T.) ;
#8534=ADVANCED_FACE('',(#1151),#86,.T.) ;
#8535=ADVANCED_FACE('',(#1152),#451,.T.) ;
#8536=ADVANCED_FACE('',(#1153),#452,.T.) ;
#8537=ADVANCED_FACE('',(#1154),#87,.T.) ;
#8538=ADVANCED_FACE('',(#1155),#453,.T.) ;
#8539=ADVANCED_FACE('',(#1156),#454,.T.) ;
#8540=ADVANCED_FACE('',(#1157),#88,.T.) ;
#8541=ADVANCED_FACE('',(#1158),#455,.T.) ;
#8542=ADVANCED_FACE('',(#1159),#456,.T.) ;
#8543=ADVANCED_FACE('',(#1160),#89,.T.) ;
#8544=ADVANCED_FACE('',(#1161),#457,.T.) ;
#8545=ADVANCED_FACE('',(#1162),#458,.T.) ;
#8546=ADVANCED_FACE('',(#1163),#90,.T.) ;
#8547=ADVANCED_FACE('',(#1164),#459,.T.) ;
#8548=ADVANCED_FACE('',(#1165),#460,.T.) ;
#8549=ADVANCED_FACE('',(#1166),#91,.T.) ;
#8550=ADVANCED_FACE('',(#1167),#461,.T.) ;
#8551=ADVANCED_FACE('',(#1168),#462,.T.) ;
#8552=ADVANCED_FACE('',(#1169),#92,.T.) ;
#8553=ADVANCED_FACE('',(#1170),#463,.T.) ;
#8554=ADVANCED_FACE('',(#1171),#464,.T.) ;
#8555=ADVANCED_FACE('',(#1172),#93,.T.) ;
#8556=ADVANCED_FACE('',(#1173),#465,.T.) ;
#8557=ADVANCED_FACE('',(#1174),#466,.T.) ;
#8558=ADVANCED_FACE('',(#1175),#94,.T.) ;
#8559=ADVANCED_FACE('',(#1176),#467,.T.) ;
#8560=ADVANCED_FACE('',(#1177),#468,.T.) ;
#8561=ADVANCED_FACE('',(#1178),#95,.T.) ;
#8562=ADVANCED_FACE('',(#1179),#469,.T.) ;
#8563=ADVANCED_FACE('',(#1180),#470,.T.) ;
#8564=ADVANCED_FACE('',(#1181),#96,.T.) ;
#8565=ADVANCED_FACE('',(#1182),#471,.T.) ;
#8566=ADVANCED_FACE('',(#1183),#472,.T.) ;
#8567=ADVANCED_FACE('',(#1184),#97,.T.) ;
#8568=ADVANCED_FACE('',(#1185),#473,.T.) ;
#8569=ADVANCED_FACE('',(#1186),#474,.T.) ;
#8570=ADVANCED_FACE('',(#1187),#98,.T.) ;
#8571=ADVANCED_FACE('',(#1188),#475,.T.) ;
#8572=ADVANCED_FACE('',(#1189),#476,.T.) ;
#8573=ADVANCED_FACE('',(#1190),#99,.T.) ;
#8574=ADVANCED_FACE('',(#1191),#477,.T.) ;
#8575=ADVANCED_FACE('',(#1192),#478,.T.) ;
#8576=ADVANCED_FACE('',(#1193),#100,.T.) ;
#8577=ADVANCED_FACE('',(#1194),#479,.T.) ;
#8578=ADVANCED_FACE('',(#1195),#480,.T.) ;
#8579=ADVANCED_FACE('',(#1196),#101,.T.) ;
#8580=ADVANCED_FACE('',(#1197),#481,.T.) ;
#8581=ADVANCED_FACE('',(#1198),#482,.T.) ;
#8582=ADVANCED_FACE('',(#1199),#102,.T.) ;
#8583=ADVANCED_FACE('',(#1200),#483,.T.) ;
#8584=ADVANCED_FACE('',(#1201),#484,.T.) ;
#8585=ADVANCED_FACE('',(#1202),#103,.T.) ;
#8586=ADVANCED_FACE('',(#1203),#485,.T.) ;
#8587=ADVANCED_FACE('',(#1204),#486,.T.) ;
#8588=ADVANCED_FACE('',(#1205),#104,.T.) ;
#8589=ADVANCED_FACE('',(#1206),#487,.T.) ;
#8590=ADVANCED_FACE('',(#1207),#488,.T.) ;
#8591=ADVANCED_FACE('',(#1208),#105,.T.) ;
#8592=ADVANCED_FACE('',(#1209),#489,.T.) ;
#8593=ADVANCED_FACE('',(#1210),#490,.T.) ;
#8594=ADVANCED_FACE('',(#1211),#106,.T.) ;
#8595=ADVANCED_FACE('',(#1212),#491,.T.) ;
#8596=ADVANCED_FACE('',(#1213),#492,.T.) ;
#8597=ADVANCED_FACE('',(#1214),#107,.T.) ;
#8598=ADVANCED_FACE('',(#1215),#493,.T.) ;
#8599=ADVANCED_FACE('',(#1216),#494,.T.) ;
#8600=ADVANCED_FACE('',(#1217),#108,.T.) ;
#8601=ADVANCED_FACE('',(#1218),#495,.T.) ;
#8602=ADVANCED_FACE('',(#1219),#496,.T.) ;
#8603=ADVANCED_FACE('',(#1220),#109,.T.) ;
#8604=ADVANCED_FACE('',(#1221),#497,.T.) ;
#8605=ADVANCED_FACE('',(#1222),#498,.T.) ;
#8606=ADVANCED_FACE('',(#1223),#110,.T.) ;
#8607=ADVANCED_FACE('',(#1224),#499,.T.) ;
#8608=ADVANCED_FACE('',(#1225),#500,.T.) ;
#8609=ADVANCED_FACE('',(#1226),#111,.T.) ;
#8610=ADVANCED_FACE('',(#1227),#501,.T.) ;
#8611=ADVANCED_FACE('',(#1228),#502,.T.) ;
#8612=ADVANCED_FACE('',(#1229),#112,.T.) ;
#8613=ADVANCED_FACE('',(#1230),#503,.T.) ;
#8614=ADVANCED_FACE('',(#1231),#504,.T.) ;
#8615=ADVANCED_FACE('',(#1232),#113,.T.) ;
#8616=ADVANCED_FACE('',(#1233),#505,.T.) ;
#8617=ADVANCED_FACE('',(#1234),#506,.T.) ;
#8618=ADVANCED_FACE('',(#1235),#114,.T.) ;
#8619=ADVANCED_FACE('',(#1236),#507,.T.) ;
#8620=ADVANCED_FACE('',(#1237),#508,.T.) ;
#8621=ADVANCED_FACE('',(#1238),#115,.T.) ;
#8622=ADVANCED_FACE('',(#1239),#509,.T.) ;
#8623=ADVANCED_FACE('',(#1240),#510,.T.) ;
#8624=ADVANCED_FACE('',(#1241),#116,.T.) ;
#8625=ADVANCED_FACE('',(#1242),#511,.T.) ;
#8626=ADVANCED_FACE('',(#1243),#512,.T.) ;
#8627=ADVANCED_FACE('',(#1244),#117,.T.) ;
#8628=ADVANCED_FACE('',(#1245),#513,.T.) ;
#8629=ADVANCED_FACE('',(#1246),#514,.T.) ;
#8630=ADVANCED_FACE('',(#1247),#118,.T.) ;
#8631=ADVANCED_FACE('',(#1248),#515,.T.) ;
#8632=ADVANCED_FACE('',(#1249),#516,.T.) ;
#8633=ADVANCED_FACE('',(#1250),#119,.T.) ;
#8634=ADVANCED_FACE('',(#1251),#517,.T.) ;
#8635=ADVANCED_FACE('',(#1252),#518,.T.) ;
#8636=ADVANCED_FACE('',(#1253),#120,.T.) ;
#8637=ADVANCED_FACE('',(#1254),#519,.T.) ;
#8638=ADVANCED_FACE('',(#1255),#520,.T.) ;
#8639=ADVANCED_FACE('',(#1256),#121,.T.) ;
#8640=ADVANCED_FACE('',(#1257),#521,.T.) ;
#8641=ADVANCED_FACE('',(#1258),#522,.T.) ;
#8642=ADVANCED_FACE('',(#1259),#122,.T.) ;
#8643=ADVANCED_FACE('',(#1260),#523,.T.) ;
#8644=ADVANCED_FACE('',(#1261),#524,.T.) ;
#8645=ADVANCED_FACE('',(#1262),#123,.T.) ;
#8646=ADVANCED_FACE('',(#1263),#525,.T.) ;
#8647=ADVANCED_FACE('',(#1264),#526,.T.) ;
#8648=ADVANCED_FACE('',(#1265),#124,.T.) ;
#8649=ADVANCED_FACE('',(#1266),#527,.T.) ;
#8650=ADVANCED_FACE('',(#1267),#528,.T.) ;
#8651=ADVANCED_FACE('',(#1268),#125,.T.) ;
#8652=ADVANCED_FACE('',(#1269),#529,.T.) ;
#8653=ADVANCED_FACE('',(#1270),#530,.T.) ;
#8654=ADVANCED_FACE('',(#1271),#126,.T.) ;
#8655=ADVANCED_FACE('',(#1272),#531,.T.) ;
#8656=ADVANCED_FACE('',(#1273),#532,.T.) ;
#8657=ADVANCED_FACE('',(#1274),#127,.T.) ;
#8658=ADVANCED_FACE('',(#1275),#533,.T.) ;
#8659=ADVANCED_FACE('',(#1276),#534,.T.) ;
#8660=ADVANCED_FACE('',(#1277),#128,.T.) ;
#8661=ADVANCED_FACE('',(#1278),#535,.T.) ;
#8662=ADVANCED_FACE('',(#1279),#536,.T.) ;
#8663=ADVANCED_FACE('',(#1280),#129,.T.) ;
#8664=ADVANCED_FACE('',(#1281),#537,.T.) ;
#8665=ADVANCED_FACE('',(#1282),#538,.T.) ;
#8666=ADVANCED_FACE('',(#1283),#130,.T.) ;
#8667=ADVANCED_FACE('',(#1284),#539,.T.) ;
#8668=ADVANCED_FACE('',(#1285,#598,#599,#600,#601,#602,#603),#540,.T.) ;
#8669=ADVANCED_FACE('',(#1286,#604),#541,.T.) ;
#8670=ADVANCED_FACE('',(#1287),#8209,.T.) ;
#8671=ADVANCED_FACE('',(#1288),#8210,.F.) ;
#8672=ADVANCED_FACE('',(#1289),#542,.T.) ;
#8673=ADVANCED_FACE('',(#1290),#8211,.F.) ;
#8674=ADVANCED_FACE('',(#1291),#8212,.F.) ;
#8675=ADVANCED_FACE('',(#1292),#8213,.F.) ;
#8676=ADVANCED_FACE('',(#1293),#543,.T.) ;
#8677=ADVANCED_FACE('',(#1294),#8214,.F.) ;
#8678=ADVANCED_FACE('',(#1295),#8215,.F.) ;
#8679=ADVANCED_FACE('',(#1296),#8216,.T.) ;
#8680=ADVANCED_FACE('',(#1297),#8217,.F.) ;
#8681=ADVANCED_FACE('',(#1298),#544,.T.) ;
#8682=ADVANCED_FACE('',(#1299),#8218,.F.) ;
#8683=ADVANCED_FACE('',(#1300),#8219,.F.) ;
#8684=ADVANCED_FACE('',(#1301),#8220,.F.) ;
#8685=ADVANCED_FACE('',(#1302),#545,.T.) ;
#8686=ADVANCED_FACE('',(#1303),#8221,.F.) ;
#8687=ADVANCED_FACE('',(#1304),#8222,.T.) ;
#8688=ADVANCED_FACE('',(#1305),#8223,.F.) ;
#8689=ADVANCED_FACE('',(#1306),#546,.T.) ;
#8690=ADVANCED_FACE('',(#1307),#8224,.F.) ;
#8691=ADVANCED_FACE('',(#1308),#8225,.F.) ;
#8692=ADVANCED_FACE('',(#1309),#8226,.F.) ;
#8693=ADVANCED_FACE('',(#1310),#547,.T.) ;
#8694=ADVANCED_FACE('',(#1311),#8227,.F.) ;
#8695=ADVANCED_FACE('',(#1312),#8228,.T.) ;
#8696=ADVANCED_FACE('',(#1313),#8229,.F.) ;
#8697=ADVANCED_FACE('',(#1314),#548,.T.) ;
#8698=ADVANCED_FACE('',(#1315),#8230,.F.) ;
#8699=ADVANCED_FACE('',(#1316),#8231,.F.) ;
#8700=ADVANCED_FACE('',(#1317),#8232,.F.) ;
#8701=ADVANCED_FACE('',(#1318),#549,.T.) ;
#8702=ADVANCED_FACE('',(#1319),#8233,.F.) ;
#8703=ADVANCED_FACE('',(#1320),#8234,.T.) ;
#8704=ADVANCED_FACE('',(#1321),#8235,.F.) ;
#8705=ADVANCED_FACE('',(#1322),#550,.T.) ;
#8706=ADVANCED_FACE('',(#1323),#8236,.F.) ;
#8707=ADVANCED_FACE('',(#1324),#8237,.F.) ;
#8708=ADVANCED_FACE('',(#1325),#8238,.F.) ;
#8709=ADVANCED_FACE('',(#1326),#551,.T.) ;
#8710=ADVANCED_FACE('',(#1327),#8239,.F.) ;
#8711=ADVANCED_FACE('',(#1328),#8240,.F.) ;
#8712=ADVANCED_FACE('',(#1329),#8241,.T.) ;
#8713=ADVANCED_FACE('',(#1330,#605),#552,.T.) ;
#8714=ADVANCED_FACE('',(#1331,#606,#607,#608,#609,#610,#611),#553,.T.) ;
#8733=CLOSED_SHELL('',(#8488,#8489,#8490,#8491,#8492,#8493,#8494,#8495,
#8496,#8497,#8498,#8499,#8500,#8501,#8502,#8503,#8504,#8505,#8506,#8507,
#8508,#8509,#8510,#8511,#8512,#8513,#8514,#8515,#8516,#8517,#8518,#8519,
#8520,#8521,#8522,#8523,#8524,#8525,#8526,#8527,#8528,#8529,#8530,#8531,
#8532,#8533,#8534,#8535,#8536,#8537,#8538,#8539,#8540,#8541,#8542,#8543,
#8544,#8545,#8546,#8547,#8548,#8549,#8550,#8551,#8552,#8553,#8554,#8555,
#8556,#8557,#8558,#8559,#8560,#8561,#8562,#8563,#8564,#8565,#8566,#8567,
#8568,#8569,#8570,#8571,#8572,#8573,#8574,#8575,#8576,#8577,#8578,#8579,
#8580,#8581,#8582,#8583,#8584,#8585,#8586,#8587,#8588,#8589,#8590,#8591,
#8592,#8593,#8594,#8595,#8596,#8597,#8598,#8599,#8600,#8601,#8602,#8603,
#8604,#8605,#8606,#8607,#8608,#8609,#8610,#8611,#8612,#8613,#8614,#8615,
#8616,#8617,#8618,#8619,#8620,#8621,#8622,#8623,#8624,#8625,#8626,#8627,
#8628,#8629,#8630,#8631,#8632,#8633,#8634,#8635,#8636,#8637,#8638,#8639,
#8640,#8641,#8642,#8643,#8644,#8645,#8646,#8647,#8648,#8649,#8650,#8651,
#8652,#8653,#8654,#8655,#8656,#8657,#8658,#8659,#8660,#8661,#8662,#8663,
#8664,#8665,#8666,#8667,#8668,#8669,#8670,#8671,#8672,#8673,#8674,#8675,
#8676,#8677,#8678,#8679,#8680,#8681,#8682,#8683,#8684,#8685,#8686,#8687,
#8688,#8689,#8690,#8691,#8692,#8693,#8694,#8695,#8696,#8697,#8698,#8699,
#8700,#8701,#8702,#8703,#8704,#8705,#8706,#8707,#8708,#8709,#8710,#8711,
#8712,#8713,#8714)) ;
#9101=AXIS2_PLACEMENT_3D('',#194853,#10385,#10386) ;
#9102=AXIS2_PLACEMENT_3D('',#194873,#10391,#10392) ;
#9103=AXIS2_PLACEMENT_3D('',#194876,#10394,#10395) ;
#9104=AXIS2_PLACEMENT_3D('',#194877,#10396,#10397) ;
#9105=AXIS2_PLACEMENT_3D('',#194883,#10401,#10402) ;
#9106=AXIS2_PLACEMENT_3D('',#194900,#10406,#10407) ;
#9107=AXIS2_PLACEMENT_3D('',#194903,#10409,#10410) ;
#9108=AXIS2_PLACEMENT_3D('',#194904,#10411,#10412) ;
#9109=AXIS2_PLACEMENT_3D('',#194910,#10416,#10417) ;
#9110=AXIS2_PLACEMENT_3D('',#194927,#10421,#10422) ;
#9111=AXIS2_PLACEMENT_3D('',#194930,#10424,#10425) ;
#9112=AXIS2_PLACEMENT_3D('',#194931,#10426,#10427) ;
#9113=AXIS2_PLACEMENT_3D('',#194937,#10431,#10432) ;
#9114=AXIS2_PLACEMENT_3D('',#194954,#10436,#10437) ;
#9115=AXIS2_PLACEMENT_3D('',#194957,#10439,#10440) ;
#9116=AXIS2_PLACEMENT_3D('',#194958,#10441,#10442) ;
#9117=AXIS2_PLACEMENT_3D('',#194964,#10446,#10447) ;
#9118=AXIS2_PLACEMENT_3D('',#194981,#10451,#10452) ;
#9119=AXIS2_PLACEMENT_3D('',#194984,#10454,#10455) ;
#9120=AXIS2_PLACEMENT_3D('',#194985,#10456,#10457) ;
#9121=AXIS2_PLACEMENT_3D('',#194991,#10461,#10462) ;
#9122=AXIS2_PLACEMENT_3D('',#195008,#10466,#10467) ;
#9123=AXIS2_PLACEMENT_3D('',#195011,#10469,#10470) ;
#9124=AXIS2_PLACEMENT_3D('',#195012,#10471,#10472) ;
#9125=AXIS2_PLACEMENT_3D('',#195018,#10476,#10477) ;
#9126=AXIS2_PLACEMENT_3D('',#195035,#10481,#10482) ;
#9127=AXIS2_PLACEMENT_3D('',#195038,#10484,#10485) ;
#9128=AXIS2_PLACEMENT_3D('',#195039,#10486,#10487) ;
#9129=AXIS2_PLACEMENT_3D('',#195045,#10491,#10492) ;
#9130=AXIS2_PLACEMENT_3D('',#195062,#10496,#10497) ;
#9131=AXIS2_PLACEMENT_3D('',#195065,#10499,#10500) ;
#9132=AXIS2_PLACEMENT_3D('',#195066,#10501,#10502) ;
#9133=AXIS2_PLACEMENT_3D('',#195072,#10506,#10507) ;
#9134=AXIS2_PLACEMENT_3D('',#195089,#10511,#10512) ;
#9135=AXIS2_PLACEMENT_3D('',#195092,#10514,#10515) ;
#9136=AXIS2_PLACEMENT_3D('',#195093,#10516,#10517) ;
#9137=AXIS2_PLACEMENT_3D('',#195099,#10521,#10522) ;
#9138=AXIS2_PLACEMENT_3D('',#195116,#10526,#10527) ;
#9139=AXIS2_PLACEMENT_3D('',#195119,#10529,#10530) ;
#9140=AXIS2_PLACEMENT_3D('',#195120,#10531,#10532) ;
#9141=AXIS2_PLACEMENT_3D('',#195126,#10536,#10537) ;
#9142=AXIS2_PLACEMENT_3D('',#195143,#10541,#10542) ;
#9143=AXIS2_PLACEMENT_3D('',#195146,#10544,#10545) ;
#9144=AXIS2_PLACEMENT_3D('',#195147,#10546,#10547) ;
#9145=AXIS2_PLACEMENT_3D('',#195153,#10551,#10552) ;
#9146=AXIS2_PLACEMENT_3D('',#195170,#10556,#10557) ;
#9147=AXIS2_PLACEMENT_3D('',#195173,#10559,#10560) ;
#9148=AXIS2_PLACEMENT_3D('',#195174,#10561,#10562) ;
#9149=AXIS2_PLACEMENT_3D('',#195180,#10566,#10567) ;
#9150=AXIS2_PLACEMENT_3D('',#195197,#10571,#10572) ;
#9151=AXIS2_PLACEMENT_3D('',#195200,#10574,#10575) ;
#9152=AXIS2_PLACEMENT_3D('',#195201,#10576,#10577) ;
#9153=AXIS2_PLACEMENT_3D('',#195207,#10581,#10582) ;
#9154=AXIS2_PLACEMENT_3D('',#195224,#10586,#10587) ;
#9155=AXIS2_PLACEMENT_3D('',#195227,#10589,#10590) ;
#9156=AXIS2_PLACEMENT_3D('',#195228,#10591,#10592) ;
#9157=AXIS2_PLACEMENT_3D('',#195234,#10596,#10597) ;
#9158=AXIS2_PLACEMENT_3D('',#195251,#10601,#10602) ;
#9159=AXIS2_PLACEMENT_3D('',#195254,#10604,#10605) ;
#9160=AXIS2_PLACEMENT_3D('',#195255,#10606,#10607) ;
#9161=AXIS2_PLACEMENT_3D('',#195261,#10611,#10612) ;
#9162=AXIS2_PLACEMENT_3D('',#195278,#10616,#10617) ;
#9163=AXIS2_PLACEMENT_3D('',#195281,#10619,#10620) ;
#9164=AXIS2_PLACEMENT_3D('',#195282,#10621,#10622) ;
#9165=AXIS2_PLACEMENT_3D('',#195288,#10626,#10627) ;
#9166=AXIS2_PLACEMENT_3D('',#195305,#10631,#10632) ;
#9167=AXIS2_PLACEMENT_3D('',#195308,#10634,#10635) ;
#9168=AXIS2_PLACEMENT_3D('',#195309,#10636,#10637) ;
#9169=AXIS2_PLACEMENT_3D('',#195315,#10641,#10642) ;
#9170=AXIS2_PLACEMENT_3D('',#195332,#10646,#10647) ;
#9171=AXIS2_PLACEMENT_3D('',#195335,#10649,#10650) ;
#9172=AXIS2_PLACEMENT_3D('',#195336,#10651,#10652) ;
#9173=AXIS2_PLACEMENT_3D('',#195342,#10656,#10657) ;
#9174=AXIS2_PLACEMENT_3D('',#195359,#10661,#10662) ;
#9175=AXIS2_PLACEMENT_3D('',#195362,#10664,#10665) ;
#9176=AXIS2_PLACEMENT_3D('',#195363,#10666,#10667) ;
#9177=AXIS2_PLACEMENT_3D('',#195369,#10671,#10672) ;
#9178=AXIS2_PLACEMENT_3D('',#195386,#10676,#10677) ;
#9179=AXIS2_PLACEMENT_3D('',#195389,#10679,#10680) ;
#9180=AXIS2_PLACEMENT_3D('',#195390,#10681,#10682) ;
#9181=AXIS2_PLACEMENT_3D('',#195396,#10686,#10687) ;
#9182=AXIS2_PLACEMENT_3D('',#195413,#10691,#10692) ;
#9183=AXIS2_PLACEMENT_3D('',#195416,#10694,#10695) ;
#9184=AXIS2_PLACEMENT_3D('',#195417,#10696,#10697) ;
#9185=AXIS2_PLACEMENT_3D('',#195423,#10701,#10702) ;
#9186=AXIS2_PLACEMENT_3D('',#195440,#10706,#10707) ;
#9187=AXIS2_PLACEMENT_3D('',#195443,#10709,#10710) ;
#9188=AXIS2_PLACEMENT_3D('',#195444,#10711,#10712) ;
#9189=AXIS2_PLACEMENT_3D('',#195450,#10716,#10717) ;
#9190=AXIS2_PLACEMENT_3D('',#195467,#10721,#10722) ;
#9191=AXIS2_PLACEMENT_3D('',#195470,#10724,#10725) ;
#9192=AXIS2_PLACEMENT_3D('',#195471,#10726,#10727) ;
#9193=AXIS2_PLACEMENT_3D('',#195477,#10731,#10732) ;
#9194=AXIS2_PLACEMENT_3D('',#195494,#10736,#10737) ;
#9195=AXIS2_PLACEMENT_3D('',#195497,#10739,#10740) ;
#9196=AXIS2_PLACEMENT_3D('',#195498,#10741,#10742) ;
#9197=AXIS2_PLACEMENT_3D('',#195504,#10746,#10747) ;
#9198=AXIS2_PLACEMENT_3D('',#195521,#10751,#10752) ;
#9199=AXIS2_PLACEMENT_3D('',#195524,#10754,#10755) ;
#9200=AXIS2_PLACEMENT_3D('',#195525,#10756,#10757) ;
#9201=AXIS2_PLACEMENT_3D('',#195531,#10761,#10762) ;
#9202=AXIS2_PLACEMENT_3D('',#195548,#10766,#10767) ;
#9203=AXIS2_PLACEMENT_3D('',#195551,#10769,#10770) ;
#9204=AXIS2_PLACEMENT_3D('',#195552,#10771,#10772) ;
#9205=AXIS2_PLACEMENT_3D('',#195558,#10776,#10777) ;
#9206=AXIS2_PLACEMENT_3D('',#195575,#10781,#10782) ;
#9207=AXIS2_PLACEMENT_3D('',#195578,#10784,#10785) ;
#9208=AXIS2_PLACEMENT_3D('',#195579,#10786,#10787) ;
#9209=AXIS2_PLACEMENT_3D('',#195585,#10791,#10792) ;
#9210=AXIS2_PLACEMENT_3D('',#195602,#10796,#10797) ;
#9211=AXIS2_PLACEMENT_3D('',#195605,#10799,#10800) ;
#9212=AXIS2_PLACEMENT_3D('',#195606,#10801,#10802) ;
#9213=AXIS2_PLACEMENT_3D('',#195612,#10806,#10807) ;
#9214=AXIS2_PLACEMENT_3D('',#195629,#10811,#10812) ;
#9215=AXIS2_PLACEMENT_3D('',#195632,#10814,#10815) ;
#9216=AXIS2_PLACEMENT_3D('',#195633,#10816,#10817) ;
#9217=AXIS2_PLACEMENT_3D('',#195639,#10821,#10822) ;
#9218=AXIS2_PLACEMENT_3D('',#195656,#10826,#10827) ;
#9219=AXIS2_PLACEMENT_3D('',#195659,#10829,#10830) ;
#9220=AXIS2_PLACEMENT_3D('',#195660,#10831,#10832) ;
#9221=AXIS2_PLACEMENT_3D('',#195666,#10836,#10837) ;
#9222=AXIS2_PLACEMENT_3D('',#195683,#10841,#10842) ;
#9223=AXIS2_PLACEMENT_3D('',#195686,#10844,#10845) ;
#9224=AXIS2_PLACEMENT_3D('',#195687,#10846,#10847) ;
#9225=AXIS2_PLACEMENT_3D('',#195693,#10851,#10852) ;
#9226=AXIS2_PLACEMENT_3D('',#195710,#10856,#10857) ;
#9227=AXIS2_PLACEMENT_3D('',#195713,#10859,#10860) ;
#9228=AXIS2_PLACEMENT_3D('',#195714,#10861,#10862) ;
#9229=AXIS2_PLACEMENT_3D('',#195720,#10866,#10867) ;
#9230=AXIS2_PLACEMENT_3D('',#195737,#10871,#10872) ;
#9231=AXIS2_PLACEMENT_3D('',#195740,#10874,#10875) ;
#9232=AXIS2_PLACEMENT_3D('',#195741,#10876,#10877) ;
#9233=AXIS2_PLACEMENT_3D('',#195747,#10881,#10882) ;
#9234=AXIS2_PLACEMENT_3D('',#195764,#10886,#10887) ;
#9235=AXIS2_PLACEMENT_3D('',#195767,#10889,#10890) ;
#9236=AXIS2_PLACEMENT_3D('',#195768,#10891,#10892) ;
#9237=AXIS2_PLACEMENT_3D('',#195774,#10896,#10897) ;
#9238=AXIS2_PLACEMENT_3D('',#195791,#10901,#10902) ;
#9239=AXIS2_PLACEMENT_3D('',#195794,#10904,#10905) ;
#9240=AXIS2_PLACEMENT_3D('',#195795,#10906,#10907) ;
#9241=AXIS2_PLACEMENT_3D('',#195801,#10911,#10912) ;
#9242=AXIS2_PLACEMENT_3D('',#195818,#10916,#10917) ;
#9243=AXIS2_PLACEMENT_3D('',#195821,#10919,#10920) ;
#9244=AXIS2_PLACEMENT_3D('',#195822,#10921,#10922) ;
#9245=AXIS2_PLACEMENT_3D('',#195828,#10926,#10927) ;
#9246=AXIS2_PLACEMENT_3D('',#195845,#10931,#10932) ;
#9247=AXIS2_PLACEMENT_3D('',#195848,#10934,#10935) ;
#9248=AXIS2_PLACEMENT_3D('',#195849,#10936,#10937) ;
#9249=AXIS2_PLACEMENT_3D('',#195855,#10941,#10942) ;
#9250=AXIS2_PLACEMENT_3D('',#195872,#10946,#10947) ;
#9251=AXIS2_PLACEMENT_3D('',#195875,#10949,#10950) ;
#9252=AXIS2_PLACEMENT_3D('',#195876,#10951,#10952) ;
#9253=AXIS2_PLACEMENT_3D('',#195882,#10956,#10957) ;
#9254=AXIS2_PLACEMENT_3D('',#195899,#10961,#10962) ;
#9255=AXIS2_PLACEMENT_3D('',#195902,#10964,#10965) ;
#9256=AXIS2_PLACEMENT_3D('',#195903,#10966,#10967) ;
#9257=AXIS2_PLACEMENT_3D('',#195909,#10971,#10972) ;
#9258=AXIS2_PLACEMENT_3D('',#195926,#10976,#10977) ;
#9259=AXIS2_PLACEMENT_3D('',#195929,#10979,#10980) ;
#9260=AXIS2_PLACEMENT_3D('',#195930,#10981,#10982) ;
#9261=AXIS2_PLACEMENT_3D('',#195936,#10986,#10987) ;
#9262=AXIS2_PLACEMENT_3D('',#195953,#10991,#10992) ;
#9263=AXIS2_PLACEMENT_3D('',#195956,#10994,#10995) ;
#9264=AXIS2_PLACEMENT_3D('',#195957,#10996,#10997) ;
#9265=AXIS2_PLACEMENT_3D('',#195963,#11001,#11002) ;
#9266=AXIS2_PLACEMENT_3D('',#195980,#11006,#11007) ;
#9267=AXIS2_PLACEMENT_3D('',#195983,#11009,#11010) ;
#9268=AXIS2_PLACEMENT_3D('',#195984,#11011,#11012) ;
#9269=AXIS2_PLACEMENT_3D('',#195990,#11016,#11017) ;
#9270=AXIS2_PLACEMENT_3D('',#196007,#11021,#11022) ;
#9271=AXIS2_PLACEMENT_3D('',#196010,#11024,#11025) ;
#9272=AXIS2_PLACEMENT_3D('',#196011,#11026,#11027) ;
#9273=AXIS2_PLACEMENT_3D('',#196017,#11031,#11032) ;
#9274=AXIS2_PLACEMENT_3D('',#196034,#11036,#11037) ;
#9275=AXIS2_PLACEMENT_3D('',#196037,#11039,#11040) ;
#9276=AXIS2_PLACEMENT_3D('',#196038,#11041,#11042) ;
#9277=AXIS2_PLACEMENT_3D('',#196044,#11046,#11047) ;
#9278=AXIS2_PLACEMENT_3D('',#196061,#11051,#11052) ;
#9279=AXIS2_PLACEMENT_3D('',#196064,#11054,#11055) ;
#9280=AXIS2_PLACEMENT_3D('',#196065,#11056,#11057) ;
#9281=AXIS2_PLACEMENT_3D('',#196071,#11061,#11062) ;
#9282=AXIS2_PLACEMENT_3D('',#196088,#11066,#11067) ;
#9283=AXIS2_PLACEMENT_3D('',#196091,#11069,#11070) ;
#9284=AXIS2_PLACEMENT_3D('',#196092,#11071,#11072) ;
#9285=AXIS2_PLACEMENT_3D('',#196098,#11076,#11077) ;
#9286=AXIS2_PLACEMENT_3D('',#196115,#11081,#11082) ;
#9287=AXIS2_PLACEMENT_3D('',#196118,#11084,#11085) ;
#9288=AXIS2_PLACEMENT_3D('',#196119,#11086,#11087) ;
#9289=AXIS2_PLACEMENT_3D('',#196125,#11091,#11092) ;
#9290=AXIS2_PLACEMENT_3D('',#196142,#11096,#11097) ;
#9291=AXIS2_PLACEMENT_3D('',#196145,#11099,#11100) ;
#9292=AXIS2_PLACEMENT_3D('',#196146,#11101,#11102) ;
#9293=AXIS2_PLACEMENT_3D('',#196152,#11106,#11107) ;
#9294=AXIS2_PLACEMENT_3D('',#196169,#11111,#11112) ;
#9295=AXIS2_PLACEMENT_3D('',#196172,#11114,#11115) ;
#9296=AXIS2_PLACEMENT_3D('',#196173,#11116,#11117) ;
#9297=AXIS2_PLACEMENT_3D('',#196179,#11121,#11122) ;
#9298=AXIS2_PLACEMENT_3D('',#196196,#11126,#11127) ;
#9299=AXIS2_PLACEMENT_3D('',#196199,#11129,#11130) ;
#9300=AXIS2_PLACEMENT_3D('',#196200,#11131,#11132) ;
#9301=AXIS2_PLACEMENT_3D('',#196206,#11136,#11137) ;
#9302=AXIS2_PLACEMENT_3D('',#196223,#11141,#11142) ;
#9303=AXIS2_PLACEMENT_3D('',#196226,#11144,#11145) ;
#9304=AXIS2_PLACEMENT_3D('',#196227,#11146,#11147) ;
#9305=AXIS2_PLACEMENT_3D('',#196233,#11151,#11152) ;
#9306=AXIS2_PLACEMENT_3D('',#196250,#11156,#11157) ;
#9307=AXIS2_PLACEMENT_3D('',#196253,#11159,#11160) ;
#9308=AXIS2_PLACEMENT_3D('',#196254,#11161,#11162) ;
#9309=AXIS2_PLACEMENT_3D('',#196260,#11166,#11167) ;
#9310=AXIS2_PLACEMENT_3D('',#196277,#11171,#11172) ;
#9311=AXIS2_PLACEMENT_3D('',#196280,#11174,#11175) ;
#9312=AXIS2_PLACEMENT_3D('',#196281,#11176,#11177) ;
#9313=AXIS2_PLACEMENT_3D('',#196287,#11181,#11182) ;
#9314=AXIS2_PLACEMENT_3D('',#196304,#11186,#11187) ;
#9315=AXIS2_PLACEMENT_3D('',#196307,#11189,#11190) ;
#9316=AXIS2_PLACEMENT_3D('',#196308,#11191,#11192) ;
#9317=AXIS2_PLACEMENT_3D('',#196314,#11196,#11197) ;
#9318=AXIS2_PLACEMENT_3D('',#196331,#11201,#11202) ;
#9319=AXIS2_PLACEMENT_3D('',#196334,#11204,#11205) ;
#9320=AXIS2_PLACEMENT_3D('',#196335,#11206,#11207) ;
#9321=AXIS2_PLACEMENT_3D('',#196341,#11211,#11212) ;
#9322=AXIS2_PLACEMENT_3D('',#196358,#11216,#11217) ;
#9323=AXIS2_PLACEMENT_3D('',#196361,#11219,#11220) ;
#9324=AXIS2_PLACEMENT_3D('',#196362,#11221,#11222) ;
#9325=AXIS2_PLACEMENT_3D('',#196368,#11226,#11227) ;
#9326=AXIS2_PLACEMENT_3D('',#196385,#11231,#11232) ;
#9327=AXIS2_PLACEMENT_3D('',#196388,#11234,#11235) ;
#9328=AXIS2_PLACEMENT_3D('',#196389,#11236,#11237) ;
#9329=AXIS2_PLACEMENT_3D('',#196395,#11241,#11242) ;
#9330=AXIS2_PLACEMENT_3D('',#196412,#11246,#11247) ;
#9331=AXIS2_PLACEMENT_3D('',#196415,#11249,#11250) ;
#9332=AXIS2_PLACEMENT_3D('',#196416,#11251,#11252) ;
#9333=AXIS2_PLACEMENT_3D('',#196422,#11256,#11257) ;
#9334=AXIS2_PLACEMENT_3D('',#196439,#11261,#11262) ;
#9335=AXIS2_PLACEMENT_3D('',#196442,#11264,#11265) ;
#9336=AXIS2_PLACEMENT_3D('',#196443,#11266,#11267) ;
#9337=AXIS2_PLACEMENT_3D('',#196449,#11271,#11272) ;
#9338=AXIS2_PLACEMENT_3D('',#196466,#11276,#11277) ;
#9339=AXIS2_PLACEMENT_3D('',#196469,#11279,#11280) ;
#9340=AXIS2_PLACEMENT_3D('',#196470,#11281,#11282) ;
#9341=AXIS2_PLACEMENT_3D('',#196473,#11285,#11286) ;
#9342=AXIS2_PLACEMENT_3D('',#196478,#11288,#11289) ;
#9343=AXIS2_PLACEMENT_3D('',#196480,#11290,#11291) ;
#9344=AXIS2_PLACEMENT_3D('',#196482,#11292,#11293) ;
#9345=AXIS2_PLACEMENT_3D('',#196486,#11295,#11296) ;
#9346=AXIS2_PLACEMENT_3D('',#196488,#11297,#11298) ;
#9347=AXIS2_PLACEMENT_3D('',#196489,#11299,#11300) ;
#9348=AXIS2_PLACEMENT_3D('',#196491,#11301,#11302) ;
#9349=AXIS2_PLACEMENT_3D('',#196496,#11304,#11305) ;
#9350=AXIS2_PLACEMENT_3D('',#196498,#11306,#11307) ;
#9351=AXIS2_PLACEMENT_3D('',#196500,#11308,#11309) ;
#9352=AXIS2_PLACEMENT_3D('',#196504,#11311,#11312) ;
#9353=AXIS2_PLACEMENT_3D('',#196506,#11313,#11314) ;
#9354=AXIS2_PLACEMENT_3D('',#196507,#11315,#11316) ;
#9355=AXIS2_PLACEMENT_3D('',#196512,#11318,#11319) ;
#9356=AXIS2_PLACEMENT_3D('',#196514,#11320,#11321) ;
#9357=AXIS2_PLACEMENT_3D('',#196516,#11322,#11323) ;
#9358=AXIS2_PLACEMENT_3D('',#196520,#11325,#11326) ;
#9359=AXIS2_PLACEMENT_3D('',#196522,#11327,#11328) ;
#9360=AXIS2_PLACEMENT_3D('',#196523,#11329,#11330) ;
#9361=AXIS2_PLACEMENT_3D('',#196528,#11332,#11333) ;
#9362=AXIS2_PLACEMENT_3D('',#196530,#11334,#11335) ;
#9363=AXIS2_PLACEMENT_3D('',#196532,#11336,#11337) ;
#9364=AXIS2_PLACEMENT_3D('',#196536,#11339,#11340) ;
#9365=AXIS2_PLACEMENT_3D('',#196538,#11341,#11342) ;
#9366=AXIS2_PLACEMENT_3D('',#196539,#11343,#11344) ;
#9367=AXIS2_PLACEMENT_3D('',#196544,#11346,#11347) ;
#9368=AXIS2_PLACEMENT_3D('',#196546,#11348,#11349) ;
#9369=AXIS2_PLACEMENT_3D('',#196548,#11350,#11351) ;
#9370=AXIS2_PLACEMENT_3D('',#196552,#11353,#11354) ;
#9371=AXIS2_PLACEMENT_3D('',#196554,#11355,#11356) ;
#9372=AXIS2_PLACEMENT_3D('',#196555,#11357,#11358) ;
#9373=AXIS2_PLACEMENT_3D('',#196556,#11359,#11360) ;
#9374=AXIS2_PLACEMENT_3D('',#196558,#11361,#11362) ;
#9375=AXIS2_PLACEMENT_3D('',#196559,#11363,#11364) ;
#9376=AXIS2_PLACEMENT_3D('',#196563,#11366,#11367) ;
#9377=AXIS2_PLACEMENT_3D('',#196565,#11369,#11370) ;
#9378=AXIS2_PLACEMENT_3D('',#196567,#11371,#11372) ;
#9379=AXIS2_PLACEMENT_3D('',#196569,#11374,#11375) ;
#9380=AXIS2_PLACEMENT_3D('',#196573,#11378,#11379) ;
#9381=AXIS2_PLACEMENT_3D('',#196575,#11380,#11381) ;
#9382=AXIS2_PLACEMENT_3D('',#196577,#11383,#11384) ;
#9383=AXIS2_PLACEMENT_3D('',#196579,#11385,#11386) ;
#9384=AXIS2_PLACEMENT_3D('',#196581,#11388,#11389) ;
#9385=AXIS2_PLACEMENT_3D('',#196583,#11390,#11391) ;
#9386=AXIS2_PLACEMENT_3D('',#196585,#11393,#11394) ;
#9387=AXIS2_PLACEMENT_3D('',#196589,#11397,#11398) ;
#9388=AXIS2_PLACEMENT_3D('',#196590,#11399,#11400) ;
#9389=AXIS2_PLACEMENT_3D('',#196591,#11401,#11402) ;
#9390=AXIS2_PLACEMENT_3D('',#196593,#11403,#11404) ;
#9391=AXIS2_PLACEMENT_3D('',#196595,#11406,#11407) ;
#9392=AXIS2_PLACEMENT_3D('',#196599,#11409,#11410) ;
#9393=AXIS2_PLACEMENT_3D('',#196601,#11412,#11413) ;
#9394=AXIS2_PLACEMENT_3D('',#196603,#11414,#11415) ;
#9395=AXIS2_PLACEMENT_3D('',#196605,#11417,#11418) ;
#9396=AXIS2_PLACEMENT_3D('',#196609,#11421,#11422) ;
#9397=AXIS2_PLACEMENT_3D('',#196611,#11423,#11424) ;
#9398=AXIS2_PLACEMENT_3D('',#196613,#11426,#11427) ;
#9399=AXIS2_PLACEMENT_3D('',#196615,#11428,#11429) ;
#9400=AXIS2_PLACEMENT_3D('',#196617,#11431,#11432) ;
#9401=AXIS2_PLACEMENT_3D('',#196619,#11433,#11434) ;
#9402=AXIS2_PLACEMENT_3D('',#196621,#11436,#11437) ;
#9403=AXIS2_PLACEMENT_3D('',#196625,#11440,#11441) ;
#9404=AXIS2_PLACEMENT_3D('',#196626,#11442,#11443) ;
#9405=AXIS2_PLACEMENT_3D('',#196627,#11444,#11445) ;
#9406=AXIS2_PLACEMENT_3D('',#196631,#11447,#11448) ;
#9407=AXIS2_PLACEMENT_3D('',#196633,#11450,#11451) ;
#9408=AXIS2_PLACEMENT_3D('',#196635,#11452,#11453) ;
#9409=AXIS2_PLACEMENT_3D('',#196637,#11455,#11456) ;
#9410=AXIS2_PLACEMENT_3D('',#196641,#11459,#11460) ;
#9411=AXIS2_PLACEMENT_3D('',#196643,#11461,#11462) ;
#9412=AXIS2_PLACEMENT_3D('',#196645,#11464,#11465) ;
#9413=AXIS2_PLACEMENT_3D('',#196647,#11466,#11467) ;
#9414=AXIS2_PLACEMENT_3D('',#196649,#11469,#11470) ;
#9415=AXIS2_PLACEMENT_3D('',#196651,#11471,#11472) ;
#9416=AXIS2_PLACEMENT_3D('',#196653,#11474,#11475) ;
#9417=AXIS2_PLACEMENT_3D('',#196657,#11478,#11479) ;
#9418=AXIS2_PLACEMENT_3D('',#196658,#11480,#11481) ;
#9419=AXIS2_PLACEMENT_3D('',#196659,#11482,#11483) ;
#9420=AXIS2_PLACEMENT_3D('',#196663,#11485,#11486) ;
#9421=AXIS2_PLACEMENT_3D('',#196665,#11488,#11489) ;
#9422=AXIS2_PLACEMENT_3D('',#196667,#11490,#11491) ;
#9423=AXIS2_PLACEMENT_3D('',#196669,#11493,#11494) ;
#9424=AXIS2_PLACEMENT_3D('',#196673,#11497,#11498) ;
#9425=AXIS2_PLACEMENT_3D('',#196675,#11499,#11500) ;
#9426=AXIS2_PLACEMENT_3D('',#196677,#11502,#11503) ;
#9427=AXIS2_PLACEMENT_3D('',#196679,#11504,#11505) ;
#9428=AXIS2_PLACEMENT_3D('',#196681,#11507,#11508) ;
#9429=AXIS2_PLACEMENT_3D('',#196683,#11509,#11510) ;
#9430=AXIS2_PLACEMENT_3D('',#196685,#11512,#11513) ;
#9431=AXIS2_PLACEMENT_3D('',#196689,#11516,#11517) ;
#9432=AXIS2_PLACEMENT_3D('',#196690,#11518,#11519) ;
#9433=AXIS2_PLACEMENT_3D('',#196691,#11520,#11521) ;
#9434=AXIS2_PLACEMENT_3D('',#196695,#11523,#11524) ;
#9435=AXIS2_PLACEMENT_3D('',#196697,#11526,#11527) ;
#9436=AXIS2_PLACEMENT_3D('',#196699,#11528,#11529) ;
#9437=AXIS2_PLACEMENT_3D('',#196701,#11531,#11532) ;
#9438=AXIS2_PLACEMENT_3D('',#196705,#11535,#11536) ;
#9439=AXIS2_PLACEMENT_3D('',#196707,#11537,#11538) ;
#9440=AXIS2_PLACEMENT_3D('',#196709,#11540,#11541) ;
#9441=AXIS2_PLACEMENT_3D('',#196711,#11542,#11543) ;
#9442=AXIS2_PLACEMENT_3D('',#196713,#11545,#11546) ;
#9443=AXIS2_PLACEMENT_3D('',#196715,#11547,#11548) ;
#9444=AXIS2_PLACEMENT_3D('',#196717,#11550,#11551) ;
#9445=AXIS2_PLACEMENT_3D('',#196721,#11554,#11555) ;
#9446=AXIS2_PLACEMENT_3D('',#196722,#11556,#11557) ;
#9447=AXIS2_PLACEMENT_3D('',#196723,#11558,#11559) ;
#9448=AXIS2_PLACEMENT_3D('',#196726,#11561,#11562) ;
#9449=AXIS2_PLACEMENT_3D('',#196727,#11563,#11564) ;
#9450=AXIS2_PLACEMENT_3D('',#196729,#11565,#11566) ;
#9451=AXIS2_PLACEMENT_3D('',#196732,#11568,#11569) ;
#9452=AXIS2_PLACEMENT_3D('',#196733,#11570,#11571) ;
#9453=AXIS2_PLACEMENT_3D('',#196734,#11572,#11573) ;
#10385=DIRECTION('center_axis',(0.664443266232236,-6.36113025469821E-15,
0.747338708992541)) ;
#10386=DIRECTION('ref_axis',(0.747338708992541,0.,-0.664443266232236)) ;
#10387=DIRECTION('',(-0.747338708992541,-7.25975707680218E-15,0.664443266232236)) ;
#10388=DIRECTION('',(0.,-1.,-1.03620815631681E-14)) ;
#10389=DIRECTION('',(-0.747338708992547,-6.45311740160199E-15,0.664443266232229)) ;
#10390=DIRECTION('',(0.,-1.,-8.88178419700125E-15)) ;
#10391=DIRECTION('center_axis',(4.66744588567091E-17,1.,1.02423325316423E-14)) ;
#10392=DIRECTION('ref_axis',(0.780900470920595,6.36148092073446E-15,-0.624655468651314)) ;
#10393=DIRECTION('',(0.,-1.,-4.44089209850063E-15)) ;
#10394=DIRECTION('center_axis',(-6.66122276787905E-17,1.,1.00236394903081E-14)) ;
#10395=DIRECTION('ref_axis',(0.780900470920575,6.31333874337391E-15,-0.624655468651339)) ;
#10396=DIRECTION('center_axis',(0.810464275400705,6.12393213561332E-15,
-0.585788066026622)) ;
#10397=DIRECTION('ref_axis',(-0.585788066026622,0.,-0.810464275400705)) ;
#10398=DIRECTION('',(0.585788066026618,-8.18378228936874E-15,0.810464275400708)) ;
#10399=DIRECTION('',(0.,-1.,-1.03620815631681E-14)) ;
#10400=DIRECTION('',(0.585788066026622,-8.1837822893688E-15,0.810464275400705)) ;
#10401=DIRECTION('center_axis',(0.582685209706625,-6.37206611617975E-15,
0.812697942897081)) ;
#10402=DIRECTION('ref_axis',(0.812697942897081,0.,-0.582685209706625)) ;
#10403=DIRECTION('',(-0.812697942896989,-6.4531174016024E-15,0.582685209706753)) ;
#10404=DIRECTION('',(0.,-1.,-1.03620815631681E-14)) ;
#10405=DIRECTION('',(-0.812697942896989,-6.4531174016024E-15,0.582685209706753)) ;
#10406=DIRECTION('center_axis',(2.78074422198555E-16,1.,1.1053880869225E-14)) ;
#10407=DIRECTION('ref_axis',(0.841916892643634,5.73063831119028E-15,-0.539607214445181)) ;
#10408=DIRECTION('',(0.,-1.,-8.88178419700125E-15)) ;
#10409=DIRECTION('center_axis',(-1.12606857017318E-16,1.,1.07950474400035E-14)) ;
#10410=DIRECTION('ref_axis',(0.841916892643638,5.91989109405419E-15,-0.539607214445176)) ;
#10411=DIRECTION('center_axis',(0.867255993642043,5.43853653899861E-15,
-0.497862472468003)) ;
#10412=DIRECTION('ref_axis',(-0.497862472468003,0.,-0.867255993642043)) ;
#10413=DIRECTION('',(0.497862472467983,-8.87732316134922E-15,0.867255993642054)) ;
#10414=DIRECTION('',(0.,-1.,-8.88178419700125E-15)) ;
#10415=DIRECTION('',(0.497862472467983,-8.59990681255706E-15,0.867255993642054)) ;
#10416=DIRECTION('center_axis',(0.494543132089066,-9.82182503760574E-15,
0.869153088071104)) ;
#10417=DIRECTION('ref_axis',(0.869153088071104,0.,-0.494543132089066)) ;
#10418=DIRECTION('',(-0.8691530880711,-6.45311740160154E-15,0.494543132089074)) ;
#10419=DIRECTION('',(0.,-1.,-5.9211894646675E-15)) ;
#10420=DIRECTION('',(-0.869153088071089,-4.03319837600091E-15,0.494543132089093)) ;
#10421=DIRECTION('center_axis',(-9.65634952856587E-17,1.,9.46520975680336E-15)) ;
#10422=DIRECTION('ref_axis',(0.893709096708599,4.3328367904494E-15,-0.448646910677318)) ;
#10423=DIRECTION('',(0.,-1.,-7.40148683083438E-15)) ;
#10424=DIRECTION('center_axis',(1.19841912038013E-16,1.,1.09286484407924E-14)) ;
#10425=DIRECTION('ref_axis',(0.89370909670859,4.79600055388485E-15,-0.448646910677334)) ;
#10426=DIRECTION('center_axis',(0.914545873732089,4.76517226719697E-15,
-0.404482193476561)) ;
#10427=DIRECTION('ref_axis',(-0.404482193476561,0.,-0.914545873732089)) ;
#10428=DIRECTION('',(0.404482193476528,-9.1547395101418E-15,0.914545873732104)) ;
#10429=DIRECTION('',(0.,-1.,-8.88178419700125E-15)) ;
#10430=DIRECTION('',(0.404482193476528,-9.43215585893399E-15,0.914545873732103)) ;
#10431=DIRECTION('center_axis',(0.400982736425919,-9.74791193386703E-15,
0.916085610130615)) ;
#10432=DIRECTION('ref_axis',(0.916085610130615,0.,-0.400982736425919)) ;
#10433=DIRECTION('',(-0.916085610130582,-3.22655870080085E-15,0.400982736425995)) ;
#10434=DIRECTION('',(0.,-1.,-5.9211894646675E-15)) ;
#10435=DIRECTION('',(-0.916085610130573,-3.22655870080082E-15,0.400982736426017)) ;
#10436=DIRECTION('center_axis',(-7.13111576133292E-17,1.,1.0031952483866E-14)) ;
#10437=DIRECTION('ref_axis',(0.935709636889367,3.60570982618191E-15,-0.352771137470696)) ;
#10438=DIRECTION('',(0.,-1.,-8.88178419700125E-15)) ;
#10439=DIRECTION('center_axis',(-1.00429960718429E-16,1.,1.04064782229712E-14)) ;
#10440=DIRECTION('ref_axis',(0.935709636889337,3.76507844185907E-15,-0.352771137470776)) ;
#10441=DIRECTION('center_axis',(0.951815797848528,3.05707044117608E-15,
-0.306670322929968)) ;
#10442=DIRECTION('ref_axis',(-0.306670322929968,0.,-0.951815797848528)) ;
#10443=DIRECTION('',(0.306670322929944,-9.43215585893339E-15,0.951815797848535)) ;
#10444=DIRECTION('',(0.,-1.,-8.88178419700125E-15)) ;
#10445=DIRECTION('',(0.306670322929944,-1.01256967309138E-14,0.951815797848535)) ;
#10446=DIRECTION('center_axis',(0.303029089991586,-9.4998790733618E-15,
0.952981306542196)) ;
#10447=DIRECTION('ref_axis',(0.952981306542196,0.,-0.303029089991586)) ;
#10448=DIRECTION('',(-0.952981306542202,-3.22655870080064E-15,0.303029089991566)) ;
#10449=DIRECTION('',(0.,-1.,-1.77635683940025E-14)) ;
#10450=DIRECTION('',(-0.952981306542225,-1.61327935040036E-15,0.303029089991496)) ;
#10451=DIRECTION('center_axis',(1.2480662469827E-16,1.,9.71479571659155E-15)) ;
#10452=DIRECTION('ref_axis',(0.96745834647859,2.33739275392867E-15,-0.253030329859707)) ;
#10453=DIRECTION('',(0.,-1.,-8.88178419700125E-15)) ;
#10454=DIRECTION('center_axis',(-3.27466891807325E-16,1.,1.11937858983162E-14)) ;
#10455=DIRECTION('ref_axis',(0.967458346478616,3.14917791590319E-15,-0.253030329859608)) ;
#10456=DIRECTION('center_axis',(0.978657428903444,3.17959536473004E-15,
-0.205498508150548)) ;
#10457=DIRECTION('ref_axis',(-0.205498508150548,0.,-0.978657428903444)) ;
#10458=DIRECTION('',(0.205498508150497,-9.98698855651799E-15,0.978657428903455)) ;
#10459=DIRECTION('',(0.,-1.,-8.88178419700125E-15)) ;
#10460=DIRECTION('',(0.205498508150497,-9.98698855651799E-15,0.978657428903455)) ;
#10461=DIRECTION('center_axis',(0.201755393434541,-1.06080915271686E-14,
0.979435940335086)) ;
#10462=DIRECTION('ref_axis',(0.979435940335086,0.,-0.201755393434541)) ;
#10463=DIRECTION('',(-0.979435940335062,-1.61327935040034E-15,0.201755393434655)) ;
#10464=DIRECTION('',(0.,-1.,-1.1842378929335E-14)) ;
#10465=DIRECTION('',(-0.979435940335067,-8.06639675200175E-16,0.20175539343463)) ;
#10466=DIRECTION('center_axis',(1.82586758620613E-16,1.,9.77984243998921E-15)) ;
#10467=DIRECTION('ref_axis',(0.9886073799701,1.29152855830694E-15,-0.150517269004768)) ;
#10468=DIRECTION('',(0.,-1.,-8.88178419700125E-15)) ;
#10469=DIRECTION('center_axis',(-2.54053681858878E-16,1.,1.14670287668068E-14)) ;
#10470=DIRECTION('ref_axis',(0.988607379970118,1.97714519837175E-15,-0.150517269004648)) ;
#10471=DIRECTION('center_axis',(0.994776684370062,1.35439464247368E-15,
-0.102075208712529)) ;
#10472=DIRECTION('ref_axis',(-0.102075208712529,0.,-0.994776684370062)) ;
#10473=DIRECTION('',(0.10207520871253,-1.05418212541018E-14,0.994776684370062)) ;
#10474=DIRECTION('',(0.,-1.,-5.9211894646675E-15)) ;
#10475=DIRECTION('',(0.102075208712529,-1.01256967309135E-14,0.994776684370062)) ;
#10476=DIRECTION('center_axis',(0.0982712225671941,-1.39810986889151E-14,
0.995159669005506)) ;
#10477=DIRECTION('ref_axis',(0.995159669005506,0.,-0.0982712225671941)) ;
#10478=DIRECTION('',(-0.995159669005508,-8.06639675199961E-16,0.0982712225671731)) ;
#10479=DIRECTION('',(0.,-1.,-1.1842378929335E-14)) ;
#10480=DIRECTION('',(-0.995159669005514,-2.41991902559989E-15,0.098271222567122)) ;
#10481=DIRECTION('center_axis',(-1.35982084744398E-16,1.,9.88995300307463E-15)) ;
#10482=DIRECTION('ref_axis',(0.998925024127247,5.94285761224491E-16,-0.0463551094527745)) ;
#10483=DIRECTION('',(0.,-1.,-1.1842378929335E-14)) ;
#10484=DIRECTION('center_axis',(6.87947995565783E-17,1.,1.09363115505266E-14)) ;
#10485=DIRECTION('ref_axis',(0.998925024127252,4.38233072126194E-16,-0.0463551094526625)) ;
#10486=DIRECTION('center_axis',(0.999996958312326,-2.13640474537978E-17,
0.00246644807282737)) ;
#10487=DIRECTION('ref_axis',(0.00246644807282737,0.,-0.999996958312326)) ;
#10488=DIRECTION('',(-0.00246644807286617,-9.98698855651738E-15,0.999996958312326)) ;
#10489=DIRECTION('',(0.,-1.,-1.1842378929335E-14)) ;
#10490=DIRECTION('',(-0.00246644807286617,-1.05418212541017E-14,0.999996958312326)) ;
#10491=DIRECTION('center_axis',(-0.00628962837959365,-1.10239774849311E-14,
0.999980220091801)) ;
#10492=DIRECTION('ref_axis',(0.999980220091801,0.,0.00628962837959364)) ;
#10493=DIRECTION('',(-0.999980220091801,0.,-0.00628962837952103)) ;
#10494=DIRECTION('',(0.,-1.,-1.1842378929335E-14)) ;
#10495=DIRECTION('',(-0.999980220091801,0.,-0.00628962837952103)) ;
#10496=DIRECTION('center_axis',(3.10052989716172E-17,1.,1.02021323753836E-14)) ;
#10497=DIRECTION('ref_axis',(0.998298236681544,-6.25889133664531E-16,0.0583149263784192)) ;
#10498=DIRECTION('',(0.,-1.,-8.88178419700125E-15)) ;
#10499=DIRECTION('center_axis',(2.09939991149458E-16,1.,9.87182977187906E-15)) ;
#10500=DIRECTION('ref_axis',(0.998298236681544,-7.85257749340864E-16,0.0583149263784198)) ;
#10501=DIRECTION('center_axis',(0.994261056316501,-1.10487221809803E-15,
0.106981081936929)) ;
#10502=DIRECTION('ref_axis',(0.106981081936929,0.,-0.994261056316501)) ;
#10503=DIRECTION('',(-0.106981081936948,-9.84828038212133E-15,0.994261056316499)) ;
#10504=DIRECTION('',(0.,-1.,-8.88178419700125E-15)) ;
#10505=DIRECTION('',(-0.106981081936948,-1.02644049053096E-14,0.994261056316499)) ;
#10506=DIRECTION('center_axis',(-0.110781568841626,-8.68506275659569E-15,
0.993844778627421)) ;
#10507=DIRECTION('ref_axis',(0.993844778627421,0.,0.110781568841626)) ;
#10508=DIRECTION('',(-0.993844778627431,0.,-0.110781568841543)) ;
#10509=DIRECTION('',(0.,-1.,-8.88178419700125E-15)) ;
#10510=DIRECTION('',(-0.993844778627431,1.6132793504004E-15,-0.110781568841543)) ;
#10511=DIRECTION('center_axis',(-4.24008527350335E-16,1.,1.08192196707972E-14)) ;
#10512=DIRECTION('ref_axis',(0.986733884847439,-1.33807401433826E-15,0.162346051673214)) ;
#10513=DIRECTION('',(0.,-1.,-1.1842378929335E-14)) ;
#10514=DIRECTION('center_axis',(-3.80940090177415E-17,1.,1.00483850234157E-14)) ;
#10515=DIRECTION('ref_axis',(0.986733884847427,-1.59372698473701E-15,0.162346051673284)) ;
#10516=DIRECTION('center_axis',(0.977631822125172,-2.02289727404569E-15,
0.210323608680092)) ;
#10517=DIRECTION('ref_axis',(0.210323608680092,0.,-0.977631822125172)) ;
#10518=DIRECTION('',(-0.210323608680131,-9.84828038212189E-15,0.977631822125163)) ;
#10519=DIRECTION('',(0.,-1.,-8.88178419700125E-15)) ;
#10520=DIRECTION('',(-0.21032360868013,-9.98698855651793E-15,0.977631822125164)) ;
#10521=DIRECTION('center_axis',(-0.214059763252521,-1.01780060649862E-14,
0.976820565793061)) ;
#10522=DIRECTION('ref_axis',(0.97682056579306,0.,0.214059763252521)) ;
#10523=DIRECTION('',(-0.976820565793055,1.61327935040072E-15,-0.214059763252546)) ;
#10524=DIRECTION('',(0.,-1.,-8.88178419700125E-15)) ;
#10525=DIRECTION('',(-0.976820565793055,2.41991902560109E-15,-0.214059763252546)) ;
#10526=DIRECTION('center_axis',(-4.16654738518614E-16,1.,1.06536625491829E-14)) ;
#10527=DIRECTION('ref_axis',(0.964358670083603,-2.41713830372618E-15,0.264598479652823)) ;
#10528=DIRECTION('',(0.,-1.,-5.9211894646675E-15)) ;
#10529=DIRECTION('center_axis',(3.60484251114169E-16,1.,1.01050337219711E-14)) ;
#10530=DIRECTION('ref_axis',(0.964358670083581,-3.02141267266539E-15,0.264598479652902)) ;
#10531=DIRECTION('center_axis',(0.950291449108004,-4.53195111194576E-15,
0.311361785953592)) ;
#10532=DIRECTION('ref_axis',(0.311361785953592,0.,-0.950291449108004)) ;
#10533=DIRECTION('',(-0.311361785953556,-9.70957220772521E-15,0.950291449108015)) ;
#10534=DIRECTION('',(0.,-1.,-1.1842378929335E-14)) ;
#10535=DIRECTION('',(-0.311361785953559,-9.70957220772529E-15,0.950291449108014)) ;
#10536=DIRECTION('center_axis',(-0.314992674102648,-1.6116694398679E-14,
0.949094102426974)) ;
#10537=DIRECTION('ref_axis',(0.949094102426974,0.,0.314992674102648)) ;
#10538=DIRECTION('',(-0.949094102426984,8.06639675200338E-16,-0.314992674102618)) ;
#10539=DIRECTION('',(0.,-1.,-1.1842378929335E-14)) ;
#10540=DIRECTION('',(-0.949094102426984,1.61327935040068E-15,-0.314992674102618)) ;
#10541=DIRECTION('center_axis',(-1.06044466970472E-16,1.,1.06621542785655E-14)) ;
#10542=DIRECTION('ref_axis',(0.931417739925256,-3.78173973070147E-15,0.363951911318692)) ;
#10543=DIRECTION('',(0.,-1.,-1.03620815631681E-14)) ;
#10544=DIRECTION('center_axis',(2.78715990627001E-16,1.,9.72764976003551E-15)) ;
#10545=DIRECTION('ref_axis',(0.93141773992525,-3.79999774087469E-15,0.363951911318705)) ;
#10546=DIRECTION('center_axis',(0.912539484113185,-3.16975044997102E-15,
0.408988618343399)) ;
#10547=DIRECTION('ref_axis',(0.408988618343399,0.,-0.912539484113185)) ;
#10548=DIRECTION('',(-0.408988618343402,-9.29344768453725E-15,0.912539484113183)) ;
#10549=DIRECTION('',(0.,-1.,-5.9211894646675E-15)) ;
#10550=DIRECTION('',(-0.408988618343399,-9.2934476845372E-15,0.912539484113185)) ;
#10551=DIRECTION('center_axis',(-0.412474459298762,-8.54656819163357E-15,
0.910969165464009)) ;
#10552=DIRECTION('ref_axis',(0.910969165464009,0.,0.412474459298762)) ;
#10553=DIRECTION('',(-0.910969165464023,3.22655870080118E-15,-0.412474459298732)) ;
#10554=DIRECTION('',(0.,-1.,-5.9211894646675E-15)) ;
#10555=DIRECTION('',(-0.910969165464023,4.83983805120177E-15,-0.412474459298732)) ;
#10556=DIRECTION('center_axis',(-4.7928013500189E-17,1.,9.98863037990808E-15)) ;
#10557=DIRECTION('ref_axis',(0.888272002096688,-4.54538271531492E-15,0.459317809682079)) ;
#10558=DIRECTION('',(0.,-1.,-1.1842378929335E-14)) ;
#10559=DIRECTION('center_axis',(2.30672676937894E-16,1.,1.00715009843182E-14)) ;
#10560=DIRECTION('ref_axis',(0.888272002096683,-4.83091985290065E-15,0.459317809682087)) ;
#10561=DIRECTION('center_axis',(0.864789545569235,-4.95945989665175E-15,
0.502134485844337)) ;
#10562=DIRECTION('ref_axis',(0.502134485844337,0.,-0.864789545569235)) ;
#10563=DIRECTION('',(-0.502134485844335,-8.32249046376412E-15,0.864789545569236)) ;
#10564=DIRECTION('',(0.,-1.,-4.44089209850063E-15)) ;
#10565=DIRECTION('',(-0.50213448584433,-8.32249046376404E-15,0.864789545569239)) ;
#10566=DIRECTION('center_axis',(-0.505437088002973,-8.877387526951E-15,
0.862863459691668)) ;
#10567=DIRECTION('ref_axis',(0.862863459691668,0.,0.505437088002973)) ;
#10568=DIRECTION('',(-0.862863459691667,4.83983805120085E-15,-0.505437088002975)) ;
#10569=DIRECTION('',(0.,-1.,-4.44089209850063E-15)) ;
#10570=DIRECTION('',(-0.862863459691667,1.61327935040028E-15,-0.505437088002975)) ;
#10571=DIRECTION('center_axis',(-3.12375763769512E-16,1.,1.04175774898207E-14)) ;
#10572=DIRECTION('ref_axis',(0.835394170330091,-5.46507838902905E-15,0.549651326004494)) ;
#10573=DIRECTION('',(0.,-1.,-5.9211894646675E-15)) ;
#10574=DIRECTION('center_axis',(3.27850817823959E-16,1.,1.00244112908562E-14)) ;
#10575=DIRECTION('ref_axis',(0.835394170330105,-5.78381562038142E-15,0.549651326004473)) ;
#10576=DIRECTION('center_axis',(0.807564791795142,-6.61148326513208E-15,
0.589778862840022)) ;
#10577=DIRECTION('ref_axis',(0.589778862840022,0.,-0.807564791795142)) ;
#10578=DIRECTION('',(-0.589778862840036,-8.32249046376468E-15,0.807564791795131)) ;
#10579=DIRECTION('',(0.,-1.,-1.03620815631681E-14)) ;
#10580=DIRECTION('',(-0.589778862840039,-8.4611986381608E-15,0.807564791795129)) ;
#10581=DIRECTION('center_axis',(-0.592862042201395,-1.10336639724356E-14,
0.805304041289246)) ;
#10582=DIRECTION('ref_axis',(0.805304041289246,0.,0.592862042201395)) ;
#10583=DIRECTION('',(-0.805304041289226,7.25975707680362E-15,-0.592862042201421)) ;
#10584=DIRECTION('',(0.,-1.,-1.1842378929335E-14)) ;
#10585=DIRECTION('',(-0.80530404128922,7.25975707680356E-15,-0.59286204220143)) ;
#10586=DIRECTION('center_axis',(8.05508786178003E-16,1.,9.79559856706725E-15)) ;
#10587=DIRECTION('ref_axis',(0.773363585216148,-6.83299574258059E-15,0.633962747376868)) ;
#10588=DIRECTION('',(0.,-1.,-1.1842378929335E-14)) ;
#10589=DIRECTION('center_axis',(-6.98671796633277E-16,1.,1.0449544858123E-14)) ;
#10590=DIRECTION('ref_axis',(0.773363585216172,-6.08429484155941E-15,0.633962747376838)) ;
#10591=DIRECTION('center_axis',(0.741492189168412,-6.18313970631509E-15,
0.670961499195174)) ;
#10592=DIRECTION('ref_axis',(0.670961499195174,0.,-0.741492189168412)) ;
#10593=DIRECTION('',(-0.670961499195179,-7.21282506859625E-15,0.741492189168408)) ;
#10594=DIRECTION('',(0.,-1.,-4.44089209850062E-15)) ;
#10595=DIRECTION('',(-0.670961499195173,-7.62894959178444E-15,0.741492189168413)) ;
#10596=DIRECTION('center_axis',(-0.673791475801331,-6.49989590464668E-15,
0.738921543289586)) ;
#10597=DIRECTION('ref_axis',(0.738921543289586,0.,0.673791475801331)) ;
#10598=DIRECTION('',(-0.738921543289622,6.45311740160379E-15,-0.673791475801293)) ;
#10599=DIRECTION('',(0.,-1.,-8.88178419700125E-15)) ;
#10600=DIRECTION('',(-0.738921543289602,7.25975707680407E-15,-0.673791475801314)) ;
#10601=DIRECTION('center_axis',(5.76177143425464E-16,1.,9.72978509576633E-15)) ;
#10602=DIRECTION('ref_axis',(0.702859866825769,-7.3260436732026E-15,0.711328340223882)) ;
#10603=DIRECTION('',(0.,-1.,-1.1842378929335E-14)) ;
#10604=DIRECTION('center_axis',(-4.52089530171145E-16,1.,1.04074137845229E-14)) ;
#10605=DIRECTION('ref_axis',(0.702859866825789,-7.08533278639819E-15,0.711328340223862)) ;
#10606=DIRECTION('center_axis',(0.667295642949931,-5.98026974983842E-15,
0.744792940957444)) ;
#10607=DIRECTION('ref_axis',(0.744792940957444,0.,-0.667295642949931)) ;
#10608=DIRECTION('',(-0.744792940957427,-6.65799237101186E-15,0.66729564294995)) ;
#10609=DIRECTION('',(0.,-1.,-1.1842378929335E-14)) ;
#10610=DIRECTION('',(-0.744792940957427,-6.65799237101186E-15,0.66729564294995)) ;
#10611=DIRECTION('center_axis',(-0.747338708992256,-6.73908241214502E-15,
0.664443266232556)) ;
#10612=DIRECTION('ref_axis',(0.664443266232556,0.,0.747338708992256)) ;
#10613=DIRECTION('',(-0.66444326623258,8.06639675199954E-15,-0.747338708992235)) ;
#10614=DIRECTION('',(0.,-1.,-1.03620815631681E-14)) ;
#10615=DIRECTION('',(-0.664443266232586,7.25975707679966E-15,-0.74733870899223)) ;
#10616=DIRECTION('center_axis',(-2.40293164046626E-18,1.,1.01147575739767E-14)) ;
#10617=DIRECTION('ref_axis',(0.624655468651339,-7.89711794837585E-15,0.780900470920575)) ;
#10618=DIRECTION('',(0.,-1.,-1.1842378929335E-14)) ;
#10619=DIRECTION('center_axis',(-2.40293164048761E-18,1.,1.01147575739767E-14)) ;
#10620=DIRECTION('ref_axis',(0.624655468651347,-7.89711794837578E-15,0.780900470920569)) ;
#10621=DIRECTION('center_axis',(0.585788066026616,-8.98424710862706E-15,
0.81046427540071)) ;
#10622=DIRECTION('ref_axis',(0.81046427540071,0.,-0.585788066026616)) ;
#10623=DIRECTION('',(-0.81046427540072,-5.40961880144683E-15,0.585788066026602)) ;
#10624=DIRECTION('',(0.,-1.,-1.03620815631681E-14)) ;
#10625=DIRECTION('',(-0.810464275400719,-6.10315967342718E-15,0.585788066026603)) ;
#10626=DIRECTION('center_axis',(-0.812697942896984,-6.2108132023361E-15,
0.582685209706759)) ;
#10627=DIRECTION('ref_axis',(0.582685209706759,0.,0.812697942896984)) ;
#10628=DIRECTION('',(-0.582685209706789,7.25975707680523E-15,-0.812697942896963)) ;
#10629=DIRECTION('',(0.,-1.,-1.1842378929335E-14)) ;
#10630=DIRECTION('',(-0.582685209706783,8.87303642720631E-15,-0.812697942896967)) ;
#10631=DIRECTION('center_axis',(-2.58097566505664E-16,1.,1.01309728578212E-14)) ;
#10632=DIRECTION('ref_axis',(0.53960721444501,-8.39016587899778E-15,0.841916892643744)) ;
#10633=DIRECTION('',(0.,-1.,-1.03620815631681E-14)) ;
#10634=DIRECTION('center_axis',(-1.15038675022374E-16,1.,1.01713935082179E-14)) ;
#10635=DIRECTION('ref_axis',(0.539607214444995,-8.50139231731336E-15,0.841916892643753)) ;
#10636=DIRECTION('center_axis',(0.497862472467958,-8.95314996644656E-15,
0.867255993642069)) ;
#10637=DIRECTION('ref_axis',(0.867255993642069,0.,-0.497862472467958)) ;
#10638=DIRECTION('',(-0.867255993642076,-4.99349427825883E-15,0.497862472467946)) ;
#10639=DIRECTION('',(0.,-1.,-1.1842378929335E-14)) ;
#10640=DIRECTION('',(-0.867255993642077,-4.99349427825884E-15,0.497862472467944)) ;
#10641=DIRECTION('center_axis',(-0.869153088071225,-5.21179790260549E-15,
0.494543132088854)) ;
#10642=DIRECTION('ref_axis',(0.494543132088854,0.,0.869153088071225)) ;
#10643=DIRECTION('',(-0.494543132088752,8.87303642720399E-15,-0.869153088071283)) ;
#10644=DIRECTION('',(0.,-1.,-1.03620815631681E-14)) ;
#10645=DIRECTION('',(-0.494543132088758,9.67967610240446E-15,-0.86915308807128)) ;
#10646=DIRECTION('center_axis',(8.69948525886045E-17,1.,1.01282337442175E-14)) ;
#10647=DIRECTION('ref_axis',(0.448646910677143,-9.09072460265772E-15,0.893709096708686)) ;
#10648=DIRECTION('',(0.,-1.,-1.03620815631681E-14)) ;
#10649=DIRECTION('center_axis',(-1.11840364983332E-16,1.,1.03692241613454E-14)) ;
#10650=DIRECTION('ref_axis',(0.4486469106771,-9.21689312456731E-15,0.893709096708708)) ;
#10651=DIRECTION('center_axis',(0.404482193476513,-9.52526104942849E-15,
0.91454587373211)) ;
#10652=DIRECTION('ref_axis',(0.91454587373211,0.,-0.404482193476513)) ;
#10653=DIRECTION('',(-0.914545873732115,-4.57736975507068E-15,0.404482193476501)) ;
#10654=DIRECTION('',(0.,-1.,-1.03620815631681E-14)) ;
#10655=DIRECTION('',(-0.914545873732115,-4.57736975507068E-15,0.404482193476501)) ;
#10656=DIRECTION('center_axis',(-0.916085610130591,-4.35036638410241E-15,
0.400982736425975)) ;
#10657=DIRECTION('ref_axis',(0.400982736425975,0.,0.916085610130591)) ;
#10658=DIRECTION('',(-0.400982736425998,1.04863157776022E-14,-0.916085610130581)) ;
#10659=DIRECTION('',(0.,-1.,-1.33226762955019E-14)) ;
#10660=DIRECTION('',(-0.400982736425988,1.04863157776019E-14,-0.916085610130585)) ;
#10661=DIRECTION('center_axis',(-1.19510675862447E-15,1.,1.03007299649568E-14)) ;
#10662=DIRECTION('ref_axis',(0.352771137470432,-9.21689312456767E-15,0.935709636889467)) ;
#10663=DIRECTION('',(0.,-1.,-9.62193288008469E-15)) ;
#10664=DIRECTION('center_axis',(2.62874961807059E-16,1.,1.00597569142651E-14)) ;
#10665=DIRECTION('ref_axis',(0.352771137470435,-9.5057461887325E-15,0.935709636889465)) ;
#10666=DIRECTION('center_axis',(0.306670322929972,-9.16808398683043E-15,
0.951815797848526)) ;
#10667=DIRECTION('ref_axis',(0.951815797848526,0.,-0.306670322929972)) ;
#10668=DIRECTION('',(-0.951815797848531,-3.32899618550598E-15,0.306670322929957)) ;
#10669=DIRECTION('',(0.,-1.,-1.03620815631681E-14)) ;
#10670=DIRECTION('',(-0.951815797848531,-3.32899618550598E-15,0.306670322929957)) ;
#10671=DIRECTION('center_axis',(-0.952981306542044,-2.78616357327354E-15,
0.303029089992064)) ;
#10672=DIRECTION('ref_axis',(0.303029089992064,0.,0.952981306542044)) ;
#10673=DIRECTION('',(-0.303029089992085,8.87303642720486E-15,-0.952981306542038)) ;
#10674=DIRECTION('',(0.,-1.,-9.62193288008469E-15)) ;
#10675=DIRECTION('',(-0.303029089992087,8.87303642720491E-15,-0.952981306542037)) ;
#10676=DIRECTION('center_axis',(4.41761309766277E-16,1.,1.03191000423786E-14)) ;
#10677=DIRECTION('ref_axis',(0.253030329859623,-1.00950784740764E-14,0.967458346478612)) ;
#10678=DIRECTION('',(0.,-1.,-1.11022302462516E-14)) ;
#10679=DIRECTION('center_axis',(-1.64998512723164E-15,1.,1.01729446383235E-14)) ;
#10680=DIRECTION('ref_axis',(0.253030329859623,-9.42440391760401E-15,0.967458346478612)) ;
#10681=DIRECTION('center_axis',(0.205498508150586,-1.03749921183994E-14,
0.978657428903436)) ;
#10682=DIRECTION('ref_axis',(0.978657428903436,0.,-0.205498508150586)) ;
#10683=DIRECTION('',(-0.978657428903435,-2.35803896473325E-15,0.205498508150591)) ;
#10684=DIRECTION('',(0.,-1.,-1.11022302462516E-14)) ;
#10685=DIRECTION('',(-0.978657428903435,-2.21933079033718E-15,0.205498508150591)) ;
#10686=DIRECTION('center_axis',(-0.979435940335074,-1.96062109375471E-15,
0.201755393434598)) ;
#10687=DIRECTION('ref_axis',(0.201755393434598,0.,0.979435940335074)) ;
#10688=DIRECTION('',(-0.201755393434827,1.04863157776031E-14,-0.979435940335027)) ;
#10689=DIRECTION('',(0.,-1.,-9.25185853854297E-15)) ;
#10690=DIRECTION('',(-0.20175539343483,9.67967610240306E-15,-0.979435940335026)) ;
#10691=DIRECTION('center_axis',(1.16349434456036E-16,1.,1.01634702626516E-14)) ;
#10692=DIRECTION('ref_axis',(0.15051726900468,-1.00651943068888E-14,0.988607379970114)) ;
#10693=DIRECTION('',(0.,-1.,-9.99200722162641E-15)) ;
#10694=DIRECTION('center_axis',(-1.54373974013215E-17,1.,1.02473462852837E-14)) ;
#10695=DIRECTION('ref_axis',(0.150517269004685,-1.01282785678434E-14,0.988607379970113)) ;
#10696=DIRECTION('center_axis',(0.102075208712476,-1.03071176810047E-14,
0.994776684370067)) ;
#10697=DIRECTION('ref_axis',(0.994776684370067,0.,-0.102075208712476)) ;
#10698=DIRECTION('',(-0.994776684370067,-1.24837356956462E-15,0.10207520871248)) ;
#10699=DIRECTION('',(0.,-1.,-9.99200722162641E-15)) ;
#10700=DIRECTION('',(-0.994776684370067,-1.10966539516855E-15,0.10207520871248)) ;
#10701=DIRECTION('center_axis',(-0.995159669005516,-1.00726298496902E-15,
0.0982712225670959)) ;
#10702=DIRECTION('ref_axis',(0.0982712225670959,0.,0.995159669005516)) ;
#10703=DIRECTION('',(-0.0982712225669734,1.20995951280066E-14,-0.995159669005528)) ;
#10704=DIRECTION('',(0.,-1.,-9.80697005085555E-15)) ;
#10705=DIRECTION('',(-0.0982712225669735,1.04863157776057E-14,-0.995159669005528)) ;
#10706=DIRECTION('center_axis',(-1.01419216451375E-15,1.,9.837244959081E-15)) ;
#10707=DIRECTION('ref_axis',(0.0463551094529302,-9.77965716930322E-15,0.99892502412724)) ;
#10708=DIRECTION('',(0.,-1.,-1.02001740387436E-14)) ;
#10709=DIRECTION('center_axis',(7.57942546382629E-16,1.,1.03782113655385E-14)) ;
#10710=DIRECTION('ref_axis',(0.0463551094529352,-1.04021895484147E-14,0.99892502412724)) ;
#10711=DIRECTION('center_axis',(-0.00246644807291988,-1.01845851894549E-14,
0.999996958312326)) ;
#10712=DIRECTION('ref_axis',(0.999996958312326,0.,0.00246644807291987)) ;
#10713=DIRECTION('',(-0.999996958312326,0.,-0.00246644807291069)) ;
#10714=DIRECTION('',(0.,-1.,-1.01886092155704E-14)) ;
#10715=DIRECTION('',(-0.999996958312326,0.,-0.00246644807291067)) ;
#10716=DIRECTION('center_axis',(-0.9999802200918,6.40022194237738E-17,-0.0062896283798014)) ;
#10717=DIRECTION('ref_axis',(-0.0062896283798014,0.,0.9999802200918)) ;
#10718=DIRECTION('',(0.00628962837972571,1.20995951280024E-14,-0.9999802200918)) ;
#10719=DIRECTION('',(0.,-1.,-1.01307850997045E-14)) ;
#10720=DIRECTION('',(0.00628962837972571,8.87303642720178E-15,-0.9999802200918)) ;
#10721=DIRECTION('center_axis',(1.24526289911119E-15,1.,1.07188166549086E-14)) ;
#10722=DIRECTION('ref_axis',(-0.0583149263784924,-1.06279583516244E-14,
0.998298236681539)) ;
#10723=DIRECTION('',(0.,-1.,-1.01770443923973E-14)) ;
#10724=DIRECTION('center_axis',(-1.3595468835695E-15,1.,9.57556002417888E-15)) ;
#10725=DIRECTION('ref_axis',(-0.0583149263784947,-9.63854656379947E-15,
0.998298236681539)) ;
#10726=DIRECTION('center_axis',(-0.106981081936937,-9.97833486220179E-15,
0.9942610563165)) ;
#10727=DIRECTION('ref_axis',(0.9942610563165,0.,0.106981081936937)) ;
#10728=DIRECTION('',(-0.9942610563165,8.3224904637647E-16,-0.106981081936942)) ;
#10729=DIRECTION('',(0.,-1.,-1.01770443923973E-14)) ;
#10730=DIRECTION('',(-0.9942610563165,1.10966539516863E-15,-0.106981081936942)) ;
#10731=DIRECTION('center_axis',(-0.993844778627483,1.14948413007461E-15,
-0.110781568841076)) ;
#10732=DIRECTION('ref_axis',(-0.110781568841076,0.,0.993844778627483)) ;
#10733=DIRECTION('',(0.110781568841025,1.20995951280029E-14,-0.993844778627488)) ;
#10734=DIRECTION('',(0.,-1.,-9.99200722162641E-15)) ;
#10735=DIRECTION('',(0.110781568841026,1.12929554528027E-14,-0.993844778627488)) ;
#10736=DIRECTION('center_axis',(-2.06325056525915E-16,1.,9.99663592581918E-15)) ;
#10737=DIRECTION('ref_axis',(-0.162346051673367,-9.89751546077705E-15,0.986733884847414)) ;
#10738=DIRECTION('',(0.,-1.,-9.99200722162641E-15)) ;
#10739=DIRECTION('center_axis',(2.54720187971674E-16,1.,1.01700699513823E-14)) ;
#10740=DIRECTION('ref_axis',(-0.162346051673361,-9.99379981549869E-15,0.986733884847414)) ;
#10741=DIRECTION('center_axis',(-0.21032360868011,-1.0737514915797E-14,
0.977631822125168)) ;
#10742=DIRECTION('ref_axis',(0.977631822125168,0.,0.21032360868011)) ;
#10743=DIRECTION('',(-0.977631822125166,2.21933079033706E-15,-0.210323608680118)) ;
#10744=DIRECTION('',(0.,-1.,-1.11022302462516E-14)) ;
#10745=DIRECTION('',(-0.977631822125166,2.21933079033706E-15,-0.210323608680119)) ;
#10746=DIRECTION('center_axis',(-0.976820565792972,2.30207841056971E-15,
-0.214059763252926)) ;
#10747=DIRECTION('ref_axis',(-0.214059763252926,0.,0.976820565792972)) ;
#10748=DIRECTION('',(0.214059763252875,1.04863157776044E-14,-0.976820565792983)) ;
#10749=DIRECTION('',(0.,-1.,-9.99200722162641E-15)) ;
#10750=DIRECTION('',(0.214059763252877,1.04863157776045E-14,-0.976820565792982)) ;
#10751=DIRECTION('center_axis',(3.14375358646724E-16,1.,1.04029311063133E-14)) ;
#10752=DIRECTION('ref_axis',(-0.264598479652911,-9.94897356471713E-15,0.964358670083578)) ;
#10753=DIRECTION('',(0.,-1.,-1.03620815631681E-14)) ;
#10754=DIRECTION('center_axis',(-2.57388810828378E-16,1.,9.91553448107732E-15)) ;
#10755=DIRECTION('ref_axis',(-0.264598479652907,-9.63023633336446E-15,0.96435867008358)) ;
#10756=DIRECTION('center_axis',(-0.311361785953514,-1.0310618920799E-14,
0.950291449108029)) ;
#10757=DIRECTION('ref_axis',(0.950291449108029,0.,0.311361785953514)) ;
#10758=DIRECTION('',(-0.950291449108031,3.19028801110968E-15,-0.311361785953507)) ;
#10759=DIRECTION('',(0.,-1.,-1.11022302462516E-14)) ;
#10760=DIRECTION('',(-0.950291449108031,3.19028801110968E-15,-0.311361785953508)) ;
#10761=DIRECTION('center_axis',(-0.949094102427042,3.05407571808092E-15,
-0.314992674102442)) ;
#10762=DIRECTION('ref_axis',(-0.314992674102442,0.,0.949094102427042)) ;
#10763=DIRECTION('',(0.314992674102518,8.87303642720378E-15,-0.949094102427017)) ;
#10764=DIRECTION('',(0.,-1.,-8.88178419700125E-15)) ;
#10765=DIRECTION('',(0.314992674102523,1.04863157776047E-14,-0.949094102427015)) ;
#10766=DIRECTION('center_axis',(2.13050222577358E-16,1.,1.04778275683277E-14)) ;
#10767=DIRECTION('ref_axis',(-0.363951911318568,-9.68169443730498E-15,0.931417739925304)) ;
#10768=DIRECTION('',(0.,-1.,-1.1842378929335E-14)) ;
#10769=DIRECTION('center_axis',(-4.07408769772116E-16,1.,9.65434384961991E-15)) ;
#10770=DIRECTION('ref_axis',(-0.363951911318561,-9.14050432932127E-15,0.931417739925307)) ;
#10771=DIRECTION('center_axis',(-0.408988618343441,-9.7764772913756E-15,
0.912539484113166)) ;
#10772=DIRECTION('ref_axis',(0.912539484113166,0.,0.408988618343441)) ;
#10773=DIRECTION('',(-0.912539484113162,4.29995340627867E-15,-0.408988618343449)) ;
#10774=DIRECTION('',(0.,-1.,-1.33226762955019E-14)) ;
#10775=DIRECTION('',(-0.912539484113162,4.16124523188258E-15,-0.408988618343451)) ;
#10776=DIRECTION('center_axis',(-0.910969165464027,4.61117069050101E-15,
-0.412474459298723)) ;
#10777=DIRECTION('ref_axis',(-0.412474459298723,0.,0.910969165464027)) ;
#10778=DIRECTION('',(0.412474459298713,8.06639675200559E-15,-0.910969165464032)) ;
#10779=DIRECTION('',(0.,-1.,-1.1842378929335E-14)) ;
#10780=DIRECTION('',(0.412474459298718,8.87303642720626E-15,-0.91096916546403)) ;
#10781=DIRECTION('center_axis',(5.92970049971339E-16,1.,1.08173517202205E-14)) ;
#10782=DIRECTION('ref_axis',(-0.459317809681956,-9.33638896534518E-15,0.888272002096751)) ;
#10783=DIRECTION('',(0.,-1.,-1.1842378929335E-14)) ;
#10784=DIRECTION('center_axis',(-6.34736289703598E-16,1.,9.60689667364641E-15)) ;
#10785=DIRECTION('ref_axis',(-0.459317809681976,-8.82508302454874E-15,0.888272002096741)) ;
#10786=DIRECTION('center_axis',(-0.502134485844411,-9.34725315396912E-15,
0.864789545569192)) ;
#10787=DIRECTION('ref_axis',(0.864789545569192,0.,0.502134485844411)) ;
#10788=DIRECTION('',(-0.864789545569198,4.85478610386242E-15,-0.502134485844401)) ;
#10789=DIRECTION('',(0.,-1.,-1.03620815631681E-14)) ;
#10790=DIRECTION('',(-0.864789545569198,5.13220245265457E-15,-0.502134485844399)) ;
#10791=DIRECTION('center_axis',(-0.862863459691754,4.75053847963801E-15,
-0.505437088002826)) ;
#10792=DIRECTION('ref_axis',(-0.505437088002826,0.,0.862863459691754)) ;
#10793=DIRECTION('',(0.505437088002901,9.67967610240523E-15,-0.86286345969171)) ;
#10794=DIRECTION('',(0.,-1.,-1.03620815631681E-14)) ;
#10795=DIRECTION('',(0.505437088002901,9.67967610240523E-15,-0.86286345969171)) ;
#10796=DIRECTION('center_axis',(-2.06384456131493E-16,1.,1.00148389344165E-14)) ;
#10797=DIRECTION('ref_axis',(-0.549651326004506,-8.47977755258572E-15,0.835394170330083)) ;
#10798=DIRECTION('',(0.,-1.,-1.1842378929335E-14)) ;
#10799=DIRECTION('center_axis',(4.94903174920278E-16,1.,1.07067666570303E-14)) ;
#10800=DIRECTION('ref_axis',(-0.5496513260045,-8.67234626202893E-15,0.835394170330087)) ;
#10801=DIRECTION('center_axis',(-0.589778862840025,-8.99774787762385E-15,
0.80756479179514)) ;
#10802=DIRECTION('ref_axis',(0.80756479179514,0.,0.589778862840025)) ;
#10803=DIRECTION('',(-0.807564791795133,6.10315967342726E-15,-0.589778862840033)) ;
#10804=DIRECTION('',(0.,-1.,-1.1842378929335E-14)) ;
#10805=DIRECTION('',(-0.807564791795133,6.10315967342726E-15,-0.589778862840033)) ;
#10806=DIRECTION('center_axis',(-0.805304041289175,6.46502283087815E-15,
-0.592862042201491)) ;
#10807=DIRECTION('ref_axis',(-0.592862042201491,0.,0.805304041289175)) ;
#10808=DIRECTION('',(0.592862042201495,7.25975707680057E-15,-0.805304041289172)) ;
#10809=DIRECTION('',(0.,-1.,-1.03620815631681E-14)) ;
#10810=DIRECTION('',(0.592862042201501,8.06639675200072E-15,-0.805304041289168)) ;
#10811=DIRECTION('center_axis',(-5.37378105936948E-17,1.,1.01243572961915E-14)) ;
#10812=DIRECTION('ref_axis',(-0.633962747376891,-7.86387702663371E-15,0.773363585216129)) ;
#10813=DIRECTION('',(0.,-1.,-1.1842378929335E-14)) ;
#10814=DIRECTION('center_axis',(-5.95031163058821E-17,1.,9.97580953733601E-15)) ;
#10815=DIRECTION('ref_axis',(-0.633962747376891,-7.75265058831819E-15,0.773363585216129)) ;
#10816=DIRECTION('center_axis',(-0.670961499195151,-8.51234557961098E-15,
0.741492189168433)) ;
#10817=DIRECTION('ref_axis',(0.741492189168433,0.,0.670961499195151)) ;
#10818=DIRECTION('',(-0.741492189168433,6.79670054540769E-15,-0.670961499195151)) ;
#10819=DIRECTION('',(0.,-1.,-8.88178419700125E-15)) ;
#10820=DIRECTION('',(-0.741492189168435,6.79670054540771E-15,-0.670961499195149)) ;
#10821=DIRECTION('center_axis',(-0.738921543289562,8.37973499779816E-15,
-0.673791475801358)) ;
#10822=DIRECTION('ref_axis',(-0.673791475801358,0.,0.738921543289562)) ;
#10823=DIRECTION('',(0.673791475801357,8.87303642720419E-15,-0.738921543289563)) ;
#10824=DIRECTION('',(0.,-1.,-1.1842378929335E-14)) ;
#10825=DIRECTION('',(0.673791475801344,8.87303642720402E-15,-0.738921543289574)) ;
#10826=DIRECTION('center_axis',(3.31674154241743E-16,1.,1.07847814889023E-14)) ;
#10827=DIRECTION('ref_axis',(0.711328340223895,7.34426085540283E-15,-0.702859866825755)) ;
#10828=DIRECTION('',(0.,-1.,-8.88178419700125E-15)) ;
#10829=DIRECTION('center_axis',(1.96148416490426E-16,1.,1.05791281541831E-14)) ;
#10830=DIRECTION('ref_axis',(0.711328340223907,7.2961186780419E-15,-0.702859866825744)) ;
#10831=DIRECTION('center_axis',(-0.744792940957456,-6.11851680912663E-15,
0.667295642949918)) ;
#10832=DIRECTION('ref_axis',(0.667295642949918,0.,0.744792940957456)) ;
#10833=DIRECTION('',(-0.667295642949917,7.49024141738854E-15,-0.744792940957456)) ;
#10834=DIRECTION('',(0.,-1.,-1.03620815631681E-14)) ;
#10835=DIRECTION('',(-0.667295642949916,7.62894959178462E-15,-0.744792940957457)) ;
#10836=DIRECTION('center_axis',(-0.664443266232475,7.93440611492218E-15,
-0.747338708992329)) ;
#10837=DIRECTION('ref_axis',(-0.747338708992329,0.,0.664443266232475)) ;
#10838=DIRECTION('',(0.747338708992195,6.45311740160396E-15,-0.664443266232626)) ;
#10839=DIRECTION('',(0.,-1.,-8.88178419700125E-15)) ;
#10840=DIRECTION('',(0.747338708992201,6.45311740160402E-15,-0.664443266232618)) ;
#10841=DIRECTION('center_axis',(-2.4269460922747E-16,1.,9.29325279088581E-15)) ;
#10842=DIRECTION('ref_axis',(0.780900470920493,5.99460151202269E-15,-0.624655468651442)) ;
#10843=DIRECTION('',(0.,-1.,-1.03620815631681E-14)) ;
#10844=DIRECTION('center_axis',(2.14289630963276E-17,1.,1.03888328400212E-14)) ;
#10845=DIRECTION('ref_axis',(0.780900470920472,6.47270735905191E-15,-0.624655468651468)) ;
#10846=DIRECTION('center_axis',(-0.810464275400682,-6.27451715502398E-15,
0.585788066026653)) ;
#10847=DIRECTION('ref_axis',(0.585788066026653,0.,0.810464275400682)) ;
#10848=DIRECTION('',(-0.585788066026645,8.3224904637648E-15,-0.810464275400688)) ;
#10849=DIRECTION('',(0.,-1.,-5.9211894646675E-15)) ;
#10850=DIRECTION('',(-0.585788066026648,8.46119863816093E-15,-0.810464275400686)) ;
#10851=DIRECTION('center_axis',(-0.582685209706604,6.72659363941242E-15,
-0.812697942897096)) ;
#10852=DIRECTION('ref_axis',(-0.812697942897096,0.,0.582685209706604)) ;
#10853=DIRECTION('',(0.812697942897149,4.83983805120176E-15,-0.582685209706529)) ;
#10854=DIRECTION('',(0.,-1.,-5.9211894646675E-15)) ;
#10855=DIRECTION('',(0.812697942897149,4.83983805120176E-15,-0.582685209706529)) ;
#10856=DIRECTION('center_axis',(-1.70957791178252E-16,1.,9.90719736310644E-15)) ;
#10857=DIRECTION('ref_axis',(0.841916892643665,5.48992742438604E-15,-0.539607214445132)) ;
#10858=DIRECTION('',(0.,-1.,-8.88178419700125E-15)) ;
#10859=DIRECTION('center_axis',(1.88267979523057E-16,1.,1.08245441680019E-14)) ;
#10860=DIRECTION('ref_axis',(0.841916892643639,5.68249613382989E-15,-0.539607214445174)) ;
#10861=DIRECTION('center_axis',(-0.867255993642078,-4.40191700704748E-15,
0.497862472467942)) ;
#10862=DIRECTION('ref_axis',(0.497862472467942,0.,0.867255993642078)) ;
#10863=DIRECTION('',(-0.497862472467943,8.59990681255647E-15,-0.867255993642077)) ;
#10864=DIRECTION('',(0.,-1.,-7.40148683083438E-15)) ;
#10865=DIRECTION('',(-0.497862472467944,9.01603133574471E-15,-0.867255993642077)) ;
#10866=DIRECTION('center_axis',(-0.494543132088875,7.68473217341133E-15,
-0.869153088071213)) ;
#10867=DIRECTION('ref_axis',(-0.869153088071213,0.,0.494543132088875)) ;
#10868=DIRECTION('',(0.869153088071255,5.64647772640236E-15,-0.494543132088801)) ;
#10869=DIRECTION('',(0.,-1.,-7.40148683083438E-15)) ;
#10870=DIRECTION('',(0.869153088071255,4.83983805120202E-15,-0.494543132088801)) ;
#10871=DIRECTION('center_axis',(-3.1221234649742E-17,1.,9.70267745702815E-15)) ;
#10872=DIRECTION('ref_axis',(0.893709096708702,4.38097896780909E-15,-0.448646910677112)) ;
#10873=DIRECTION('',(0.,-1.,-7.40148683083438E-15)) ;
#10874=DIRECTION('center_axis',(3.41210259861974E-17,1.,9.94014515725119E-15)) ;
#10875=DIRECTION('ref_axis',(0.893709096708695,4.42912114517003E-15,-0.448646910677125)) ;
#10876=DIRECTION('center_axis',(-0.914545873732137,-4.20941261989503E-15,
0.404482193476453)) ;
#10877=DIRECTION('ref_axis',(0.404482193476453,0.,0.914545873732137)) ;
#10878=DIRECTION('',(-0.404482193476438,9.57086403332927E-15,-0.914545873732144)) ;
#10879=DIRECTION('',(0.,-1.,-8.88178419700125E-15)) ;
#10880=DIRECTION('',(-0.404482193476437,9.2934476845371E-15,-0.914545873732144)) ;
#10881=DIRECTION('center_axis',(-0.400982736425726,9.53362691950711E-15,
-0.9160856101307)) ;
#10882=DIRECTION('ref_axis',(-0.9160856101307,0.,0.400982736425726)) ;
#10883=DIRECTION('',(0.916085610130674,3.22655870080186E-15,-0.400982736425785)) ;
#10884=DIRECTION('',(0.,-1.,-8.88178419700125E-15)) ;
#10885=DIRECTION('',(0.916085610130674,4.03319837600232E-15,-0.400982736425785)) ;
#10886=DIRECTION('center_axis',(-2.01056104879991E-17,1.,1.08924721297816E-14)) ;
#10887=DIRECTION('ref_axis',(0.935709636889487,3.86136279657659E-15,-0.352771137470377)) ;
#10888=DIRECTION('',(0.,-1.,-8.88178419700125E-15)) ;
#10889=DIRECTION('center_axis',(-7.13111576134709E-17,1.,1.00319524838657E-14)) ;
#10890=DIRECTION('ref_axis',(0.935709636889487,3.60570982617873E-15,-0.352771137470377)) ;
#10891=DIRECTION('center_axis',(-0.951815797848514,-3.21985774616526E-15,
0.30667032293001)) ;
#10892=DIRECTION('ref_axis',(0.30667032293001,0.,0.951815797848514)) ;
#10893=DIRECTION('',(-0.306670322930025,9.84828038212145E-15,-0.951815797848509)) ;
#10894=DIRECTION('',(0.,-1.,-8.88178419700125E-15)) ;
#10895=DIRECTION('',(-0.306670322930025,9.70957220772538E-15,-0.951815797848509)) ;
#10896=DIRECTION('center_axis',(-0.303029089991788,9.05281451950862E-15,
-0.952981306542132)) ;
#10897=DIRECTION('ref_axis',(-0.952981306542132,0.,0.303029089991788)) ;
#10898=DIRECTION('',(0.952981306542113,3.22655870080145E-15,-0.303029089991849)) ;
#10899=DIRECTION('',(0.,-1.,-8.88178419700125E-15)) ;
#10900=DIRECTION('',(0.952981306542113,2.41991902560109E-15,-0.303029089991849)) ;
#10901=DIRECTION('center_axis',(1.68432817896581E-16,1.,1.04523873599391E-14)) ;
#10902=DIRECTION('ref_axis',(0.967458346478576,2.48181928601245E-15,-0.253030329859762)) ;
#10903=DIRECTION('',(0.,-1.,-8.88178419700125E-15)) ;
#10904=DIRECTION('center_axis',(-4.04932785370262E-17,1.,9.96192856271833E-15)) ;
#10905=DIRECTION('ref_axis',(0.967458346478598,2.55984563056011E-15,-0.253030329859679)) ;
#10906=DIRECTION('center_axis',(-0.978657428903448,-2.07313293814295E-15,
0.205498508150528)) ;
#10907=DIRECTION('ref_axis',(0.205498508150528,0.,0.978657428903448)) ;
#10908=DIRECTION('',(-0.20549850815054,1.01256967309133E-14,-0.978657428903445)) ;
#10909=DIRECTION('',(0.,-1.,-5.9211894646675E-15)) ;
#10910=DIRECTION('',(-0.205498508150541,9.84828038212124E-15,-0.978657428903445)) ;
#10911=DIRECTION('center_axis',(-0.201755393434603,8.89276926769736E-15,
-0.979435940335073)) ;
#10912=DIRECTION('ref_axis',(-0.979435940335073,0.,0.201755393434603)) ;
#10913=DIRECTION('',(0.979435940335075,2.41991902560011E-15,-0.201755393434595)) ;
#10914=DIRECTION('',(0.,-1.,-8.88178419700125E-15)) ;
#10915=DIRECTION('',(0.979435940335069,2.4199190256001E-15,-0.20175539343462)) ;
#10916=DIRECTION('center_axis',(-8.02786814923323E-17,1.,9.6305190171109E-15)) ;
#10917=DIRECTION('ref_axis',(0.988607379970119,1.52892351853044E-15,-0.150517269004647)) ;
#10918=DIRECTION('',(0.,-1.,-2.96059473233375E-15)) ;
#10919=DIRECTION('center_axis',(4.25238749047059E-17,1.,1.08782409716021E-14)) ;
#10920=DIRECTION('ref_axis',(0.988607379970123,1.59532370606395E-15,-0.150517269004616)) ;
#10921=DIRECTION('center_axis',(-0.994776684370068,-8.31135026344039E-16,
0.102075208712465)) ;
#10922=DIRECTION('ref_axis',(0.102075208712465,0.,0.994776684370068)) ;
#10923=DIRECTION('',(-0.102075208712471,1.01256967309134E-14,-0.994776684370068)) ;
#10924=DIRECTION('',(0.,-1.,-1.1842378929335E-14)) ;
#10925=DIRECTION('',(-0.10207520871247,1.04031130797054E-14,-0.994776684370068)) ;
#10926=DIRECTION('center_axis',(-0.0982712225670478,1.21544506469537E-14,
-0.995159669005521)) ;
#10927=DIRECTION('ref_axis',(-0.995159669005521,0.,0.0982712225670478)) ;
#10928=DIRECTION('',(0.995159669005524,0.,-0.0982712225670169)) ;
#10929=DIRECTION('',(0.,-1.,-5.9211894646675E-15)) ;
#10930=DIRECTION('',(0.995159669005529,0.,-0.0982712225669658)) ;
#10931=DIRECTION('center_axis',(-3.35936425939149E-17,1.,1.04131322768018E-14)) ;
#10932=DIRECTION('ref_axis',(0.998925024127235,5.1625941667882E-16,-0.0463551094530441)) ;
#10933=DIRECTION('',(0.,-1.,-5.9211894646675E-15)) ;
#10934=DIRECTION('center_axis',(1.13981116732401E-16,1.,9.43907375433126E-15)) ;
#10935=DIRECTION('ref_axis',(0.998925024127238,3.23690707234739E-16,-0.0463551094529721)) ;
#10936=DIRECTION('center_axis',(-0.999996958312326,3.165819530985E-17,-0.0024664480727807)) ;
#10937=DIRECTION('ref_axis',(-0.0024664480727807,0.,0.999996958312326)) ;
#10938=DIRECTION('',(0.00246644807278117,9.98698855651831E-15,-0.999996958312326)) ;
#10939=DIRECTION('',(0.,-1.,-8.88178419700125E-15)) ;
#10940=DIRECTION('',(0.00246644807278116,9.84828038212218E-15,-0.999996958312326)) ;
#10941=DIRECTION('center_axis',(0.00628962837951835,1.23218756090995E-14,
-0.999980220091801)) ;
#10942=DIRECTION('ref_axis',(-0.999980220091801,0.,-0.00628962837951835)) ;
#10943=DIRECTION('',(0.999980220091801,0.,0.00628962837952207)) ;
#10944=DIRECTION('',(0.,-1.,-5.9211894646675E-15)) ;
#10945=DIRECTION('',(0.999980220091801,0.,0.00628962837954788)) ;
#10946=DIRECTION('center_axis',(2.0993999114902E-16,1.,9.8718297718797E-15)) ;
#10947=DIRECTION('ref_axis',(0.998298236681533,-7.85257749342236E-16,0.0583149263785996)) ;
#10948=DIRECTION('',(0.,-1.,-8.88178419700125E-15)) ;
#10949=DIRECTION('center_axis',(-2.64718292924584E-16,1.,1.06244133911044E-14)) ;
#10950=DIRECTION('ref_axis',(0.99829823668153,-3.55294079674656E-16,0.0583149263786514)) ;
#10951=DIRECTION('center_axis',(-0.994261056316499,1.10829147690483E-15,
-0.106981081936945)) ;
#10952=DIRECTION('ref_axis',(-0.106981081936945,0.,0.994261056316499)) ;
#10953=DIRECTION('',(0.106981081937005,1.04031130797057E-14,-0.994261056316493)) ;
#10954=DIRECTION('',(0.,-1.,-8.88178419700125E-15)) ;
#10955=DIRECTION('',(0.106981081937005,1.01256967309136E-14,-0.994261056316493)) ;
#10956=DIRECTION('center_axis',(0.1107815688414,9.26633671878109E-15,-0.993844778627446)) ;
#10957=DIRECTION('ref_axis',(-0.993844778627446,0.,-0.1107815688414)) ;
#10958=DIRECTION('',(0.993844778627456,-2.41991902560067E-15,0.110781568841314)) ;
#10959=DIRECTION('',(0.,-1.,-8.88178419700125E-15)) ;
#10960=DIRECTION('',(0.993844778627456,0.,0.110781568841314)) ;
#10961=DIRECTION('center_axis',(9.52458188624454E-19,1.,1.01996408650293E-14)) ;
#10962=DIRECTION('ref_axis',(0.986733884847386,-1.65681124569414E-15,0.162346051673533)) ;
#10963=DIRECTION('',(0.,-1.,-8.88178419700125E-15)) ;
#10964=DIRECTION('center_axis',(-8.57645545929274E-17,1.,1.04301634872781E-14)) ;
#10965=DIRECTION('ref_axis',(0.98673388484739,-1.60866906833312E-15,0.162346051673509)) ;
#10966=DIRECTION('center_axis',(-0.977631822125173,2.52799211926821E-15,
-0.210323608680085)) ;
#10967=DIRECTION('ref_axis',(-0.210323608680085,0.,0.977631822125173)) ;
#10968=DIRECTION('',(0.210323608680057,1.01256967309132E-14,-0.977631822125179)) ;
#10969=DIRECTION('',(0.,-1.,-1.1842378929335E-14)) ;
#10970=DIRECTION('',(0.210323608680056,1.01256967309132E-14,-0.97763182212518)) ;
#10971=DIRECTION('center_axis',(0.214059763252555,1.1740929645326E-14,-0.976820565793053)) ;
#10972=DIRECTION('ref_axis',(-0.976820565793053,0.,-0.214059763252555)) ;
#10973=DIRECTION('',(0.976820565793052,-3.22655870080087E-15,0.21405976325256)) ;
#10974=DIRECTION('',(0.,-1.,-8.88178419700125E-15)) ;
#10975=DIRECTION('',(0.976820565793047,-4.03319837600107E-15,0.214059763252584)) ;
#10976=DIRECTION('center_axis',(1.81080030082074E-16,1.,9.86170298058838E-15)) ;
#10977=DIRECTION('ref_axis',(0.964358670083573,-2.78401771244109E-15,0.26459847965293)) ;
#10978=DIRECTION('',(0.,-1.,-5.9211894646675E-15)) ;
#10979=DIRECTION('center_axis',(-6.26182825359398E-17,1.,1.01475850653259E-14)) ;
#10980=DIRECTION('ref_axis',(0.964358670083549,-2.62464909676563E-15,0.264598479653017)) ;
#10981=DIRECTION('center_axis',(-0.950291449108025,2.79072426922236E-15,
-0.311361785953526)) ;
#10982=DIRECTION('ref_axis',(-0.311361785953526,0.,0.950291449108025)) ;
#10983=DIRECTION('',(0.311361785953537,9.70957220772551E-15,-0.950291449108022)) ;
#10984=DIRECTION('',(0.,-1.,-1.1842378929335E-14)) ;
#10985=DIRECTION('',(0.311361785953534,9.70957220772542E-15,-0.950291449108023)) ;
#10986=DIRECTION('center_axis',(0.314992674102732,1.05082710782995E-14,
-0.949094102426946)) ;
#10987=DIRECTION('ref_axis',(-0.949094102426946,0.,-0.314992674102732)) ;
#10988=DIRECTION('',(0.949094102426945,-3.22655870080122E-15,0.314992674102735)) ;
#10989=DIRECTION('',(0.,-1.,-1.1842378929335E-14)) ;
#10990=DIRECTION('',(0.949094102426945,-4.83983805120183E-15,0.314992674102735)) ;
#10991=DIRECTION('center_axis',(-3.91781290604668E-16,1.,1.06088593500335E-14)) ;
#10992=DIRECTION('ref_axis',(0.931417739925253,-3.49620259311591E-15,0.363951911318697)) ;
#10993=DIRECTION('',(0.,-1.,-8.88178419700125E-15)) ;
#10994=DIRECTION('center_axis',(-1.26280518287485E-16,1.,1.01939480117985E-14)) ;
#10995=DIRECTION('ref_axis',(0.931417739925251,-3.59248694783763E-15,0.363951911318703)) ;
#10996=DIRECTION('center_axis',(-0.912539484113164,4.35097671557943E-15,
-0.408988618343445)) ;
#10997=DIRECTION('ref_axis',(-0.408988618343445,0.,0.912539484113164)) ;
#10998=DIRECTION('',(0.408988618343461,9.29344768453666E-15,-0.912539484113157)) ;
#10999=DIRECTION('',(0.,-1.,-1.1842378929335E-14)) ;
#11000=DIRECTION('',(0.40898861834346,9.43215585893269E-15,-0.912539484113158)) ;
#11001=DIRECTION('center_axis',(0.412474459298714,9.2066751427435E-15,-0.910969165464031)) ;
#11002=DIRECTION('ref_axis',(-0.910969165464031,0.,-0.412474459298714)) ;
#11003=DIRECTION('',(0.910969165464035,-3.22655870080239E-15,0.412474459298706)) ;
#11004=DIRECTION('',(0.,-1.,-8.88178419700125E-15)) ;
#11005=DIRECTION('',(0.910969165464025,-4.83983805120353E-15,0.412474459298727)) ;
#11006=DIRECTION('center_axis',(-2.11241429924909E-16,1.,1.03369922670322E-14)) ;
#11007=DIRECTION('ref_axis',(0.888272002096608,-4.56032479891027E-15,0.459317809682233)) ;
#11008=DIRECTION('',(0.,-1.,-1.03620815631681E-14)) ;
#11009=DIRECTION('center_axis',(-3.55344389385075E-16,1.,1.03735164026929E-14)) ;
#11010=DIRECTION('ref_axis',(0.888272002096621,-4.4490983605945E-15,0.459317809682208)) ;
#11011=DIRECTION('center_axis',(-0.864789545569218,5.11990655170529E-15,
-0.502134485844365)) ;
#11012=DIRECTION('ref_axis',(-0.502134485844365,0.,0.864789545569218)) ;
#11013=DIRECTION('',(0.502134485844339,8.8773231613489E-15,-0.864789545569234)) ;
#11014=DIRECTION('',(0.,-1.,-5.9211894646675E-15)) ;
#11015=DIRECTION('',(0.502134485844341,8.59990681255679E-15,-0.864789545569232)) ;
#11016=DIRECTION('center_axis',(0.505437088002809,8.79800213895728E-15,
-0.862863459691764)) ;
#11017=DIRECTION('ref_axis',(-0.862863459691764,0.,-0.505437088002809)) ;
#11018=DIRECTION('',(0.86286345969171,-7.25975707680022E-15,0.505437088002902)) ;
#11019=DIRECTION('',(0.,-1.,-4.44089209850063E-15)) ;
#11020=DIRECTION('',(0.862863459691704,-4.0331983760001E-15,0.505437088002912)) ;
#11021=DIRECTION('center_axis',(-2.86525193258626E-16,1.,1.02635167737766E-14)) ;
#11022=DIRECTION('ref_axis',(0.835394170330141,-5.40199412807391E-15,0.549651326004418)) ;
#11023=DIRECTION('',(0.,-1.,-5.9211894646675E-15)) ;
#11024=DIRECTION('center_axis',(1.54868887170924E-16,1.,1.01997331986189E-14)) ;
#11025=DIRECTION('ref_axis',(0.835394170330114,-5.73567344302071E-15,0.54965132600446)) ;
#11026=DIRECTION('center_axis',(-0.807564791795179,4.15110561799591E-15,
-0.589778862839971)) ;
#11027=DIRECTION('ref_axis',(-0.589778862839971,0.,0.807564791795179)) ;
#11028=DIRECTION('',(0.589778862839977,8.32249046376459E-15,-0.807564791795174)) ;
#11029=DIRECTION('',(0.,-1.,-7.40148683083438E-15)) ;
#11030=DIRECTION('',(0.589778862839976,8.32249046376458E-15,-0.807564791795175)) ;
#11031=DIRECTION('center_axis',(0.592862042201329,8.7200926955354E-15,-0.805304041289295)) ;
#11032=DIRECTION('ref_axis',(-0.805304041289295,0.,-0.592862042201329)) ;
#11033=DIRECTION('',(0.805304041289269,-5.64647772640202E-15,0.592862042201364)) ;
#11034=DIRECTION('',(0.,-1.,-8.88178419700125E-15)) ;
#11035=DIRECTION('',(0.805304041289275,-7.25975707680266E-15,0.592862042201356)) ;
#11036=DIRECTION('center_axis',(-2.53028520067911E-16,1.,1.0432248940987E-14)) ;
#11037=DIRECTION('ref_axis',(0.773363585216212,-6.41797415650504E-15,0.633962747376789)) ;
#11038=DIRECTION('',(0.,-1.,-7.40148683083438E-15)) ;
#11039=DIRECTION('center_axis',(5.08413268466143E-16,1.,9.80712917849221E-15)) ;
#11040=DIRECTION('ref_axis',(0.773363585216203,-6.61054286594857E-15,0.6339627473768)) ;
#11041=DIRECTION('center_axis',(-0.741492189168386,5.86396883463657E-15,
-0.670961499195203)) ;
#11042=DIRECTION('ref_axis',(-0.670961499195203,0.,0.741492189168386)) ;
#11043=DIRECTION('',(0.670961499195207,7.76765776618055E-15,-0.741492189168383)) ;
#11044=DIRECTION('',(0.,-1.,-8.88178419700125E-15)) ;
#11045=DIRECTION('',(0.670961499195206,7.49024141738837E-15,-0.741492189168384)) ;
#11046=DIRECTION('center_axis',(0.673791475801613,8.07239481379984E-15,
-0.738921543289329)) ;
#11047=DIRECTION('ref_axis',(-0.738921543289329,0.,-0.673791475801613)) ;
#11048=DIRECTION('',(0.738921543289407,-8.06639675200647E-15,0.673791475801528)) ;
#11049=DIRECTION('',(0.,-1.,-7.40148683083438E-15)) ;
#11050=DIRECTION('',(0.7389215432894,-6.45311740160512E-15,0.673791475801535)) ;
#11051=DIRECTION('center_axis',(1.6487047398713E-16,1.,1.00008365712691E-14)) ;
#11052=DIRECTION('ref_axis',(0.702859866825732,-7.22975931848158E-15,0.711328340223918)) ;
#11053=DIRECTION('',(0.,-1.,-8.88178419700125E-15)) ;
#11054=DIRECTION('center_axis',(-6.00426167406994E-16,1.,1.03976200383323E-14)) ;
#11055=DIRECTION('ref_axis',(0.702859866825719,-6.97410634808367E-15,0.711328340223931)) ;
#11056=DIRECTION('center_axis',(-0.667295642949829,9.23495925018412E-15,
-0.744792940957535)) ;
#11057=DIRECTION('ref_axis',(-0.744792940957535,0.,0.667295642949829)) ;
#11058=DIRECTION('',(0.744792940957537,6.6579923710114E-15,-0.667295642949826)) ;
#11059=DIRECTION('',(0.,-1.,-8.88178419700125E-15)) ;
#11060=DIRECTION('',(0.744792940957537,6.93540871980354E-15,-0.667295642949826)) ;
#11061=DIRECTION('center_axis',(0.747338708992277,7.68942937953467E-15,
-0.664443266232533)) ;
#11062=DIRECTION('ref_axis',(-0.664443266232533,0.,-0.747338708992277)) ;
#11063=DIRECTION('',(0.664443266232557,-8.0663967520038E-15,0.747338708992256)) ;
#11064=DIRECTION('',(0.,-1.,-1.03620815631681E-14)) ;
#11065=DIRECTION('',(0.664443266232563,-9.67967610240466E-15,0.74733870899225)) ;
#11066=DIRECTION('center_axis',(-5.86289322685982E-16,1.,1.03160854512866E-14)) ;
#11067=DIRECTION('ref_axis',(0.62465546865154,-7.68960715533712E-15,0.780900470920414)) ;
#11068=DIRECTION('',(0.,-1.,-1.03620815631681E-14)) ;
#11069=DIRECTION('center_axis',(-1.24448328915284E-15,1.,1.03536356505393E-14)) ;
#11070=DIRECTION('ref_axis',(0.62465546865156,-7.30778566302953E-15,0.780900470920398)) ;
#11071=DIRECTION('center_axis',(-0.58578806602664,9.01205074559401E-15,
-0.810464275400692)) ;
#11072=DIRECTION('ref_axis',(-0.810464275400692,0.,0.58578806602664)) ;
#11073=DIRECTION('',(0.81046427540069,5.96445149903181E-15,-0.585788066026643)) ;
#11074=DIRECTION('',(0.,-1.,-1.1842378929335E-14)) ;
#11075=DIRECTION('',(0.810464275400689,5.9644514990318E-15,-0.585788066026645)) ;
#11076=DIRECTION('center_axis',(0.812697942896958,6.80319698211002E-15,
-0.582685209706796)) ;
#11077=DIRECTION('ref_axis',(-0.582685209706796,0.,-0.812697942896958)) ;
#11078=DIRECTION('',(0.582685209706823,-7.25975707680421E-15,0.812697942896939)) ;
#11079=DIRECTION('',(0.,-1.,-1.33226762955019E-14)) ;
#11080=DIRECTION('',(0.582685209706829,-7.25975707680429E-15,0.812697942896934)) ;
#11081=DIRECTION('center_axis',(-5.73712077470761E-16,1.,1.03510063935686E-14)) ;
#11082=DIRECTION('ref_axis',(0.539607214445007,-8.40510796259135E-15,0.841916892643745)) ;
#11083=DIRECTION('',(0.,-1.,-1.1842378929335E-14)) ;
#11084=DIRECTION('center_axis',(5.43474700650759E-16,1.,1.02028490167325E-14)) ;
#11085=DIRECTION('ref_axis',(0.539607214445004,-8.88321380962026E-15,0.841916892643748)) ;
#11086=DIRECTION('center_axis',(-0.497862472467949,9.24279903998311E-15,
-0.867255993642074)) ;
#11087=DIRECTION('ref_axis',(-0.867255993642074,0.,0.497862472467949)) ;
#11088=DIRECTION('',(0.867255993642073,5.13220245265459E-15,-0.49786247246795)) ;
#11089=DIRECTION('',(0.,-1.,-1.1842378929335E-14)) ;
#11090=DIRECTION('',(0.867255993642073,5.13220245265459E-15,-0.49786247246795)) ;
#11091=DIRECTION('center_axis',(0.869153088071339,5.40930396016028E-15,
-0.494543132088654)) ;
#11092=DIRECTION('ref_axis',(-0.494543132088654,0.,-0.869153088071339)) ;
#11093=DIRECTION('',(0.494543132088806,-9.67967610240516E-15,0.869153088071252)) ;
#11094=DIRECTION('',(0.,-1.,-1.03620815631681E-14)) ;
#11095=DIRECTION('',(0.494543132088801,-9.67967610240505E-15,0.869153088071255)) ;
#11096=DIRECTION('center_axis',(2.25044944025704E-16,1.,1.01833866921453E-14)) ;
#11097=DIRECTION('ref_axis',(0.448646910677237,-9.20195104097265E-15,0.893709096708639)) ;
#11098=DIRECTION('',(0.,-1.,-1.25825276124184E-14)) ;
#11099=DIRECTION('center_axis',(8.69948525886785E-17,1.,1.01282337442173E-14)) ;
#11100=DIRECTION('ref_axis',(0.44864691067723,-9.0907246026572E-15,0.893709096708643)) ;
#11101=DIRECTION('center_axis',(-0.404482193476504,8.53954795220647E-15,
-0.914545873732114)) ;
#11102=DIRECTION('ref_axis',(-0.914545873732114,0.,0.404482193476504)) ;
#11103=DIRECTION('',(0.914545873732116,4.02253705748631E-15,-0.4044821934765)) ;
#11104=DIRECTION('',(0.,-1.,-1.11022302462516E-14)) ;
#11105=DIRECTION('',(0.914545873732117,4.02253705748631E-15,-0.404482193476498)) ;
#11106=DIRECTION('center_axis',(0.916085610130586,4.65184225264105E-15,
-0.400982736425987)) ;
#11107=DIRECTION('ref_axis',(-0.400982736425986,0.,-0.916085610130586)) ;
#11108=DIRECTION('',(0.400982736425754,-8.06639675200351E-15,0.916085610130688)) ;
#11109=DIRECTION('',(0.,-1.,-1.25825276124184E-14)) ;
#11110=DIRECTION('',(0.400982736425759,-8.87303642720397E-15,0.916085610130686)) ;
#11111=DIRECTION('center_axis',(5.25932533206529E-16,1.,1.01983188707056E-14)) ;
#11112=DIRECTION('ref_axis',(0.352771137470506,-9.72819906536265E-15,0.935709636889439)) ;
#11113=DIRECTION('',(0.,-1.,-1.11022302462516E-14)) ;
#11114=DIRECTION('center_axis',(-2.23118945004188E-16,1.,1.01400812644954E-14)) ;
#11115=DIRECTION('ref_axis',(0.35277113747051,-9.40946183401001E-15,0.935709636889437)) ;
#11116=DIRECTION('center_axis',(-0.306670322929993,8.8306883875111E-15,
-0.95181579784852)) ;
#11117=DIRECTION('ref_axis',(-0.95181579784852,0.,0.306670322929993)) ;
#11118=DIRECTION('',(0.951815797848522,2.91287166231757E-15,-0.306670322929987)) ;
#11119=DIRECTION('',(0.,-1.,-1.03620815631681E-14)) ;
#11120=DIRECTION('',(0.951815797848522,3.19028801110972E-15,-0.306670322929986)) ;
#11121=DIRECTION('center_axis',(0.952981306542014,2.98443212964133E-15,
-0.30302908999216)) ;
#11122=DIRECTION('ref_axis',(-0.30302908999216,0.,-0.952981306542014)) ;
#11123=DIRECTION('',(0.303029089992011,-9.67967610240377E-15,0.952981306542061)) ;
#11124=DIRECTION('',(0.,-1.,-9.62193288008469E-15)) ;
#11125=DIRECTION('',(0.303029089992009,-1.0486315777604E-14,0.952981306542062)) ;
#11126=DIRECTION('center_axis',(1.94628463640725E-16,1.,1.01538001391442E-14)) ;
#11127=DIRECTION('ref_axis',(0.253030329859795,-9.87262559744541E-15,0.967458346478567)) ;
#11128=DIRECTION('',(0.,-1.,-9.25185853854297E-15)) ;
#11129=DIRECTION('center_axis',(1.05705549506074E-15,1.,1.03726658651972E-14)) ;
#11130=DIRECTION('ref_axis',(0.253030329859796,-1.03025892671137E-14,0.967458346478567)) ;
#11131=DIRECTION('center_axis',(-0.205498508150555,1.04287811652079E-14,
-0.978657428903442)) ;
#11132=DIRECTION('ref_axis',(-0.978657428903442,0.,0.205498508150555)) ;
#11133=DIRECTION('',(0.978657428903442,1.94191444154532E-15,-0.205498508150555)) ;
#11134=DIRECTION('',(0.,-1.,-9.99200722162641E-15)) ;
#11135=DIRECTION('',(0.978657428903442,2.3580389647336E-15,-0.205498508150556)) ;
#11136=DIRECTION('center_axis',(0.979435940334998,2.23710833589319E-15,
-0.201755393434965)) ;
#11137=DIRECTION('ref_axis',(-0.201755393434965,0.,-0.979435940334998)) ;
#11138=DIRECTION('',(0.201755393435196,-8.87303642720528E-15,0.979435940334951)) ;
#11139=DIRECTION('',(0.,-1.,-1.03620815631681E-14)) ;
#11140=DIRECTION('',(0.201755393435197,-1.12929554528067E-14,0.979435940334951)) ;
#11141=DIRECTION('center_axis',(-4.89974951768729E-16,1.,1.0045882123369E-14)) ;
#11142=DIRECTION('ref_axis',(0.150517269004771,-9.85768351385133E-15,0.9886073799701)) ;
#11143=DIRECTION('',(0.,-1.,-1.01770443923973E-14)) ;
#11144=DIRECTION('center_axis',(-1.29687638237839E-16,1.,1.01522328904347E-14)) ;
#11145=DIRECTION('ref_axis',(0.150517269004776,-1.00170521295277E-14,0.988607379970099)) ;
#11146=DIRECTION('center_axis',(-0.102075208712513,1.01166708051081E-14,
-0.994776684370064)) ;
#11147=DIRECTION('ref_axis',(-0.994776684370063,0.,0.102075208712513)) ;
#11148=DIRECTION('',(0.994776684370064,8.32249046376464E-16,-0.102075208712511)) ;
#11149=DIRECTION('',(0.,-1.,-1.03620815631681E-14)) ;
#11150=DIRECTION('',(0.994776684370064,8.32249046376464E-16,-0.102075208712511)) ;
#11151=DIRECTION('center_axis',(0.995159669005514,1.02795200060226E-15,
-0.0982712225671202)) ;
#11152=DIRECTION('ref_axis',(-0.0982712225671202,0.,-0.995159669005514)) ;
#11153=DIRECTION('',(0.0982712225673851,-8.87303642720472E-15,0.995159669005488)) ;
#11154=DIRECTION('',(0.,-1.,-9.80697005085555E-15)) ;
#11155=DIRECTION('',(0.0982712225673846,-8.87303642720467E-15,0.995159669005488)) ;
#11156=DIRECTION('center_axis',(-7.6283654532969E-17,1.,1.01609955402209E-14)) ;
#11157=DIRECTION('ref_axis',(0.0463551094530843,-1.01465365780165E-14,0.998925024127233)) ;
#11158=DIRECTION('',(0.,-1.,-1.01886092155704E-14)) ;
#11159=DIRECTION('center_axis',(-7.6283654532977E-17,1.,1.01609955402209E-14)) ;
#11160=DIRECTION('ref_axis',(0.0463551094530828,-1.01465365780165E-14,0.998925024127233)) ;
#11161=DIRECTION('center_axis',(0.00246644807280478,1.01799886558946E-14,
-0.999996958312326)) ;
#11162=DIRECTION('ref_axis',(-0.999996958312326,0.,-0.00246644807280478)) ;
#11163=DIRECTION('',(0.999996958312326,0.,0.00246644807279149)) ;
#11164=DIRECTION('',(0.,-1.,-1.01886092155704E-14)) ;
#11165=DIRECTION('',(0.999996958312326,0.,0.00246644807279149)) ;
#11166=DIRECTION('center_axis',(0.9999802200918,-6.40285403098758E-17,0.00628962837969165)) ;
#11167=DIRECTION('ref_axis',(0.00628962837969165,0.,-0.9999802200918)) ;
#11168=DIRECTION('',(-0.00628962837970035,-1.04863157776029E-14,0.9999802200918)) ;
#11169=DIRECTION('',(0.,-1.,-1.022330368509E-14)) ;
#11170=DIRECTION('',(-0.00628962837970035,-1.04863157776029E-14,0.9999802200918)) ;
#11171=DIRECTION('center_axis',(-1.30314881765276E-16,1.,1.01745098931728E-14)) ;
#11172=DIRECTION('ref_axis',(-0.0583149263785945,-1.01647945881894E-14,
0.998298236681534)) ;
#11173=DIRECTION('',(0.,-1.,-9.43689570931383E-15)) ;
#11174=DIRECTION('center_axis',(-2.2229329398051E-16,1.,1.0057720993455E-14)) ;
#11175=DIRECTION('ref_axis',(-0.0583149263785934,-1.00535681498739E-14,
0.998298236681534)) ;
#11176=DIRECTION('center_axis',(0.10698108193693,9.92439105702673E-15,-0.994261056316501)) ;
#11177=DIRECTION('ref_axis',(-0.994261056316501,0.,-0.10698108193693)) ;
#11178=DIRECTION('',(0.994261056316502,-1.10966539516868E-15,0.106981081936923)) ;
#11179=DIRECTION('',(0.,-1.,-1.03620815631681E-14)) ;
#11180=DIRECTION('',(0.994261056316502,-1.10966539516868E-15,0.106981081936921)) ;
#11181=DIRECTION('center_axis',(0.993844778627463,-1.14674067685148E-15,
0.110781568841248)) ;
#11182=DIRECTION('ref_axis',(0.110781568841248,0.,-0.993844778627463)) ;
#11183=DIRECTION('',(-0.110781568840856,-9.67967610240325E-15,0.993844778627507)) ;
#11184=DIRECTION('',(0.,-1.,-1.03620815631681E-14)) ;
#11185=DIRECTION('',(-0.110781568840856,-9.67967610240325E-15,0.993844778627507)) ;
#11186=DIRECTION('center_axis',(1.82731126992894E-16,1.,1.03348798985764E-14)) ;
#11187=DIRECTION('ref_axis',(-0.162346051673409,-1.01681105147685E-14,0.986733884847406)) ;
#11188=DIRECTION('',(0.,-1.,-1.1842378929335E-14)) ;
#11189=DIRECTION('center_axis',(-1.27058275890956E-16,1.,1.01223994058069E-14)) ;
#11190=DIRECTION('ref_axis',(-0.162346051673407,-1.00087418990923E-14,0.986733884847407)) ;
#11191=DIRECTION('center_axis',(0.210323608680103,1.03556219669971E-14,
-0.977631822125169)) ;
#11192=DIRECTION('ref_axis',(-0.977631822125169,0.,-0.210323608680103)) ;
#11193=DIRECTION('',(0.977631822125166,-2.08062261594135E-15,0.210323608680121)) ;
#11194=DIRECTION('',(0.,-1.,-1.14723045877933E-14)) ;
#11195=DIRECTION('',(0.977631822125165,-1.80320626714917E-15,0.210323608680122)) ;
#11196=DIRECTION('center_axis',(0.97682056579313,-2.26744049898666E-15,
0.214059763252206)) ;
#11197=DIRECTION('ref_axis',(0.214059763252206,0.,-0.976820565793129)) ;
#11198=DIRECTION('',(-0.214059763252224,-1.04863157776028E-14,0.976820565793125)) ;
#11199=DIRECTION('',(0.,-1.,-1.03620815631681E-14)) ;
#11200=DIRECTION('',(-0.214059763252222,-1.04863157776027E-14,0.976820565793126)) ;
#11201=DIRECTION('center_axis',(6.00257443383549E-16,1.,1.06466294189312E-14)) ;
#11202=DIRECTION('ref_axis',(-0.264598479653095,-1.01083421803929E-14,0.964358670083528)) ;
#11203=DIRECTION('',(0.,-1.,-9.62193288008469E-15)) ;
#11204=DIRECTION('center_axis',(-6.32092923448246E-16,1.,9.8282183636024E-15)) ;
#11205=DIRECTION('ref_axis',(-0.264598479653085,-9.64517841695802E-15,0.964358670083531)) ;
#11206=DIRECTION('center_axis',(0.311361785953555,1.015548158715E-14,-0.950291449108016)) ;
#11207=DIRECTION('ref_axis',(-0.950291449108016,0.,-0.311361785953555)) ;
#11208=DIRECTION('',(0.950291449108017,-2.91287166231775E-15,0.311361785953551)) ;
#11209=DIRECTION('',(0.,-1.,-9.62193288008469E-15)) ;
#11210=DIRECTION('',(0.950291449108017,-3.05157983671383E-15,0.311361785953551)) ;
#11211=DIRECTION('center_axis',(0.949094102427118,-3.3188211289215E-15,
0.314992674102214)) ;
#11212=DIRECTION('ref_axis',(0.314992674102214,0.,-0.949094102427118)) ;
#11213=DIRECTION('',(-0.314992674102324,-1.04863157776006E-14,0.949094102427081)) ;
#11214=DIRECTION('',(0.,-1.,-1.03620815631681E-14)) ;
#11215=DIRECTION('',(-0.314992674102326,-9.67967610240063E-15,0.94909410242708)) ;
#11216=DIRECTION('center_axis',(2.13050222576724E-16,1.,1.04778275683273E-14)) ;
#11217=DIRECTION('ref_axis',(-0.363951911318812,-9.6816944373038E-15,0.931417739925209)) ;
#11218=DIRECTION('',(0.,-1.,-1.1842378929335E-14)) ;
#11219=DIRECTION('center_axis',(-4.57923600694674E-17,1.,1.0205581445571E-14)) ;
#11220=DIRECTION('ref_axis',(-0.363951911318796,-9.52232582162755E-15,0.931417739925215)) ;
#11221=DIRECTION('center_axis',(0.4089886183435,9.42299093837688E-15,-0.91253948411314)) ;
#11222=DIRECTION('ref_axis',(-0.91253948411314,0.,-0.4089886183435)) ;
#11223=DIRECTION('',(0.912539484113151,-3.88382888309014E-15,0.408988618343474)) ;
#11224=DIRECTION('',(0.,-1.,-1.03620815631681E-14)) ;
#11225=DIRECTION('',(0.91253948411315,-4.16124523188229E-15,0.408988618343476)) ;
#11226=DIRECTION('center_axis',(0.910969165464123,-4.00871546860473E-15,
0.412474459298511)) ;
#11227=DIRECTION('ref_axis',(0.412474459298511,0.,-0.910969165464123)) ;
#11228=DIRECTION('',(-0.4124744592984,-1.04863157776079E-14,0.910969165464173)) ;
#11229=DIRECTION('',(0.,-1.,-1.1842378929335E-14)) ;
#11230=DIRECTION('',(-0.412474459298405,-8.87303642720676E-15,0.910969165464171)) ;
#11231=DIRECTION('center_axis',(-2.133261312597E-16,1.,1.00584160089897E-14)) ;
#11232=DIRECTION('ref_axis',(-0.459317809682225,-9.03259381758412E-15,0.888272002096612)) ;
#11233=DIRECTION('',(0.,-1.,-1.1842378929335E-14)) ;
#11234=DIRECTION('center_axis',(9.85116202033927E-17,1.,1.00776264659541E-14)) ;
#11235=DIRECTION('ref_axis',(-0.459317809682244,-8.90642529567464E-15,0.888272002096602)) ;
#11236=DIRECTION('center_axis',(0.502134485844415,9.27426518722038E-15,
-0.864789545569189)) ;
#11237=DIRECTION('ref_axis',(-0.864789545569189,0.,-0.502134485844415)) ;
#11238=DIRECTION('',(0.86478954556918,-5.40961880144727E-15,0.502134485844432)) ;
#11239=DIRECTION('',(0.,-1.,-1.03620815631681E-14)) ;
#11240=DIRECTION('',(0.864789545569179,-4.99349427825901E-15,0.502134485844433)) ;
#11241=DIRECTION('center_axis',(0.862863459691766,-5.88507142137273E-15,
0.505437088002807)) ;
#11242=DIRECTION('ref_axis',(0.505437088002807,0.,-0.862863459691766)) ;
#11243=DIRECTION('',(-0.505437088002738,-7.25975707680418E-15,0.862863459691806)) ;
#11244=DIRECTION('',(0.,-1.,-1.03620815631681E-14)) ;
#11245=DIRECTION('',(-0.505437088002738,-1.0486315777606E-14,0.862863459691806)) ;
#11246=DIRECTION('center_axis',(6.91486274403049E-16,1.,1.10268799478273E-14)) ;
#11247=DIRECTION('ref_axis',(-0.549651326004292,-8.83171487770677E-15,0.835394170330224)) ;
#11248=DIRECTION('',(0.,-1.,-1.1842378929335E-14)) ;
#11249=DIRECTION('center_axis',(-2.27645647850203E-16,1.,9.86770757427363E-15)) ;
#11250=DIRECTION('ref_axis',(-0.549651326004315,-8.36855111427142E-15,0.835394170330209)) ;
#11251=DIRECTION('center_axis',(0.589778862839997,7.48932209630947E-15,
-0.80756479179516)) ;
#11252=DIRECTION('ref_axis',(-0.80756479179516,0.,-0.589778862839997)) ;
#11253=DIRECTION('',(0.807564791795158,-6.24186784782375E-15,0.589778862839999)) ;
#11254=DIRECTION('',(0.,-1.,-1.1842378929335E-14)) ;
#11255=DIRECTION('',(0.807564791795158,-6.10315967342767E-15,0.589778862839999)) ;
#11256=DIRECTION('center_axis',(0.8053040412894,-5.68145037082667E-15,0.592862042201185)) ;
#11257=DIRECTION('ref_axis',(0.592862042201185,0.,-0.8053040412894)) ;
#11258=DIRECTION('',(-0.592862042201501,-8.06639675200317E-15,0.805304041289168)) ;
#11259=DIRECTION('',(0.,-1.,-1.1842378929335E-14)) ;
#11260=DIRECTION('',(-0.592862042201501,-8.87303642720349E-15,0.805304041289168)) ;
#11261=DIRECTION('center_axis',(9.67768243175678E-17,1.,1.01661699844692E-14)) ;
#11262=DIRECTION('ref_axis',(-0.633962747376858,-7.80079276567923E-15,0.773363585216156)) ;
#11263=DIRECTION('',(0.,-1.,-8.88178419700125E-15)) ;
#11264=DIRECTION('center_axis',(-5.9503116306081E-17,1.,9.97580953733579E-15)) ;
#11265=DIRECTION('ref_axis',(-0.633962747376867,-7.75265058831834E-15,0.773363585216148)) ;
#11266=DIRECTION('center_axis',(0.670961499195176,6.24391619839882E-15,
-0.741492189168411)) ;
#11267=DIRECTION('ref_axis',(-0.741492189168411,0.,-0.670961499195176)) ;
#11268=DIRECTION('',(0.74149218916841,-7.07411689419958E-15,0.670961499195176)) ;
#11269=DIRECTION('',(0.,-1.,-1.1842378929335E-14)) ;
#11270=DIRECTION('',(0.741492189168413,-6.79670054540746E-15,0.670961499195174)) ;
#11271=DIRECTION('center_axis',(0.738921543289395,-5.46368409941558E-15,
0.673791475801542)) ;
#11272=DIRECTION('ref_axis',(0.673791475801541,0.,-0.738921543289395)) ;
#11273=DIRECTION('',(-0.67379147580165,-7.25975707680296E-15,0.738921543289296)) ;
#11274=DIRECTION('',(0.,-1.,-1.1842378929335E-14)) ;
#11275=DIRECTION('',(-0.67379147580165,-8.06639675200329E-15,0.738921543289296)) ;
#11276=DIRECTION('center_axis',(7.04164249301842E-17,1.,1.02251381822285E-14)) ;
#11277=DIRECTION('ref_axis',(0.711328340223902,7.13675006236594E-15,-0.702859866825748)) ;
#11278=DIRECTION('',(0.,-1.,-8.88178419700125E-15)) ;
#11279=DIRECTION('center_axis',(-1.81047558190989E-16,1.,9.51715823831775E-15)) ;
#11280=DIRECTION('ref_axis',(0.71132834022391,6.8180128310131E-15,-0.70285986682574)) ;
#11281=DIRECTION('center_axis',(0.744792940957504,5.45910190214161E-15,
-0.667295642949863)) ;
#11282=DIRECTION('ref_axis',(-0.667295642949863,0.,-0.744792940957504)) ;
#11283=DIRECTION('',(0.667295642949854,-7.62894959178434E-15,0.744792940957512)) ;
#11284=DIRECTION('',(0.667295642949854,-7.62894959178434E-15,0.744792940957512)) ;
#11285=DIRECTION('center_axis',(1.01038501025472E-18,1.,1.01832385299507E-14)) ;
#11286=DIRECTION('ref_axis',(0.,-1.01832385299507E-14,1.)) ;
#11287=DIRECTION('',(0.685780405335872,-7.40870801634297E-15,0.727808515790635)) ;
#11288=DIRECTION('center_axis',(2.99231463188634E-15,1.,9.17249458945792E-15)) ;
#11289=DIRECTION('ref_axis',(-0.727808515790229,-4.21884749357582E-15,0.685780405336303)) ;
#11290=DIRECTION('center_axis',(-9.73559573494954E-19,1.,1.01191400279987E-14)) ;
#11291=DIRECTION('ref_axis',(-0.579268556534064,8.25126782750514E-15,-0.815136761170138)) ;
#11292=DIRECTION('center_axis',(-3.90366527253116E-16,1.,1.16402614894552E-14)) ;
#11293=DIRECTION('ref_axis',(0.45164185742236,1.06581410364017E-14,-0.89219932337123)) ;
#11294=DIRECTION('',(0.569953339326871,8.37382706828044E-15,-0.821677060036453)) ;
#11295=DIRECTION('center_axis',(-1.93203794446472E-16,1.,7.89444606623193E-15)) ;
#11296=DIRECTION('ref_axis',(0.821677060036449,-4.44089209850189E-15,0.569953339326876)) ;
#11297=DIRECTION('center_axis',(1.1550026710782E-15,-1.,-7.82090740015345E-15)) ;
#11298=DIRECTION('ref_axis',(0.0537080995988211,7.86672314592065E-15,-0.998556678430165)) ;
#11299=DIRECTION('center_axis',(-1.25123697270413E-16,1.,1.09805252983441E-14)) ;
#11300=DIRECTION('ref_axis',(0.201569759100209,-1.0658141036402E-14,0.979474161076383)) ;
#11301=DIRECTION('center_axis',(-4.61040819041639E-17,1.,1.0045818217579E-14)) ;
#11302=DIRECTION('ref_axis',(0.85487989018869,-5.20417042793038E-15,0.51882595670511)) ;
#11303=DIRECTION('',(0.904104831215912,4.36195963669746E-15,-0.427310723212099)) ;
#11304=DIRECTION('center_axis',(-3.71070252500866E-16,1.,1.14893261314214E-14)) ;
#11305=DIRECTION('ref_axis',(0.427310723212573,-1.0214051826551E-14,0.904104831215688)) ;
#11306=DIRECTION('center_axis',(-6.5542035569204E-17,1.,1.0154433419378E-14)) ;
#11307=DIRECTION('ref_axis',(-0.954244956658656,-3.10213905535359E-15,0.299026023435283)) ;
#11308=DIRECTION('center_axis',(-5.51213759928002E-17,1.,9.72049936282107E-15)) ;
#11309=DIRECTION('ref_axis',(-0.708966971011695,6.88338275267498E-15,-0.705241684824786)) ;
#11310=DIRECTION('',(-0.605336054385156,8.09943047508256E-15,-0.795970012790313)) ;
#11311=DIRECTION('center_axis',(-4.37006372857839E-15,1.,1.28163190547884E-14)) ;
#11312=DIRECTION('ref_axis',(0.795970012790317,1.13242748511803E-14,-0.605336054385151)) ;
#11313=DIRECTION('center_axis',(4.49394212051378E-16,-1.,-9.96715601710005E-15)) ;
#11314=DIRECTION('ref_axis',(-0.933087120399413,3.17206578464678E-15,-0.359650421582863)) ;
#11315=DIRECTION('center_axis',(2.35873547596961E-15,1.,1.17632702241326E-14)) ;
#11316=DIRECTION('ref_axis',(0.99382376454844,-3.55271367880014E-15,0.110969928443552)) ;
#11317=DIRECTION('',(-0.12701289025145,1.01053641908739E-14,-0.991901066493011)) ;
#11318=DIRECTION('center_axis',(1.15531629141496E-15,1.,9.89396570300712E-15)) ;
#11319=DIRECTION('ref_axis',(0.991901066492928,0.,-0.127012890252103)) ;
#11320=DIRECTION('center_axis',(1.00617405775911E-16,1.,1.02022269426731E-14)) ;
#11321=DIRECTION('ref_axis',(-0.0104872602741568,-1.01997769393712E-14,
0.999945007173866)) ;
#11322=DIRECTION('center_axis',(-4.95744530348576E-16,1.,9.94939236716821E-15)) ;
#11323=DIRECTION('ref_axis',(-0.889807542408672,-4.8849813083509E-15,0.456335991866343)) ;
#11324=DIRECTION('',(-0.944071595552654,-3.36845473029134E-15,0.329740538106351)) ;
#11325=DIRECTION('center_axis',(4.63955102136965E-17,1.,2.22312900262673E-14)) ;
#11326=DIRECTION('ref_axis',(-0.329740538106308,2.10942374678848E-14,-0.944071595552669)) ;
#11327=DIRECTION('center_axis',(2.20937231112283E-15,-1.,-1.67700671001831E-14)) ;
#11328=DIRECTION('ref_axis',(-0.630387654470438,-1.44011786622908E-14,0.776280493823759)) ;
#11329=DIRECTION('center_axis',(2.8694095257642E-15,1.,9.77672005189204E-15)) ;
#11330=DIRECTION('ref_axis',(0.412647106218261,7.77156117237546E-15,-0.910890973569118)) ;
#11331=DIRECTION('',(-0.982603114400669,1.89239029791646E-15,-0.185717849357851)) ;
#11332=DIRECTION('center_axis',(2.32293377607812E-15,1.,9.72874974239161E-15)) ;
#11333=DIRECTION('ref_axis',(0.185717849357345,9.10382880192643E-15,-0.982603114400765)) ;
#11334=DIRECTION('center_axis',(1.82671911090264E-17,1.,1.01683562978219E-14)) ;
#11335=DIRECTION('ref_axis',(0.94776347336036,-3.26392862059879E-15,0.318973977878926)) ;
#11336=DIRECTION('center_axis',(-4.9958972588217E-16,1.,1.09497348570251E-14)) ;
#11337=DIRECTION('ref_axis',(0.159035666357331,-1.06581410364028E-14,0.987272838087973)) ;
#11338=DIRECTION('',(0.0218677205202773,-1.01810598027907E-14,0.999760872808717)) ;
#11339=DIRECTION('center_axis',(-2.90264567693173E-16,1.,9.90066071632332E-15)) ;
#11340=DIRECTION('ref_axis',(-0.999760872808717,-4.4408920985022E-16,0.0218677205202719)) ;
#11341=DIRECTION('center_axis',(1.25843900772593E-14,-1.,4.50134704742774E-15)) ;
#11342=DIRECTION('ref_axis',(0.543486123848407,1.06264203785598E-14,0.839418151569427)) ;
#11343=DIRECTION('center_axis',(-2.52101501674842E-16,1.,9.31589964004196E-15)) ;
#11344=DIRECTION('ref_axis',(-0.738793827546322,5.99520433297592E-15,-0.673931510154746)) ;
#11345=DIRECTION('',(-0.480269231899665,-8.93208220616572E-15,0.877121123272325)) ;
#11346=DIRECTION('center_axis',(-5.02745638862898E-16,1.,8.71829150130473E-15)) ;
#11347=DIRECTION('ref_axis',(-0.877121123272599,3.77475828372576E-15,-0.480269231899166)) ;
#11348=DIRECTION('center_axis',(-2.09226926848338E-18,1.,1.02438071869812E-14)) ;
#11349=DIRECTION('ref_axis',(0.596237300106514,8.22313051181033E-15,-0.802808247317935)) ;
#11350=DIRECTION('center_axis',(-6.55287701147568E-16,1.,1.11149082005131E-14)) ;
#11351=DIRECTION('ref_axis',(0.988096989640894,-1.11022302462509E-15,0.153832178241753)) ;
#11352=DIRECTION('',(0.957586590090667,-2.94266691326012E-15,0.288145661911694)) ;
#11353=DIRECTION('center_axis',(3.1901714689479E-15,1.,8.32778241288616E-15)) ;
#11354=DIRECTION('ref_axis',(-0.288145661911686,-7.10542735760418E-15,0.95758659009067)) ;
#11355=DIRECTION('center_axis',(2.16932355798421E-14,-1.,-1.82594434819788E-14)) ;
#11356=DIRECTION('ref_axis',(0.966280551422668,2.56620121977777E-14,-0.25749154538024)) ;
#11357=DIRECTION('center_axis',(-1.0463360744244E-14,1.,5.55222444913644E-15)) ;
#11358=DIRECTION('ref_axis',(-0.869246802320409,-1.17683640610269E-14,0.494378394204019)) ;
#11359=DIRECTION('center_axis',(-1.01038501025472E-18,-1.,-1.01832385299507E-14)) ;
#11360=DIRECTION('ref_axis',(0.,1.01832385299507E-14,-1.)) ;
#11361=DIRECTION('center_axis',(1.27732005678872E-17,1.,1.01872910948437E-14)) ;
#11362=DIRECTION('ref_axis',(-0.567531504838376,-8.38184392457865E-15,0.823351681249202)) ;
#11363=DIRECTION('center_axis',(-9.9248854779219E-16,1.,1.0123642478546E-14)) ;
#11364=DIRECTION('ref_axis',(0.053708099598814,1.0162335480767E-14,-0.998556678430165)) ;
#11365=DIRECTION('',(0.,-1.,-1.03620815631681E-14)) ;
#11366=DIRECTION('center_axis',(-1.27095136349964E-15,-1.,-2.69759843588644E-14)) ;
#11367=DIRECTION('ref_axis',(0.0537080995988265,2.68673971959465E-14,-0.998556678430164)) ;
#11368=DIRECTION('',(0.,-1.,-1.03620815631681E-14)) ;
#11369=DIRECTION('center_axis',(1.36053615763085E-16,-1.,-1.01410167552715E-14)) ;
#11370=DIRECTION('ref_axis',(0.201569759100217,-9.90543958427637E-15,0.979474161076381)) ;
#11371=DIRECTION('center_axis',(-7.84926116427115E-17,1.,1.00769224206684E-14)) ;
#11372=DIRECTION('ref_axis',(0.201569759100214,-9.76996261670192E-15,0.979474161076382)) ;
#11373=DIRECTION('',(0.,-1.,-9.99200722162641E-15)) ;
#11374=DIRECTION('center_axis',(0.727808515790636,7.02309814391564E-15,
-0.685780405335871)) ;
#11375=DIRECTION('ref_axis',(-0.685780405335871,0.,-0.727808515790636)) ;
#11376=DIRECTION('',(0.,-1.,-1.1842378929335E-14)) ;
#11377=DIRECTION('',(0.685780405335872,-7.39924606485339E-15,0.727808515790635)) ;
#11378=DIRECTION('center_axis',(1.88696881337211E-17,-1.,-1.02210045222401E-14)) ;
#11379=DIRECTION('ref_axis',(-0.727808515790264,-7.02309814391841E-15,0.685780405336265)) ;
#11380=DIRECTION('center_axis',(2.99231463188634E-15,1.,9.17249458945792E-15)) ;
#11381=DIRECTION('ref_axis',(-0.727808515790229,-4.21884749357582E-15,0.685780405336303)) ;
#11382=DIRECTION('',(0.,-1.,-8.88178419700125E-15)) ;
#11383=DIRECTION('center_axis',(-8.16917681390859E-16,-1.,-9.66049649164156E-15)) ;
#11384=DIRECTION('ref_axis',(-0.579268556534065,8.34784054759856E-15,-0.815136761170137)) ;
#11385=DIRECTION('center_axis',(1.12759823687013E-17,1.,1.01917284713483E-14)) ;
#11386=DIRECTION('ref_axis',(-0.579268556534064,8.31457678781848E-15,-0.815136761170138)) ;
#11387=DIRECTION('',(0.,-1.,-8.88178419700125E-15)) ;
#11388=DIRECTION('center_axis',(5.64135403633836E-16,-1.,-9.18738132441649E-15)) ;
#11389=DIRECTION('ref_axis',(0.45164185742237,8.45176256273169E-15,-0.892199323371225)) ;
#11390=DIRECTION('center_axis',(-5.55151177432328E-15,1.,1.23389758122368E-14)) ;
#11391=DIRECTION('ref_axis',(0.451641857422362,1.35447209004271E-14,-0.892199323371229)) ;
#11392=DIRECTION('',(0.,-1.,-8.88178419700125E-15)) ;
#11393=DIRECTION('center_axis',(-0.821677060036453,5.25321865069352E-15,
-0.569953339326871)) ;
#11394=DIRECTION('ref_axis',(-0.569953339326871,0.,0.821677060036453)) ;
#11395=DIRECTION('',(0.569953339326872,8.37382706828045E-15,-0.821677060036452)) ;
#11396=DIRECTION('',(0.,-1.,-9.99200722162641E-15)) ;
#11397=DIRECTION('center_axis',(1.15120034560029E-17,-1.,-1.01296141149143E-14)) ;
#11398=DIRECTION('ref_axis',(0.821677060036409,-5.76394824173468E-15,0.569953339326935)) ;
#11399=DIRECTION('center_axis',(2.83896812655439E-15,1.,1.61596563378519E-14)) ;
#11400=DIRECTION('ref_axis',(0.821677060036451,-1.15463194561049E-14,0.569953339326874)) ;
#11401=DIRECTION('center_axis',(4.35568030595358E-19,-1.,-1.01768969648663E-14)) ;
#11402=DIRECTION('ref_axis',(0.997217727878536,7.59060640552051E-16,-0.0745439682655105)) ;
#11403=DIRECTION('center_axis',(8.35722644427098E-17,1.,1.0193865474578E-14)) ;
#11404=DIRECTION('ref_axis',(0.85487989018869,-5.34294830600853E-15,0.51882595670511)) ;
#11405=DIRECTION('',(-4.35568030595358E-19,1.,1.01768969648663E-14)) ;
#11406=DIRECTION('center_axis',(3.00697478893843E-18,1.,1.01692228197527E-14)) ;
#11407=DIRECTION('ref_axis',(-0.933087120399434,3.66017104374068E-15,-0.35965042158281)) ;
#11408=DIRECTION('',(0.,-1.,-1.01770443923973E-14)) ;
#11409=DIRECTION('center_axis',(-5.14081247751989E-15,-1.,-1.14600397072667E-14)) ;
#11410=DIRECTION('ref_axis',(-0.933087120399412,8.91350485485745E-15,-0.359650421582866)) ;
#11411=DIRECTION('',(0.,-1.,-1.01770443923973E-14)) ;
#11412=DIRECTION('center_axis',(-2.48643695099992E-19,-1.,-1.01827982029087E-14)) ;
#11413=DIRECTION('ref_axis',(0.993823764548442,-1.13023149594521E-15,0.110969928443534)) ;
#11414=DIRECTION('center_axis',(8.86561589770877E-17,1.,1.04217772078769E-14)) ;
#11415=DIRECTION('ref_axis',(0.99382376454844,-1.33226762955005E-15,0.110969928443552)) ;
#11416=DIRECTION('',(0.,-1.,-1.01822847028976E-14)) ;
#11417=DIRECTION('center_axis',(-0.427310723212094,9.20507379483528E-15,
-0.904104831215914)) ;
#11418=DIRECTION('ref_axis',(-0.904104831215914,0.,0.427310723212094)) ;
#11419=DIRECTION('',(0.,-1.,-1.03620815631681E-14)) ;
#11420=DIRECTION('',(0.904104831215912,4.34303573371829E-15,-0.427310723212099)) ;
#11421=DIRECTION('center_axis',(1.05573181252421E-16,-1.,-1.01629152374729E-14)) ;
#11422=DIRECTION('ref_axis',(0.42731072321255,-9.14322821300122E-15,0.904104831215699)) ;
#11423=DIRECTION('center_axis',(1.37735827364208E-16,1.,9.59365051910165E-15)) ;
#11424=DIRECTION('ref_axis',(0.427310723212573,-8.65973959207583E-15,0.904104831215688)) ;
#11425=DIRECTION('',(0.,-1.,-1.03620815631681E-14)) ;
#11426=DIRECTION('center_axis',(2.24889090216542E-18,-1.,-1.02338540319814E-14)) ;
#11427=DIRECTION('ref_axis',(-0.954244956658656,-3.06233466840199E-15,0.299026023435285)) ;
#11428=DIRECTION('center_axis',(8.21270872692169E-19,1.,1.01916550133699E-14)) ;
#11429=DIRECTION('ref_axis',(-0.954244956658657,-3.04586442396396E-15,0.299026023435282)) ;
#11430=DIRECTION('',(0.,-1.,-1.1842378929335E-14)) ;
#11431=DIRECTION('center_axis',(-2.23460467479023E-16,-1.,-1.00163897919004E-14)) ;
#11432=DIRECTION('ref_axis',(-0.708966971011677,7.22240170347135E-15,-0.705241684824804)) ;
#11433=DIRECTION('center_axis',(2.75045346022906E-17,1.,1.06984003662012E-14)) ;
#11434=DIRECTION('ref_axis',(-0.708966971011695,7.54951656744997E-15,-0.705241684824786)) ;
#11435=DIRECTION('',(0.,-1.,-1.1842378929335E-14)) ;
#11436=DIRECTION('center_axis',(-0.79597001279031,-6.19926508094888E-15,
0.60533605438516)) ;
#11437=DIRECTION('ref_axis',(0.60533605438516,0.,0.79597001279031)) ;
#11438=DIRECTION('',(-0.605336054385156,8.09943047508256E-15,-0.795970012790313)) ;
#11439=DIRECTION('',(0.,-1.,-9.99200722162641E-15)) ;
#11440=DIRECTION('center_axis',(-8.09828272505317E-18,-1.,-1.02516792551804E-14)) ;
#11441=DIRECTION('ref_axis',(0.795970012790343,6.19926508094789E-15,-0.605336054385117)) ;
#11442=DIRECTION('center_axis',(9.43700811201809E-15,1.,1.03942385143954E-14)) ;
#11443=DIRECTION('ref_axis',(0.795970012790318,-1.11022302462551E-15,-0.60533605438515)) ;
#11444=DIRECTION('center_axis',(4.4990462626596E-16,1.,1.05423745132031E-14)) ;
#11445=DIRECTION('ref_axis',(-0.630387654470441,-7.90022537109696E-15,0.776280493823757)) ;
#11446=DIRECTION('',(0.,-1.,-1.03620815631681E-14)) ;
#11447=DIRECTION('center_axis',(-4.63754202816028E-15,-1.,-2.86699818779913E-15)) ;
#11448=DIRECTION('ref_axis',(-0.630387654470438,6.97854472622012E-16,0.77628049382376)) ;
#11449=DIRECTION('',(0.,-1.,-9.99200722162641E-15)) ;
#11450=DIRECTION('center_axis',(9.31785348230183E-17,-1.,-1.00708065010557E-14)) ;
#11451=DIRECTION('ref_axis',(0.412647106218168,9.21185659112935E-15,-0.91089097356916)) ;
#11452=DIRECTION('center_axis',(-3.52226263200537E-15,1.,9.96767797577172E-15)) ;
#11453=DIRECTION('ref_axis',(0.412647106218264,1.04360964314755E-14,-0.910890973569116)) ;
#11454=DIRECTION('',(0.,-1.,-9.99200722162641E-15)) ;
#11455=DIRECTION('center_axis',(-0.991901066493012,-1.3007429008436E-15,
0.127012890251444)) ;
#11456=DIRECTION('ref_axis',(0.127012890251444,0.,0.991901066493012)) ;
#11457=DIRECTION('',(0.,-1.,-7.40148683083438E-15)) ;
#11458=DIRECTION('',(-0.12701289025145,1.01148261423635E-14,-0.991901066493011)) ;
#11459=DIRECTION('center_axis',(3.94655273193483E-17,-1.,-9.93282650058954E-15)) ;
#11460=DIRECTION('ref_axis',(0.991901066492934,1.30074290085124E-15,-0.127012890252055)) ;
#11461=DIRECTION('center_axis',(-9.73674917507053E-16,1.,8.39436511489026E-15)) ;
#11462=DIRECTION('ref_axis',(0.991901066492929,1.99840144432547E-15,-0.127012890252095)) ;
#11463=DIRECTION('',(0.,-1.,-1.03620815631681E-14)) ;
#11464=DIRECTION('center_axis',(9.70577347955382E-16,-1.,-9.71879985172455E-15)) ;
#11465=DIRECTION('ref_axis',(-0.0104872602741544,-9.72844408471828E-15,
0.999945007173866)) ;
#11466=DIRECTION('center_axis',(-8.65191641729209E-18,1.,1.02495761242682E-14)) ;
#11467=DIRECTION('ref_axis',(-0.0104872602741568,-1.02490172418371E-14,
0.999945007173866)) ;
#11468=DIRECTION('',(0.,-1.,-1.11022302462516E-14)) ;
#11469=DIRECTION('center_axis',(-8.59442262184789E-18,-1.,-1.02577888676658E-14)) ;
#11470=DIRECTION('ref_axis',(-0.889807542408722,-4.67335087520974E-15,0.456335991866246)) ;
#11471=DIRECTION('center_axis',(1.04858035239816E-16,1.,1.01895922080626E-14)) ;
#11472=DIRECTION('ref_axis',(-0.889807542408673,-4.66293670342585E-15,0.456335991866342)) ;
#11473=DIRECTION('',(0.,-1.,-1.1842378929335E-14)) ;
#11474=DIRECTION('center_axis',(0.329740538106355,-9.42655948374898E-15,
0.944071595552653)) ;
#11475=DIRECTION('ref_axis',(0.944071595552653,0.,-0.329740538106355)) ;
#11476=DIRECTION('',(-0.944071595552654,-3.35899277880175E-15,0.329740538106351)) ;
#11477=DIRECTION('',(0.,-1.,-9.99200722162641E-15)) ;
#11478=DIRECTION('center_axis',(2.37459557569859E-17,-1.,-1.01213116247813E-14)) ;
#11479=DIRECTION('ref_axis',(-0.329740538106337,9.5474128104636E-15,-0.944071595552659)) ;
#11480=DIRECTION('center_axis',(-3.88792192335817E-16,1.,1.14881096764339E-14)) ;
#11481=DIRECTION('ref_axis',(-0.32974053810631,1.0658141036405E-14,-0.944071595552669)) ;
#11482=DIRECTION('center_axis',(2.42728163606961E-16,1.,1.00838748912754E-14)) ;
#11483=DIRECTION('ref_axis',(0.543486123848403,-8.59650701067922E-15,0.83941815156943)) ;
#11484=DIRECTION('',(0.,-1.,-9.99200722162641E-15)) ;
#11485=DIRECTION('center_axis',(1.29625497688541E-14,-1.,4.18092764719124E-15)) ;
#11486=DIRECTION('ref_axis',(0.543486123848413,1.05629790628669E-14,0.839418151569423)) ;
#11487=DIRECTION('',(0.,-1.,-9.99200722162641E-15)) ;
#11488=DIRECTION('center_axis',(-3.28765762400409E-17,-1.,-1.01409834277618E-14)) ;
#11489=DIRECTION('ref_axis',(-0.738793827546362,6.85861728752183E-15,-0.673931510154701)) ;
#11490=DIRECTION('center_axis',(2.41297603013022E-16,1.,1.00743387886781E-14)) ;
#11491=DIRECTION('ref_axis',(-0.73879382754632,6.88338275267602E-15,-0.673931510154747)) ;
#11492=DIRECTION('',(0.,-1.,-9.99200722162641E-15)) ;
#11493=DIRECTION('center_axis',(-0.185717849357856,-1.00628686023381E-14,
0.982603114400668)) ;
#11494=DIRECTION('ref_axis',(0.982603114400668,0.,0.185717849357856)) ;
#11495=DIRECTION('',(0.,-1.,-9.62193288008469E-15)) ;
#11496=DIRECTION('',(-0.982603114400669,1.89239029791646E-15,-0.185717849357851)) ;
#11497=DIRECTION('center_axis',(8.26778425727097E-18,-1.,-1.01114550972676E-14)) ;
#11498=DIRECTION('ref_axis',(0.185717849357425,9.93708274481032E-15,-0.98260311440075)) ;
#11499=DIRECTION('center_axis',(4.37018402263533E-15,1.,6.82416255865663E-15)) ;
#11500=DIRECTION('ref_axis',(0.185717849357345,5.99520433297595E-15,-0.982603114400765)) ;
#11501=DIRECTION('',(0.,-1.,-9.62193288008469E-15)) ;
#11502=DIRECTION('center_axis',(3.62128080408835E-17,-1.,-1.0348629313777E-14)) ;
#11503=DIRECTION('ref_axis',(0.947763473360361,-3.26662228108087E-15,0.318973977878924)) ;
#11504=DIRECTION('center_axis',(-2.1280459065345E-16,1.,9.97985065191849E-15)) ;
#11505=DIRECTION('ref_axis',(0.94776347336036,-2.98255546365061E-15,0.318973977878926)) ;
#11506=DIRECTION('',(0.,-1.,-1.03620815631681E-14)) ;
#11507=DIRECTION('center_axis',(-2.80344073704828E-16,-1.,-9.93984541648658E-15)) ;
#11508=DIRECTION('ref_axis',(0.159035666357184,-9.85792410106006E-15,0.987272838087996)) ;
#11509=DIRECTION('center_axis',(7.4253034470058E-16,1.,9.45879140455388E-15)) ;
#11510=DIRECTION('ref_axis',(0.159035666357338,-9.54791801177758E-15,0.987272838087971)) ;
#11511=DIRECTION('',(0.,-1.,-7.40148683083438E-15)) ;
#11512=DIRECTION('center_axis',(0.999760872808717,2.18349295995649E-16,
-0.0218677205202793)) ;
#11513=DIRECTION('ref_axis',(-0.0218677205202793,0.,-0.999760872808717)) ;
#11514=DIRECTION('',(0.0218677205202773,-1.01905217542803E-14,0.999760872808717)) ;
#11515=DIRECTION('',(0.,-1.,-1.07321559047098E-14)) ;
#11516=DIRECTION('center_axis',(5.0107008882313E-19,-1.,-1.0282128875273E-14)) ;
#11517=DIRECTION('ref_axis',(-0.999760872808717,-2.25347670868714E-16,0.0218677205202789)) ;
#11518=DIRECTION('center_axis',(1.9244387534717E-15,1.,1.1331727736871E-14)) ;
#11519=DIRECTION('ref_axis',(-0.999760872808717,1.77635683940087E-15,0.0218677205202701)) ;
#11520=DIRECTION('center_axis',(-1.47015018359715E-17,1.,1.01378559388477E-14)) ;
#11521=DIRECTION('ref_axis',(0.966280551422667,2.62461796783717E-15,-0.257491545380244)) ;
#11522=DIRECTION('',(0.,-1.,-1.02695629777827E-14)) ;
#11523=DIRECTION('center_axis',(1.41800139605514E-14,-1.,-1.62531235822279E-14)) ;
#11524=DIRECTION('ref_axis',(0.966280551422669,1.78904510253976E-14,-0.257491545380237)) ;
#11525=DIRECTION('',(0.,-1.,-9.99200722162641E-15)) ;
#11526=DIRECTION('center_axis',(-1.37590905074469E-17,-1.,-1.02012162869233E-14)) ;
#11527=DIRECTION('ref_axis',(-0.869246802320393,-5.03130088143227E-15,0.494378394204046)) ;
#11528=DIRECTION('center_axis',(-5.18014709467136E-15,1.,9.15466687533215E-15)) ;
#11529=DIRECTION('ref_axis',(-0.869246802320409,-9.10382880192644E-15,0.494378394204018)) ;
#11530=DIRECTION('',(0.,-1.,-9.99200722162641E-15)) ;
#11531=DIRECTION('center_axis',(0.877121123272322,-4.85697127072896E-15,
0.480269231899671)) ;
#11532=DIRECTION('ref_axis',(0.480269231899671,0.,-0.877121123272322)) ;
#11533=DIRECTION('',(0.,-1.,-1.03620815631681E-14)) ;
#11534=DIRECTION('',(-0.480269231899665,-8.93208220616572E-15,0.877121123272325)) ;
#11535=DIRECTION('center_axis',(-3.92906616480111E-17,-1.,-1.0169273661626E-14)) ;
#11536=DIRECTION('ref_axis',(-0.877121123272574,4.91845191972174E-15,-0.48026923189921)) ;
#11537=DIRECTION('center_axis',(-6.63014437645751E-16,1.,1.07398920018271E-14)) ;
#11538=DIRECTION('ref_axis',(-0.877121123272594,4.6629367034259E-15,-0.480269231899175)) ;
#11539=DIRECTION('',(0.,-1.,-1.1842378929335E-14)) ;
#11540=DIRECTION('center_axis',(5.50013901675183E-17,-1.,-9.94415591679671E-15)) ;
#11541=DIRECTION('ref_axis',(0.596237300106512,8.01604426299543E-15,-0.802808247317936)) ;
#11542=DIRECTION('center_axis',(1.63311325766893E-16,1.,1.01319355034507E-14)) ;
#11543=DIRECTION('ref_axis',(0.596237300106513,8.03320363087032E-15,-0.802808247317936)) ;
#11544=DIRECTION('',(0.,-1.,-1.03620815631681E-14)) ;
#11545=DIRECTION('center_axis',(-1.52159333529704E-17,-1.,-1.01432954457967E-14)) ;
#11546=DIRECTION('ref_axis',(0.988096989640907,-1.5754000509151E-15,0.153832178241672)) ;
#11547=DIRECTION('center_axis',(-8.46415552567221E-16,1.,9.70638848492343E-15)) ;
#11548=DIRECTION('ref_axis',(0.988096989640894,-6.66133814775051E-16,0.153832178241752)) ;
#11549=DIRECTION('',(0.,-1.,-9.99200722162641E-15)) ;
#11550=DIRECTION('center_axis',(0.288145661911693,9.745381900288E-15,-0.957586590090668)) ;
#11551=DIRECTION('ref_axis',(-0.957586590090668,0.,-0.288145661911693)) ;
#11552=DIRECTION('',(0.957586590090667,-2.91428105879137E-15,0.288145661911694)) ;
#11553=DIRECTION('',(0.,-1.,-1.01770443923973E-14)) ;
#11554=DIRECTION('center_axis',(-4.04272951601914E-17,-1.,-1.02051907145046E-14)) ;
#11555=DIRECTION('ref_axis',(-0.288145661911697,-9.76070482780411E-15,0.957586590090666)) ;
#11556=DIRECTION('center_axis',(-3.73351796497035E-15,1.,1.37656397128939E-14)) ;
#11557=DIRECTION('ref_axis',(-0.288145661911685,-1.42108547152084E-14,0.95758659009067)) ;
#11558=DIRECTION('center_axis',(3.25068633533587E-16,-1.,-1.13443493764018E-14)) ;
#11559=DIRECTION('ref_axis',(0.016584812332587,-1.13401417803123E-14,0.99986246254167)) ;
#11560=DIRECTION('',(-3.25068633533587E-16,1.,1.13443493764018E-14)) ;
#11561=DIRECTION('center_axis',(-8.63182864965974E-18,-1.,-1.0183797638573E-14)) ;
#11562=DIRECTION('ref_axis',(0.594525808996939,-8.1952846003432E-15,0.804076527723907)) ;
#11563=DIRECTION('center_axis',(5.42235451464647E-16,1.,1.13299633222955E-14)) ;
#11564=DIRECTION('ref_axis',(0.0165848123325861,-1.13397508997188E-14,0.99986246254167)) ;
#11565=DIRECTION('center_axis',(-8.64209275723101E-18,1.,1.01866654475327E-14)) ;
#11566=DIRECTION('ref_axis',(-0.567531504838378,-8.39360559958068E-15,0.823351681249201)) ;
#11567=DIRECTION('',(-5.42235451464647E-16,-1.,-1.13299633222955E-14)) ;
#11568=DIRECTION('center_axis',(-1.30163597487239E-17,-1.,-1.01751445312373E-14)) ;
#11569=DIRECTION('ref_axis',(0.594525808996942,-8.19172107843299E-15,0.804076527723905)) ;
#11570=DIRECTION('center_axis',(1.40039764464111E-20,-1.,-1.01816657134689E-14)) ;
#11571=DIRECTION('ref_axis',(0.,1.01816657134689E-14,-1.)) ;
#11572=DIRECTION('center_axis',(-1.01038501025472E-18,-1.,-1.01832385299507E-14)) ;
#11573=DIRECTION('ref_axis',(0.,1.01832385299507E-14,-1.)) ;
#194853=CARTESIAN_POINT('Origin',(59.7994569137529,3.00000000004983,67.2203874623164)) ;
#194854=CARTESIAN_POINT('',(60.0566078658528,3.00000000004983,66.9917599116864)) ;
#194855=CARTESIAN_POINT('',(59.542305961653,3.00000000004982,67.4490150129465)) ;
#194856=CARTESIAN_POINT('',(60.0566078658528,3.00000000004983,66.9917599116864)) ;
#194857=CARTESIAN_POINT('',(59.542305961653,-2.99999999995018,67.4490150129464)) ;
#194858=CARTESIAN_POINT('',(59.542305961653,3.00000000004982,67.4490150129465)) ;
#194859=CARTESIAN_POINT('',(60.0566078658528,-2.99999999995017,66.9917599116863)) ;
#194860=CARTESIAN_POINT('',(60.0566078658528,-2.99999999995017,66.9917599116863)) ;
#194861=CARTESIAN_POINT('',(60.0566078658528,3.00000000004983,66.9917599116864)) ;
#194862=CARTESIAN_POINT('Ctrl Pts',(59.542305961653,3.00000000004982,67.4490150129465)) ;
#194863=CARTESIAN_POINT('Ctrl Pts',(59.542305961653,-4.19999999995018,67.4490150129464)) ;
#194864=CARTESIAN_POINT('Ctrl Pts',(59.5414850140413,3.00000000004983,67.447985689744)) ;
#194865=CARTESIAN_POINT('Ctrl Pts',(59.5414850140413,-4.19999999995018,
67.447985689744)) ;
#194866=CARTESIAN_POINT('Ctrl Pts',(59.5406625872324,3.00000000004983,67.44695754941)) ;
#194867=CARTESIAN_POINT('Ctrl Pts',(59.5406625872324,-4.19999999995018,
67.4469575494099)) ;
#194868=CARTESIAN_POINT('Ctrl Pts',(57.0984025861256,3.00000000004986,64.3938153283195)) ;
#194869=CARTESIAN_POINT('Ctrl Pts',(57.0984025861256,-4.19999999995015,
64.3938153283194)) ;
#194870=CARTESIAN_POINT('Ctrl Pts',(50.3765961969602,3.0000000000498,69.658693810807)) ;
#194871=CARTESIAN_POINT('Ctrl Pts',(50.3765961969602,-4.1999999999502,69.6586938108069)) ;
#194872=CARTESIAN_POINT('',(50.3765961969604,3.0000000000498,69.6586938108071)) ;
#194873=CARTESIAN_POINT('Origin',(52.7209259427923,3.00000000004977,72.9021800116133)) ;
#194874=CARTESIAN_POINT('',(50.3765961969604,-2.9999999999502,69.658693810807)) ;
#194875=CARTESIAN_POINT('',(50.3765961969604,3.0000000000498,69.6586938108071)) ;
#194876=CARTESIAN_POINT('Origin',(52.720925942792,-2.99999999995023,72.9021800116138)) ;
#194877=CARTESIAN_POINT('Origin',(51.5487610698759,3.00000000004979,71.2804369112112)) ;
#194878=CARTESIAN_POINT('',(52.7209259427917,3.00000000004977,72.9021800116154)) ;
#194879=CARTESIAN_POINT('',(50.3765961969604,3.0000000000498,69.6586938108071)) ;
#194880=CARTESIAN_POINT('',(52.7209259427917,-2.99999999995023,72.9021800116153)) ;
#194881=CARTESIAN_POINT('',(52.7209259427917,3.00000000004977,72.9021800116154)) ;
#194882=CARTESIAN_POINT('',(50.3765961969604,-2.9999999999502,69.658693810807)) ;
#194883=CARTESIAN_POINT('Origin',(52.4412856039855,3.00000000004977,73.1026755227506)) ;
#194884=CARTESIAN_POINT('',(52.1616452651796,3.00000000004977,73.3031710338859)) ;
#194885=CARTESIAN_POINT('',(52.7209259427917,3.00000000004977,72.9021800116154)) ;
#194886=CARTESIAN_POINT('',(52.1616452651796,-2.99999999995024,73.3031710338858)) ;
#194887=CARTESIAN_POINT('',(52.1616452651796,3.00000000004977,73.3031710338859)) ;
#194888=CARTESIAN_POINT('',(52.7209259427917,-2.99999999995023,72.9021800116153)) ;
#194889=CARTESIAN_POINT('Ctrl Pts',(52.1616452651794,3.00000000004977,73.3031710338858)) ;
#194890=CARTESIAN_POINT('Ctrl Pts',(52.1616452651794,-4.19999999995024,
73.3031710338858)) ;
#194891=CARTESIAN_POINT('Ctrl Pts',(52.1609364083768,3.00000000004977,73.3020615370311)) ;
#194892=CARTESIAN_POINT('Ctrl Pts',(52.1609364083768,-4.19999999995024,
73.3020615370311)) ;
#194893=CARTESIAN_POINT('Ctrl Pts',(52.1602259568374,3.00000000004977,73.3009530619476)) ;
#194894=CARTESIAN_POINT('Ctrl Pts',(52.1602259568374,-4.19999999995024,
73.3009530619475)) ;
#194895=CARTESIAN_POINT('Ctrl Pts',(50.050485176063,3.0000000000498,70.0092505885835)) ;
#194896=CARTESIAN_POINT('Ctrl Pts',(50.050485176063,-4.19999999995021,70.0092505885834)) ;
#194897=CARTESIAN_POINT('Ctrl Pts',(42.8151718885461,3.00000000004975,74.5426674236288)) ;
#194898=CARTESIAN_POINT('Ctrl Pts',(42.8151718885461,-4.19999999995025,
74.5426674236287)) ;
#194899=CARTESIAN_POINT('',(42.8151718885463,3.00000000004975,74.5426674236288)) ;
#194900=CARTESIAN_POINT('Origin',(44.8076225225366,3.00000000004971,78.0134346533848)) ;
#194901=CARTESIAN_POINT('',(42.8151718885463,-2.99999999995025,74.5426674236287)) ;
#194902=CARTESIAN_POINT('',(42.8151718885463,3.00000000004975,74.5426674236288)) ;
#194903=CARTESIAN_POINT('Origin',(44.8076225225365,-2.99999999995029,78.0134346533847)) ;
#194904=CARTESIAN_POINT('Origin',(43.8113972055423,3.00000000004974,76.2780510385053)) ;
#194905=CARTESIAN_POINT('',(44.8076225225385,3.00000000004972,78.0134346533818)) ;
#194906=CARTESIAN_POINT('',(42.8151718885463,3.00000000004975,74.5426674236288)) ;
#194907=CARTESIAN_POINT('',(44.8076225225385,-2.99999999995028,78.0134346533818)) ;
#194908=CARTESIAN_POINT('',(44.8076225225385,3.00000000004972,78.0134346533819)) ;
#194909=CARTESIAN_POINT('',(42.8151718885463,-2.99999999995025,74.5426674236288)) ;
#194910=CARTESIAN_POINT('Origin',(44.5085565950966,3.00000000004971,78.183601454246)) ;
#194911=CARTESIAN_POINT('',(44.2094906676548,3.00000000004971,78.3537682551101)) ;
#194912=CARTESIAN_POINT('',(44.8076225225385,3.00000000004972,78.0134346533819)) ;
#194913=CARTESIAN_POINT('',(44.2094906676548,-2.99999999995029,78.35376825511)) ;
#194914=CARTESIAN_POINT('',(44.2094906676548,3.00000000004971,78.3537682551101)) ;
#194915=CARTESIAN_POINT('',(44.8076225225385,-2.99999999995028,78.0134346533818)) ;
#194916=CARTESIAN_POINT('Ctrl Pts',(44.2094906676547,3.00000000004971,78.35376825511)) ;
#194917=CARTESIAN_POINT('Ctrl Pts',(44.2094906676547,-4.19999999995029,
78.3537682551099)) ;
#194918=CARTESIAN_POINT('Ctrl Pts',(44.2089016680448,3.00000000004971,78.3525907404827)) ;
#194919=CARTESIAN_POINT('Ctrl Pts',(44.2089016680448,-4.19999999995029,
78.3525907404826)) ;
#194920=CARTESIAN_POINT('Ctrl Pts',(44.2083109756305,3.00000000004971,78.3514140753339)) ;
#194921=CARTESIAN_POINT('Ctrl Pts',(44.2083109756305,-4.19999999995029,
78.3514140753338)) ;
#194922=CARTESIAN_POINT('Ctrl Pts',(42.4542041766734,3.00000000004975,74.8572159308281)) ;
#194923=CARTESIAN_POINT('Ctrl Pts',(42.4542041766734,-4.19999999995026,
74.857215930828)) ;
#194924=CARTESIAN_POINT('Ctrl Pts',(34.7846555972706,3.00000000004971,78.6095020549076)) ;
#194925=CARTESIAN_POINT('Ctrl Pts',(34.7846555972706,-4.1999999999503,78.6095020549075)) ;
#194926=CARTESIAN_POINT('',(34.7846555972707,3.00000000004971,78.6095020549077)) ;
#194927=CARTESIAN_POINT('Origin',(36.4033974133286,3.00000000004968,82.2695238615344)) ;
#194928=CARTESIAN_POINT('',(34.7846555972707,-2.99999999995029,78.6095020549076)) ;
#194929=CARTESIAN_POINT('',(34.7846555972707,3.00000000004971,78.6095020549076)) ;
#194930=CARTESIAN_POINT('Origin',(36.4033974133284,-2.99999999995033,82.2695238615347)) ;
#194931=CARTESIAN_POINT('Origin',(35.5940265053006,3.00000000004969,80.4395129582195)) ;
#194932=CARTESIAN_POINT('',(36.4033974133305,3.00000000004967,82.2695238615314)) ;
#194933=CARTESIAN_POINT('',(34.7846555972707,3.00000000004971,78.6095020549076)) ;
#194934=CARTESIAN_POINT('',(36.4033974133305,-2.99999999995033,82.2695238615314)) ;
#194935=CARTESIAN_POINT('',(36.4033974133305,3.00000000004967,82.2695238615314)) ;
#194936=CARTESIAN_POINT('',(34.7846555972707,-2.99999999995029,78.6095020549076)) ;
#194937=CARTESIAN_POINT('Origin',(36.0881825261374,3.00000000004967,82.4074975690443)) ;
#194938=CARTESIAN_POINT('',(35.7729676389444,3.00000000004967,82.5454712765571)) ;
#194939=CARTESIAN_POINT('',(36.4033974133305,3.00000000004967,82.2695238615314)) ;
#194940=CARTESIAN_POINT('',(35.7729676389444,-2.99999999995033,82.5454712765571)) ;
#194941=CARTESIAN_POINT('',(35.7729676389443,3.00000000004967,82.5454712765571)) ;
#194942=CARTESIAN_POINT('',(36.4033974133305,-2.99999999995033,82.2695238615314)) ;
#194943=CARTESIAN_POINT('Ctrl Pts',(35.7729676389443,3.00000000004967,82.5454712765571)) ;
#194944=CARTESIAN_POINT('Ctrl Pts',(35.7729676389443,-4.19999999995034,
82.545471276557)) ;
#194945=CARTESIAN_POINT('Ctrl Pts',(35.7725049497303,3.00000000004967,82.5442386452546)) ;
#194946=CARTESIAN_POINT('Ctrl Pts',(35.7725049497303,-4.19999999995034,
82.5442386452545)) ;
#194947=CARTESIAN_POINT('Ctrl Pts',(35.7720404881907,3.00000000004967,82.5430066818299)) ;
#194948=CARTESIAN_POINT('Ctrl Pts',(35.7720404881907,-4.19999999995034,
82.5430066818298)) ;
#194949=CARTESIAN_POINT('Ctrl Pts',(34.3927860322115,3.00000000004971,78.8845960322615)) ;
#194950=CARTESIAN_POINT('Ctrl Pts',(34.3927860322115,-4.1999999999503,78.8845960322614)) ;
#194951=CARTESIAN_POINT('Ctrl Pts',(26.373031340114,3.00000000004968,81.8146406133832)) ;
#194952=CARTESIAN_POINT('Ctrl Pts',(26.373031340114,-4.19999999995033,81.8146406133831)) ;
#194953=CARTESIAN_POINT('',(26.3730313401142,3.00000000004968,81.8146406133833)) ;
#194954=CARTESIAN_POINT('Origin',(27.6003290641584,3.00000000004964,85.6238170320596)) ;
#194955=CARTESIAN_POINT('',(26.3730313401142,-2.99999999995032,81.8146406133832)) ;
#194956=CARTESIAN_POINT('',(26.3730313401142,3.00000000004968,81.8146406133833)) ;
#194957=CARTESIAN_POINT('Origin',(27.6003290641572,-2.99999999995036,85.6238170320607)) ;
#194958=CARTESIAN_POINT('Origin',(26.9866802021375,3.00000000004966,83.7192288227197)) ;
#194959=CARTESIAN_POINT('',(27.6003290641612,3.00000000004964,85.6238170320561)) ;
#194960=CARTESIAN_POINT('',(26.3730313401142,3.00000000004968,81.8146406133833)) ;
#194961=CARTESIAN_POINT('',(27.6003290641612,-2.99999999995036,85.6238170320561)) ;
#194962=CARTESIAN_POINT('',(27.6003290641612,3.00000000004964,85.6238170320561)) ;
#194963=CARTESIAN_POINT('',(26.3730313401142,-2.99999999995032,81.8146406133832)) ;
#194964=CARTESIAN_POINT('Origin',(27.2724187774839,3.00000000004964,85.7280859774054)) ;
#194965=CARTESIAN_POINT('',(26.9445084908067,3.00000000004964,85.8323549227545)) ;
#194966=CARTESIAN_POINT('',(27.6003290641612,3.00000000004964,85.6238170320561)) ;
#194967=CARTESIAN_POINT('',(26.9445084908067,-2.99999999995036,85.8323549227545)) ;
#194968=CARTESIAN_POINT('',(26.9445084908067,3.00000000004964,85.8323549227546)) ;
#194969=CARTESIAN_POINT('',(27.6003290641612,-2.99999999995036,85.6238170320561)) ;
#194970=CARTESIAN_POINT('Ctrl Pts',(26.9445084908067,3.00000000004964,85.8323549227545)) ;
#194971=CARTESIAN_POINT('Ctrl Pts',(26.9445084908067,-4.19999999995036,
85.8323549227544)) ;
#194972=CARTESIAN_POINT('Ctrl Pts',(26.9441771813086,3.00000000004964,85.8310806797426)) ;
#194973=CARTESIAN_POINT('Ctrl Pts',(26.9441771813086,-4.19999999995036,
85.8310806797425)) ;
#194974=CARTESIAN_POINT('Ctrl Pts',(26.9438440393814,3.00000000004964,85.8298069156914)) ;
#194975=CARTESIAN_POINT('Ctrl Pts',(26.9438440393814,-4.19999999995036,
85.8298069156913)) ;
#194976=CARTESIAN_POINT('Ctrl Pts',(25.9545533268276,3.00000000004968,82.0472660737088)) ;
#194977=CARTESIAN_POINT('Ctrl Pts',(25.9545533268276,-4.19999999995032,
82.0472660737087)) ;
#194978=CARTESIAN_POINT('Ctrl Pts',(17.6724586326834,3.00000000004966,84.1229669302911)) ;
#194979=CARTESIAN_POINT('Ctrl Pts',(17.6724586326834,-4.19999999995034,
84.122966930291)) ;
#194980=CARTESIAN_POINT('',(17.6724586326837,3.00000000004966,84.1229669302912)) ;
#194981=CARTESIAN_POINT('Origin',(18.494865734023,3.00000000004962,88.0395638270497)) ;
#194982=CARTESIAN_POINT('',(17.6724586326837,-2.99999999995035,84.1229669302911)) ;
#194983=CARTESIAN_POINT('',(17.6724586326838,3.00000000004966,84.1229669302912)) ;
#194984=CARTESIAN_POINT('Origin',(18.4948657340247,-2.99999999995039,88.0395638270483)) ;
#194985=CARTESIAN_POINT('Origin',(18.0836621833541,3.00000000004964,86.0812653786697)) ;
#194986=CARTESIAN_POINT('',(18.4948657340249,3.00000000004962,88.0395638270482)) ;
#194987=CARTESIAN_POINT('',(17.6724586326838,3.00000000004966,84.1229669302912)) ;
#194988=CARTESIAN_POINT('',(18.4948657340249,-2.99999999995039,88.0395638270482)) ;
#194989=CARTESIAN_POINT('',(18.4948657340249,3.00000000004962,88.0395638270483)) ;
#194990=CARTESIAN_POINT('',(17.6724586326838,-2.99999999995035,84.1229669302912)) ;
#194991=CARTESIAN_POINT('Origin',(18.1578527015839,3.00000000004962,88.1089856178489)) ;
#194992=CARTESIAN_POINT('',(17.8208396691431,3.00000000004961,88.1784074086498)) ;
#194993=CARTESIAN_POINT('',(18.4948657340249,3.00000000004962,88.0395638270483)) ;
#194994=CARTESIAN_POINT('',(17.8208396691431,-2.99999999995039,88.1784074086497)) ;
#194995=CARTESIAN_POINT('',(17.8208396691431,3.00000000004962,88.1784074086499)) ;
#194996=CARTESIAN_POINT('',(18.4948657340249,-2.99999999995039,88.0395638270482)) ;
#194997=CARTESIAN_POINT('Ctrl Pts',(17.8208396691429,3.00000000004961,88.1784074086497)) ;
#194998=CARTESIAN_POINT('Ctrl Pts',(17.8208396691429,-4.19999999995039,
88.1784074086496)) ;
#194999=CARTESIAN_POINT('Ctrl Pts',(17.8206433692571,3.00000000004961,88.1771055148015)) ;
#195000=CARTESIAN_POINT('Ctrl Pts',(17.8206433692571,-4.19999999995039,
88.1771055148014)) ;
#195001=CARTESIAN_POINT('Ctrl Pts',(17.820445196915,3.00000000004961,88.1758039057497)) ;
#195002=CARTESIAN_POINT('Ctrl Pts',(17.820445196915,-4.19999999995039,88.1758039057496)) ;
#195003=CARTESIAN_POINT('Ctrl Pts',(17.2319571038551,3.00000000004966,84.3105751803646)) ;
#195004=CARTESIAN_POINT('Ctrl Pts',(17.2319571038551,-4.19999999995035,
84.3105751803645)) ;
#195005=CARTESIAN_POINT('Ctrl Pts',(8.77826277027357,3.00000000004964,85.5091904994544)) ;
#195006=CARTESIAN_POINT('Ctrl Pts',(8.77826277027357,-4.19999999995037,
85.5091904994543)) ;
#195007=CARTESIAN_POINT('',(8.77826277027361,3.00000000004964,85.5091904994544)) ;
#195008=CARTESIAN_POINT('Origin',(9.18676878460585,3.0000000000496,89.490296819095)) ;
#195009=CARTESIAN_POINT('',(8.77826277027361,-2.99999999995036,85.5091904994543)) ;
#195010=CARTESIAN_POINT('',(8.77826277027362,3.00000000004964,85.5091904994544)) ;
#195011=CARTESIAN_POINT('Origin',(9.18676878460804,-2.99999999995041,89.4902968190937)) ;
#195012=CARTESIAN_POINT('Origin',(8.98251577744044,3.00000000004962,87.4997436592745)) ;
#195013=CARTESIAN_POINT('',(9.18676878460724,3.0000000000496,89.4902968190945)) ;
#195014=CARTESIAN_POINT('',(8.77826277027362,3.00000000004964,85.5091904994544)) ;
#195015=CARTESIAN_POINT('',(9.18676878460724,-2.9999999999504,89.4902968190944)) ;
#195016=CARTESIAN_POINT('',(9.18676878460724,3.0000000000496,89.4902968190945)) ;
#195017=CARTESIAN_POINT('',(8.77826277027362,-2.99999999995036,85.5091904994543)) ;
#195018=CARTESIAN_POINT('Origin',(8.84434539171061,3.0000000000496,89.5241108556793)) ;
#195019=CARTESIAN_POINT('',(8.50192199881383,3.0000000000496,89.5579248922642)) ;
#195020=CARTESIAN_POINT('',(9.18676878460724,3.0000000000496,89.4902968190945)) ;
#195021=CARTESIAN_POINT('',(8.50192199881383,-2.9999999999504,89.5579248922642)) ;
#195022=CARTESIAN_POINT('',(8.50192199881383,3.0000000000496,89.5579248922642)) ;
#195023=CARTESIAN_POINT('',(9.18676878460724,-2.9999999999504,89.4902968190944)) ;
#195024=CARTESIAN_POINT('Ctrl Pts',(8.50192199881385,3.0000000000496,89.5579248922642)) ;
#195025=CARTESIAN_POINT('Ctrl Pts',(8.50192199881385,-4.19999999995041,
89.5579248922641)) ;
#195026=CARTESIAN_POINT('Ctrl Pts',(8.50186285924251,3.0000000000496,89.5566096114014)) ;
#195027=CARTESIAN_POINT('Ctrl Pts',(8.50186285924251,-4.19999999995041,
89.5566096114013)) ;
#195028=CARTESIAN_POINT('Ctrl Pts',(8.50180182770343,3.0000000000496,89.5552944180496)) ;
#195029=CARTESIAN_POINT('Ctrl Pts',(8.50180182770343,-4.19999999995041,
89.5552944180495)) ;
#195030=CARTESIAN_POINT('Ctrl Pts',(8.32056395283395,3.00000000004964,85.6497260640287)) ;
#195031=CARTESIAN_POINT('Ctrl Pts',(8.32056395283395,-4.19999999995037,
85.6497260640286)) ;
#195032=CARTESIAN_POINT('Ctrl Pts',(-0.212109576016898,3.00000000004964,
85.9581235653636)) ;
#195033=CARTESIAN_POINT('Ctrl Pts',(-0.212109576016898,-4.19999999995037,
85.9581235653635)) ;
#195034=CARTESIAN_POINT('',(-0.212109576016928,3.00000000004964,85.9581235653636)) ;
#195035=CARTESIAN_POINT('Origin',(-0.221980326067951,3.00000000004959,89.9601214739474)) ;
#195036=CARTESIAN_POINT('',(-0.212109576016928,-2.99999999995036,85.9581235653635)) ;
#195037=CARTESIAN_POINT('',(-0.212109576016928,3.00000000004963,85.9581235653635)) ;
#195038=CARTESIAN_POINT('Origin',(-0.221980326066147,-2.99999999995041,
89.9601214739464)) ;
#195039=CARTESIAN_POINT('Origin',(-0.217044951043372,3.00000000004962,87.9591225196562)) ;
#195040=CARTESIAN_POINT('',(-0.221980326069911,3.00000000004959,89.9601214739486)) ;
#195041=CARTESIAN_POINT('',(-0.212109576016928,3.00000000004963,85.9581235653635)) ;
#195042=CARTESIAN_POINT('',(-0.221980326069911,-2.9999999999504,89.9601214739485)) ;
#195043=CARTESIAN_POINT('',(-0.221980326069911,3.00000000004959,89.9601214739485)) ;
#195044=CARTESIAN_POINT('',(-0.212109576016928,-2.99999999995036,85.9581235653634)) ;
#195045=CARTESIAN_POINT('Origin',(-0.566062417072776,3.0000000000496,89.9579572826566)) ;
#195046=CARTESIAN_POINT('',(-0.91014450807586,3.00000000004959,89.9557930913646)) ;
#195047=CARTESIAN_POINT('',(-0.221980326069911,3.00000000004959,89.9601214739485)) ;
#195048=CARTESIAN_POINT('',(-0.91014450807586,-2.9999999999504,89.9557930913645)) ;
#195049=CARTESIAN_POINT('',(-0.910144508075859,3.00000000004959,89.9557930913646)) ;
#195050=CARTESIAN_POINT('',(-0.221980326069911,-2.9999999999504,89.9601214739484)) ;
#195051=CARTESIAN_POINT('Ctrl Pts',(-0.91014450807588,3.0000000000496,89.9557930913647)) ;
#195052=CARTESIAN_POINT('Ctrl Pts',(-0.91014450807588,-4.1999999999504,
89.9557930913646)) ;
#195053=CARTESIAN_POINT('Ctrl Pts',(-0.910065839387319,3.0000000000496,
89.9544788339794)) ;
#195054=CARTESIAN_POINT('Ctrl Pts',(-0.910065839387319,-4.1999999999504,
89.9544788339793)) ;
#195055=CARTESIAN_POINT('Ctrl Pts',(-0.909989061449521,3.0000000000496,
89.9531644658614)) ;
#195056=CARTESIAN_POINT('Ctrl Pts',(-0.909989061449521,-4.19999999995041,
89.9531644658614)) ;
#195057=CARTESIAN_POINT('Ctrl Pts',(-0.681991038044035,3.00000000004963,
86.0500467073845)) ;
#195058=CARTESIAN_POINT('Ctrl Pts',(-0.681991038044035,-4.19999999995037,
86.0500467073845)) ;
#195059=CARTESIAN_POINT('Ctrl Pts',(-9.20015800540569,3.00000000004964,
85.4648475234035)) ;
#195060=CARTESIAN_POINT('Ctrl Pts',(-9.20015800540569,-4.19999999995036,
85.4648475234034)) ;
#195061=CARTESIAN_POINT('',(-9.2001580054058,3.00000000004964,85.4648475234036)) ;
#195062=CARTESIAN_POINT('Origin',(-9.62829737384348,3.0000000000496,89.4438902943758)) ;
#195063=CARTESIAN_POINT('',(-9.2001580054058,-2.99999999995036,85.4648475234035)) ;
#195064=CARTESIAN_POINT('',(-9.2001580054058,3.00000000004964,85.4648475234036)) ;
#195065=CARTESIAN_POINT('Origin',(-9.62829737384347,-2.9999999999504,89.4438902943758)) ;
#195066=CARTESIAN_POINT('Origin',(-9.41422768962381,3.00000000004962,87.4543689088892)) ;
#195067=CARTESIAN_POINT('',(-9.62829737384186,3.0000000000496,89.443890294375)) ;
#195068=CARTESIAN_POINT('',(-9.2001580054058,3.00000000004964,85.4648475234036)) ;
#195069=CARTESIAN_POINT('',(-9.62829737384186,-2.9999999999504,89.443890294375)) ;
#195070=CARTESIAN_POINT('',(-9.62829737384186,3.0000000000496,89.443890294375)) ;
#195071=CARTESIAN_POINT('',(-9.2001580054058,-2.99999999995036,85.4648475234035)) ;
#195072=CARTESIAN_POINT('Origin',(-9.97026832755854,3.0000000000496,89.4057715865388)) ;
#195073=CARTESIAN_POINT('',(-10.3122392812752,3.0000000000496,89.3676528787028)) ;
#195074=CARTESIAN_POINT('',(-9.62829737384186,3.0000000000496,89.443890294375)) ;
#195075=CARTESIAN_POINT('',(-10.3122392812752,-2.9999999999504,89.3676528787027)) ;
#195076=CARTESIAN_POINT('',(-10.3122392812752,3.0000000000496,89.3676528787028)) ;
#195077=CARTESIAN_POINT('',(-9.62829737384186,-2.9999999999504,89.443890294375)) ;
#195078=CARTESIAN_POINT('Ctrl Pts',(-10.3122392812751,3.0000000000496,89.3676528787027)) ;
#195079=CARTESIAN_POINT('Ctrl Pts',(-10.3122392812751,-4.19999999995041,
89.3676528787026)) ;
#195080=CARTESIAN_POINT('Ctrl Pts',(-10.3120236662372,3.0000000000496,89.3663540440742)) ;
#195081=CARTESIAN_POINT('Ctrl Pts',(-10.3120236662372,-4.19999999995041,
89.3663540440741)) ;
#195082=CARTESIAN_POINT('Ctrl Pts',(-10.3118099200173,3.0000000000496,89.3650549016823)) ;
#195083=CARTESIAN_POINT('Ctrl Pts',(-10.3118099200173,-4.19999999995041,
89.3650549016822)) ;
#195084=CARTESIAN_POINT('Ctrl Pts',(-9.67707399239374,3.00000000004964,
85.5071511136907)) ;
#195085=CARTESIAN_POINT('Ctrl Pts',(-9.67707399239374,-4.19999999995037,
85.5071511136907)) ;
#195086=CARTESIAN_POINT('Ctrl Pts',(-18.0874075784306,3.00000000004966,
84.0347668091144)) ;
#195087=CARTESIAN_POINT('Ctrl Pts',(-18.0874075784306,-4.19999999995035,
84.0347668091143)) ;
#195088=CARTESIAN_POINT('',(-18.0874075784307,3.00000000004966,84.0347668091144)) ;
#195089=CARTESIAN_POINT('Origin',(-18.9291247807382,3.00000000004961,87.9472592172066)) ;
#195090=CARTESIAN_POINT('',(-18.0874075784307,-2.99999999995034,84.0347668091144)) ;
#195091=CARTESIAN_POINT('',(-18.0874075784307,3.00000000004966,84.0347668091144)) ;
#195092=CARTESIAN_POINT('Origin',(-18.9291247807369,-2.99999999995038,87.9472592172062)) ;
#195093=CARTESIAN_POINT('Origin',(-18.5082661795829,3.00000000004964,85.9910130131597)) ;
#195094=CARTESIAN_POINT('',(-18.9291247807354,3.00000000004962,87.9472592172052)) ;
#195095=CARTESIAN_POINT('',(-18.0874075784307,3.00000000004966,84.0347668091144)) ;
#195096=CARTESIAN_POINT('',(-18.9291247807354,-2.99999999995038,87.9472592172051)) ;
#195097=CARTESIAN_POINT('',(-18.9291247807354,3.00000000004962,87.9472592172052)) ;
#195098=CARTESIAN_POINT('',(-18.0874075784307,-2.99999999995034,84.0347668091144)) ;
#195099=CARTESIAN_POINT('Origin',(-19.2652378918346,3.00000000004962,87.8736036293648)) ;
#195100=CARTESIAN_POINT('',(-19.6013510029339,3.00000000004962,87.7999480415246)) ;
#195101=CARTESIAN_POINT('',(-18.9291247807354,3.00000000004962,87.9472592172052)) ;
#195102=CARTESIAN_POINT('',(-19.6013510029339,-2.99999999995038,87.7999480415245)) ;
#195103=CARTESIAN_POINT('',(-19.6013510029339,3.00000000004962,87.7999480415246)) ;
#195104=CARTESIAN_POINT('',(-18.9291247807354,-2.99999999995038,87.9472592172051)) ;
#195105=CARTESIAN_POINT('Ctrl Pts',(-19.6013510029339,3.00000000004962,
87.7999480415246)) ;
#195106=CARTESIAN_POINT('Ctrl Pts',(-19.6013510029339,-4.1999999999504,
87.7999480415245)) ;
#195107=CARTESIAN_POINT('Ctrl Pts',(-19.6010008038698,3.00000000004962,
87.7986788599565)) ;
#195108=CARTESIAN_POINT('Ctrl Pts',(-19.6010008038698,-4.19999999995039,
87.7986788599564)) ;
#195109=CARTESIAN_POINT('Ctrl Pts',(-19.6006524312165,3.00000000004962,
87.7974091769667)) ;
#195110=CARTESIAN_POINT('Ctrl Pts',(-19.6006524312165,-4.1999999999504,
87.7974091769666)) ;
#195111=CARTESIAN_POINT('Ctrl Pts',(-18.5661328990248,3.00000000004966,
84.0269873606799)) ;
#195112=CARTESIAN_POINT('Ctrl Pts',(-18.5661328990248,-4.19999999995036,
84.0269873606798)) ;
#195113=CARTESIAN_POINT('Ctrl Pts',(-26.7764877289929,3.00000000004968,
81.6835496860654)) ;
#195114=CARTESIAN_POINT('Ctrl Pts',(-26.7764877289929,-4.19999999995033,
81.6835496860653)) ;
#195115=CARTESIAN_POINT('',(-26.7764877289929,3.00000000004968,81.6835496860653)) ;
#195116=CARTESIAN_POINT('Origin',(-28.0225607353604,3.00000000004964,85.4866256457122)) ;
#195117=CARTESIAN_POINT('',(-26.7764877289929,-2.99999999995032,81.6835496860653)) ;
#195118=CARTESIAN_POINT('',(-26.7764877289929,3.00000000004968,81.6835496860653)) ;
#195119=CARTESIAN_POINT('Origin',(-28.0225607353587,-2.99999999995036,85.4866256457119)) ;
#195120=CARTESIAN_POINT('Origin',(-27.3995242321751,3.00000000004966,83.5850876658882)) ;
#195121=CARTESIAN_POINT('',(-28.0225607353573,3.00000000004964,85.4866256457111)) ;
#195122=CARTESIAN_POINT('',(-26.7764877289929,3.00000000004968,81.6835496860653)) ;
#195123=CARTESIAN_POINT('',(-28.0225607353573,-2.99999999995036,85.486625645711)) ;
#195124=CARTESIAN_POINT('',(-28.0225607353573,3.00000000004964,85.4866256457111)) ;
#195125=CARTESIAN_POINT('',(-26.7764877289929,-2.99999999995032,81.6835496860653)) ;
#195126=CARTESIAN_POINT('Origin',(-28.3491334782579,3.00000000004964,85.3782401639004)) ;
#195127=CARTESIAN_POINT('',(-28.6757062211584,3.00000000004964,85.2698546820896)) ;
#195128=CARTESIAN_POINT('',(-28.0225607353573,3.00000000004964,85.4866256457111)) ;
#195129=CARTESIAN_POINT('',(-28.6757062211584,-2.99999999995036,85.2698546820896)) ;
#195130=CARTESIAN_POINT('',(-28.6757062211584,3.00000000004964,85.2698546820896)) ;
#195131=CARTESIAN_POINT('',(-28.0225607353573,-2.99999999995036,85.486625645711)) ;
#195132=CARTESIAN_POINT('Ctrl Pts',(-28.6757062211583,3.00000000004964,
85.2698546820896)) ;
#195133=CARTESIAN_POINT('Ctrl Pts',(-28.6757062211583,-4.1999999999504,
85.2698546820895)) ;
#195134=CARTESIAN_POINT('Ctrl Pts',(-28.6752252749224,3.00000000004964,
85.2686290590011)) ;
#195135=CARTESIAN_POINT('Ctrl Pts',(-28.6752252749224,-4.1999999999504,
85.268629059001)) ;
#195136=CARTESIAN_POINT('Ctrl Pts',(-28.6747460926791,3.00000000004964,
85.2674027463255)) ;
#195137=CARTESIAN_POINT('Ctrl Pts',(-28.6747460926791,-4.1999999999504,
85.2674027463254)) ;
#195138=CARTESIAN_POINT('Ctrl Pts',(-27.2517773684014,3.00000000004968,
81.6257724321745)) ;
#195139=CARTESIAN_POINT('Ctrl Pts',(-27.2517773684014,-4.19999999995036,
81.6257724321744)) ;
#195140=CARTESIAN_POINT('Ctrl Pts',(-35.172199076656,3.00000000004971,78.4369565810807)) ;
#195141=CARTESIAN_POINT('Ctrl Pts',(-35.172199076656,-4.19999999995033,
78.4369565810806)) ;
#195142=CARTESIAN_POINT('',(-35.1721990766561,3.00000000004971,78.4369565810808)) ;
#195143=CARTESIAN_POINT('Origin',(-36.8089756504653,3.00000000004967,82.0889487962232)) ;
#195144=CARTESIAN_POINT('',(-35.1721990766561,-2.99999999995029,78.4369565810807)) ;
#195145=CARTESIAN_POINT('',(-35.1721990766561,3.00000000004971,78.4369565810808)) ;
#195146=CARTESIAN_POINT('Origin',(-36.8089756504651,-2.99999999995032,82.0889487962231)) ;
#195147=CARTESIAN_POINT('Origin',(-35.9905873635603,3.0000000000497,80.2629526886517)) ;
#195148=CARTESIAN_POINT('',(-36.8089756504645,3.00000000004968,82.0889487962226)) ;
#195149=CARTESIAN_POINT('',(-35.1721990766561,3.00000000004971,78.4369565810808)) ;
#195150=CARTESIAN_POINT('',(-36.8089756504645,-2.99999999995033,82.0889487962225)) ;
#195151=CARTESIAN_POINT('',(-36.8089756504645,3.00000000004968,82.0889487962226)) ;
#195152=CARTESIAN_POINT('',(-35.1721990766561,-2.99999999995029,78.4369565810807)) ;
#195153=CARTESIAN_POINT('Origin',(-37.1224300258554,3.00000000004968,81.9470209144612)) ;
#195154=CARTESIAN_POINT('',(-37.4358844012463,3.00000000004968,81.8050930326999)) ;
#195155=CARTESIAN_POINT('',(-36.8089756504645,3.00000000004968,82.0889487962226)) ;
#195156=CARTESIAN_POINT('',(-37.4358844012463,-2.99999999995032,81.8050930326999)) ;
#195157=CARTESIAN_POINT('',(-37.4358844012463,3.00000000004968,81.8050930326999)) ;
#195158=CARTESIAN_POINT('',(-36.8089756504645,-2.99999999995033,82.0889487962225)) ;
#195159=CARTESIAN_POINT('Ctrl Pts',(-37.4358844012462,3.00000000004968,
81.8050930326999)) ;
#195160=CARTESIAN_POINT('Ctrl Pts',(-37.4358844012462,-4.19999999995034,
81.8050930326998)) ;
#195161=CARTESIAN_POINT('Ctrl Pts',(-37.4352779771863,3.00000000004968,
81.8039243962738)) ;
#195162=CARTESIAN_POINT('Ctrl Pts',(-37.4352779771863,-4.19999999995034,
81.8039243962737)) ;
#195163=CARTESIAN_POINT('Ctrl Pts',(-37.4346732353739,3.00000000004968,
81.8027548896506)) ;
#195164=CARTESIAN_POINT('Ctrl Pts',(-37.4346732353739,-4.19999999995034,
81.8027548896505)) ;
#195165=CARTESIAN_POINT('Ctrl Pts',(-35.6388456621282,3.00000000004971,
78.3298145414176)) ;
#195166=CARTESIAN_POINT('Ctrl Pts',(-35.6388456621282,-4.1999999999503,
78.3298145414175)) ;
#195167=CARTESIAN_POINT('Ctrl Pts',(-43.1825564509794,3.00000000004975,
74.3305578476115)) ;
#195168=CARTESIAN_POINT('Ctrl Pts',(-43.1825564509794,-4.19999999995026,
74.3305578476115)) ;
#195169=CARTESIAN_POINT('',(-43.1825564509793,3.00000000004975,74.3305578476115)) ;
#195170=CARTESIAN_POINT('Origin',(-45.1921037255759,3.00000000004972,77.7914543273124)) ;
#195171=CARTESIAN_POINT('',(-43.1825564509793,-2.99999999995025,74.3305578476114)) ;
#195172=CARTESIAN_POINT('',(-43.1825564509793,3.00000000004975,74.3305578476115)) ;
#195173=CARTESIAN_POINT('Origin',(-45.1921037255757,-2.99999999995028,77.7914543273123)) ;
#195174=CARTESIAN_POINT('Origin',(-44.1873300882757,3.00000000004974,76.0610060874618)) ;
#195175=CARTESIAN_POINT('',(-45.192103725572,3.00000000004972,77.7914543273121)) ;
#195176=CARTESIAN_POINT('',(-43.1825564509793,3.00000000004975,74.3305578476115)) ;
#195177=CARTESIAN_POINT('',(-45.192103725572,-2.99999999995028,77.791454327312)) ;
#195178=CARTESIAN_POINT('',(-45.192103725572,3.00000000004972,77.791454327312)) ;
#195179=CARTESIAN_POINT('',(-43.1825564509793,-2.99999999995025,74.3305578476114)) ;
#195180=CARTESIAN_POINT('Origin',(-45.489005461722,3.00000000004972,77.617539037173)) ;
#195181=CARTESIAN_POINT('',(-45.7859071978719,3.00000000004972,77.443623747034)) ;
#195182=CARTESIAN_POINT('',(-45.192103725572,3.00000000004972,77.791454327312)) ;
#195183=CARTESIAN_POINT('',(-45.7859071978719,-2.99999999995028,77.4436237470339)) ;
#195184=CARTESIAN_POINT('',(-45.7859071978719,3.00000000004972,77.4436237470339)) ;
#195185=CARTESIAN_POINT('',(-45.192103725572,-2.99999999995028,77.791454327312)) ;
#195186=CARTESIAN_POINT('Ctrl Pts',(-45.7859071978719,3.00000000004972,
77.443623747034)) ;
#195187=CARTESIAN_POINT('Ctrl Pts',(-45.7859071978719,-4.19999999995028,
77.443623747034)) ;
#195188=CARTESIAN_POINT('Ctrl Pts',(-45.7851819400964,3.00000000004972,
77.4425249010956)) ;
#195189=CARTESIAN_POINT('Ctrl Pts',(-45.7851819400964,-4.19999999995028,
77.4425249010955)) ;
#195190=CARTESIAN_POINT('Ctrl Pts',(-45.7844582643927,3.00000000004972,
77.4414250138846)) ;
#195191=CARTESIAN_POINT('Ctrl Pts',(-45.7844582643927,-4.19999999995028,
77.4414250138846)) ;
#195192=CARTESIAN_POINT('Ctrl Pts',(-43.6354473048728,3.00000000004976,
74.1752248927841)) ;
#195193=CARTESIAN_POINT('Ctrl Pts',(-43.6354473048728,-4.19999999995024,
74.175224892784)) ;
#195194=CARTESIAN_POINT('Ctrl Pts',(-50.7197967002948,3.00000000004981,
69.4093440495017)) ;
#195195=CARTESIAN_POINT('Ctrl Pts',(-50.7197967002948,-4.1999999999502,
69.4093440495016)) ;
#195196=CARTESIAN_POINT('',(-50.7197967002948,3.00000000004981,69.4093440495017)) ;
#195197=CARTESIAN_POINT('Origin',(-53.0800976552041,3.00000000004977,72.64122648769)) ;
#195198=CARTESIAN_POINT('',(-50.7197967002948,-2.9999999999502,69.4093440495017)) ;
#195199=CARTESIAN_POINT('',(-50.7197967002948,3.00000000004981,69.4093440495017)) ;
#195200=CARTESIAN_POINT('Origin',(-53.0800976552046,-2.99999999995023,72.6412264876899)) ;
#195201=CARTESIAN_POINT('Origin',(-51.8999471777507,3.00000000004979,71.0252852685956)) ;
#195202=CARTESIAN_POINT('',(-53.0800976552065,3.00000000004977,72.6412264876896)) ;
#195203=CARTESIAN_POINT('',(-50.7197967002948,3.00000000004981,69.4093440495017)) ;
#195204=CARTESIAN_POINT('',(-53.0800976552065,-2.99999999995023,72.6412264876895)) ;
#195205=CARTESIAN_POINT('',(-53.0800976552065,3.00000000004977,72.6412264876896)) ;
#195206=CARTESIAN_POINT('',(-50.7197967002948,-2.9999999999502,69.4093440495017)) ;
#195207=CARTESIAN_POINT('Origin',(-53.3571938345634,3.00000000004977,72.4372292414858)) ;
#195208=CARTESIAN_POINT('',(-53.6342900139203,3.00000000004978,72.2332319952821)) ;
#195209=CARTESIAN_POINT('',(-53.0800976552065,3.00000000004977,72.6412264876896)) ;
#195210=CARTESIAN_POINT('',(-53.6342900139203,-2.99999999995022,72.233231995282)) ;
#195211=CARTESIAN_POINT('',(-53.6342900139203,3.00000000004978,72.2332319952821)) ;
#195212=CARTESIAN_POINT('',(-53.0800976552065,-2.99999999995023,72.6412264876895)) ;
#195213=CARTESIAN_POINT('Ctrl Pts',(-53.6342900139204,3.00000000004978,
72.233231995282)) ;
#195214=CARTESIAN_POINT('Ctrl Pts',(-53.6342900139204,-4.19999999995022,
72.2332319952819)) ;
#195215=CARTESIAN_POINT('Ctrl Pts',(-53.6334538685056,3.00000000004978,
72.2322149790174)) ;
#195216=CARTESIAN_POINT('Ctrl Pts',(-53.6334538685056,-4.19999999995023,
72.2322149790173)) ;
#195217=CARTESIAN_POINT('Ctrl Pts',(-53.6326191876533,3.00000000004978,
72.2311967618127)) ;
#195218=CARTESIAN_POINT('Ctrl Pts',(-53.6326191876533,-4.19999999995023,
72.2311967618126)) ;
#195219=CARTESIAN_POINT('Ctrl Pts',(-51.1539698556413,3.00000000004981,
69.2075220398674)) ;
#195220=CARTESIAN_POINT('Ctrl Pts',(-51.1539698556413,-4.19999999995019,
69.2075220398673)) ;
#195221=CARTESIAN_POINT('Ctrl Pts',(-57.7013402431623,3.00000000004986,
63.7272330349523)) ;
#195222=CARTESIAN_POINT('Ctrl Pts',(-57.7013402431623,-4.19999999995014,
63.7272330349523)) ;
#195223=CARTESIAN_POINT('',(-57.7013402431622,3.00000000004986,63.7272330349524)) ;
#195224=CARTESIAN_POINT('Origin',(-60.3865349272081,3.00000000004984,66.6946922513203)) ;
#195225=CARTESIAN_POINT('',(-57.7013402431622,-2.99999999995014,63.7272330349524)) ;
#195226=CARTESIAN_POINT('',(-57.7013402431622,3.00000000004986,63.7272330349524)) ;
#195227=CARTESIAN_POINT('Origin',(-60.3865349272089,-2.99999999995017,66.69469225132)) ;
#195228=CARTESIAN_POINT('Origin',(-59.0439375851841,3.00000000004985,65.2109626431365)) ;
#195229=CARTESIAN_POINT('',(-60.3865349272058,3.00000000004983,66.6946922513205)) ;
#195230=CARTESIAN_POINT('',(-57.7013402431622,3.00000000004986,63.7272330349524)) ;
#195231=CARTESIAN_POINT('',(-60.3865349272058,-2.99999999995017,66.6946922513204)) ;
#195232=CARTESIAN_POINT('',(-60.3865349272058,3.00000000004983,66.6946922513205)) ;
#195233=CARTESIAN_POINT('',(-57.7013402431622,-2.99999999995014,63.7272330349524)) ;
#195234=CARTESIAN_POINT('Origin',(-60.6407896260427,3.00000000004984,66.4628480855705)) ;
#195235=CARTESIAN_POINT('',(-60.8950443248795,3.00000000004984,66.2310039198205)) ;
#195236=CARTESIAN_POINT('',(-60.3865349272058,3.00000000004983,66.6946922513205)) ;
#195237=CARTESIAN_POINT('',(-60.8950443248795,-2.99999999995016,66.2310039198205)) ;
#195238=CARTESIAN_POINT('',(-60.8950443248795,3.00000000004984,66.2310039198205)) ;
#195239=CARTESIAN_POINT('',(-60.3865349272058,-2.99999999995017,66.6946922513204)) ;
#195240=CARTESIAN_POINT('Ctrl Pts',(-60.8950443248795,3.00000000004984,
66.2310039198205)) ;
#195241=CARTESIAN_POINT('Ctrl Pts',(-60.8950443248795,-4.19999999995016,
66.2310039198204)) ;
#195242=CARTESIAN_POINT('Ctrl Pts',(-60.8941064528096,3.00000000004984,
66.2300798758727)) ;
#195243=CARTESIAN_POINT('Ctrl Pts',(-60.8941064528096,-4.19999999995016,
66.2300798758727)) ;
#195244=CARTESIAN_POINT('Ctrl Pts',(-60.8931699117466,3.00000000004984,
66.2291544844751)) ;
#195245=CARTESIAN_POINT('Ctrl Pts',(-60.8931699117466,-4.19999999995016,
66.2291544844751)) ;
#195246=CARTESIAN_POINT('Ctrl Pts',(-58.112038808014,3.00000000004987,63.4811331746838)) ;
#195247=CARTESIAN_POINT('Ctrl Pts',(-58.112038808014,-4.19999999995014,
63.4811331746838)) ;
#195248=CARTESIAN_POINT('Ctrl Pts',(-64.0506958275439,3.00000000004993,
57.3464792012979)) ;
#195249=CARTESIAN_POINT('Ctrl Pts',(-64.0506958275439,-4.19999999995007,
57.3464792012979)) ;
#195250=CARTESIAN_POINT('',(-64.050695827544,3.00000000004993,57.346479201298)) ;
#195251=CARTESIAN_POINT('Origin',(-67.0313646858506,3.0000000000499,60.0170030916901)) ;
#195252=CARTESIAN_POINT('',(-64.050695827544,-2.99999999995007,57.3464792012979)) ;
#195253=CARTESIAN_POINT('',(-64.050695827544,3.00000000004993,57.3464792012979)) ;
#195254=CARTESIAN_POINT('Origin',(-67.0313646858511,-2.9999999999501,60.0170030916897)) ;
#195255=CARTESIAN_POINT('Origin',(-65.5410302566959,3.00000000004991,58.6817411464945)) ;
#195256=CARTESIAN_POINT('',(-67.0313646858481,3.0000000000499,60.017003091691)) ;
#195257=CARTESIAN_POINT('',(-64.050695827544,3.00000000004993,57.3464792012979)) ;
#195258=CARTESIAN_POINT('',(-67.0313646858481,-2.9999999999501,60.017003091691)) ;
#195259=CARTESIAN_POINT('',(-67.0313646858481,3.0000000000499,60.017003091691)) ;
#195260=CARTESIAN_POINT('',(-64.050695827544,-2.99999999995007,57.3464792012979)) ;
#195261=CARTESIAN_POINT('Origin',(-67.2599922364783,3.0000000000499,59.7598521395911)) ;
#195262=CARTESIAN_POINT('',(-67.4886197871086,3.00000000004991,59.5027011874913)) ;
#195263=CARTESIAN_POINT('',(-67.0313646858481,3.0000000000499,60.017003091691)) ;
#195264=CARTESIAN_POINT('',(-67.4886197871086,-2.99999999995009,59.5027011874912)) ;
#195265=CARTESIAN_POINT('',(-67.4886197871085,3.00000000004991,59.5027011874913)) ;
#195266=CARTESIAN_POINT('',(-67.0313646858481,-2.9999999999501,60.0170030916909)) ;
#195267=CARTESIAN_POINT('Ctrl Pts',(-67.4886197871085,3.0000000000499,59.5027011874913)) ;
#195268=CARTESIAN_POINT('Ctrl Pts',(-67.4886197871085,-4.1999999999501,
59.5027011874912)) ;
#195269=CARTESIAN_POINT('Ctrl Pts',(-67.4875904639056,3.00000000004991,
59.5018802398793)) ;
#195270=CARTESIAN_POINT('Ctrl Pts',(-67.4875904639056,-4.1999999999501,
59.5018802398792)) ;
#195271=CARTESIAN_POINT('Ctrl Pts',(-67.4865623235721,3.00000000004991,
59.5010578130706)) ;
#195272=CARTESIAN_POINT('Ctrl Pts',(-67.4865623235721,-4.19999999995009,
59.5010578130705)) ;
#195273=CARTESIAN_POINT('Ctrl Pts',(-64.4334201024814,3.00000000004993,
57.0587978119635)) ;
#195274=CARTESIAN_POINT('Ctrl Pts',(-64.4334201024814,-4.19999999995007,
57.0587978119634)) ;
#195275=CARTESIAN_POINT('Ctrl Pts',(-69.6982985849688,3.00000000005,50.3369914227983)) ;
#195276=CARTESIAN_POINT('Ctrl Pts',(-69.6982985849688,-4.19999999995,50.3369914227982)) ;
#195277=CARTESIAN_POINT('',(-69.6982985849687,3.00000000005,50.3369914227984)) ;
#195278=CARTESIAN_POINT('Origin',(-72.9417847857762,3.00000000004998,52.6813211686304)) ;
#195279=CARTESIAN_POINT('',(-69.6982985849687,-2.99999999995,50.3369914227983)) ;
#195280=CARTESIAN_POINT('',(-69.6982985849687,3.00000000005,50.3369914227984)) ;
#195281=CARTESIAN_POINT('Origin',(-72.9417847857764,-2.99999999995003,52.6813211686303)) ;
#195282=CARTESIAN_POINT('Origin',(-71.3200416853732,3.00000000004999,51.509156295714)) ;
#195283=CARTESIAN_POINT('',(-72.9417847857773,3.00000000004998,52.6813211686299)) ;
#195284=CARTESIAN_POINT('',(-69.6982985849687,3.00000000005,50.3369914227984)) ;
#195285=CARTESIAN_POINT('',(-72.9417847857773,-2.99999999995002,52.6813211686298)) ;
#195286=CARTESIAN_POINT('',(-72.9417847857773,3.00000000004998,52.6813211686299)) ;
#195287=CARTESIAN_POINT('',(-69.6982985849687,-2.99999999995,50.3369914227983)) ;
#195288=CARTESIAN_POINT('Origin',(-73.1422802969127,3.00000000004998,52.4016808298238)) ;
#195289=CARTESIAN_POINT('',(-73.3427758080476,3.00000000004998,52.1220404910179)) ;
#195290=CARTESIAN_POINT('',(-72.9417847857773,3.00000000004998,52.6813211686299)) ;
#195291=CARTESIAN_POINT('',(-73.3427758080476,-2.99999999995002,52.1220404910178)) ;
#195292=CARTESIAN_POINT('',(-73.3427758080477,3.00000000004998,52.1220404910179)) ;
#195293=CARTESIAN_POINT('',(-72.9417847857773,-2.99999999995003,52.6813211686298)) ;
#195294=CARTESIAN_POINT('Ctrl Pts',(-73.3427758080479,3.00000000004998,
52.1220404910178)) ;
#195295=CARTESIAN_POINT('Ctrl Pts',(-73.3427758080479,-4.19999999995002,
52.1220404910177)) ;
#195296=CARTESIAN_POINT('Ctrl Pts',(-73.3416663111934,3.00000000004998,
52.1213316342151)) ;
#195297=CARTESIAN_POINT('Ctrl Pts',(-73.3416663111934,-4.19999999995002,
52.121331634215)) ;
#195298=CARTESIAN_POINT('Ctrl Pts',(-73.3405578361091,3.00000000004998,
52.1206211826759)) ;
#195299=CARTESIAN_POINT('Ctrl Pts',(-73.3405578361091,-4.19999999995002,
52.1206211826759)) ;
#195300=CARTESIAN_POINT('Ctrl Pts',(-70.0488553627454,3.00000000005,50.0108804019009)) ;
#195301=CARTESIAN_POINT('Ctrl Pts',(-70.0488553627454,-4.19999999995,50.0108804019008)) ;
#195302=CARTESIAN_POINT('Ctrl Pts',(-74.5822721977904,3.00000000005008,
42.7755671143843)) ;
#195303=CARTESIAN_POINT('Ctrl Pts',(-74.5822721977904,-4.19999999994992,
42.7755671143842)) ;
#195304=CARTESIAN_POINT('',(-74.5822721977904,3.00000000005008,42.7755671143843)) ;
#195305=CARTESIAN_POINT('Origin',(-78.0530394275431,3.00000000005006,44.7680177483762)) ;
#195306=CARTESIAN_POINT('',(-74.5822721977904,-2.99999999994992,42.7755671143842)) ;
#195307=CARTESIAN_POINT('',(-74.5822721977904,3.00000000005008,42.7755671143843)) ;
#195308=CARTESIAN_POINT('Origin',(-78.0530394275428,-2.99999999994995,44.7680177483764)) ;
#195309=CARTESIAN_POINT('Origin',(-76.3176558126671,3.00000000005007,43.7717924313804)) ;
#195310=CARTESIAN_POINT('',(-78.0530394275436,3.00000000005006,44.7680177483765)) ;
#195311=CARTESIAN_POINT('',(-74.5822721977904,3.00000000005008,42.7755671143843)) ;
#195312=CARTESIAN_POINT('',(-78.0530394275436,-2.99999999994994,44.7680177483764)) ;
#195313=CARTESIAN_POINT('',(-78.0530394275436,3.00000000005006,44.7680177483765)) ;
#195314=CARTESIAN_POINT('',(-74.5822721977904,-2.99999999994992,42.7755671143843)) ;
#195315=CARTESIAN_POINT('Origin',(-78.2232062284076,3.00000000005006,44.4689518209346)) ;
#195316=CARTESIAN_POINT('',(-78.3933730292715,3.00000000005006,44.1698858934927)) ;
#195317=CARTESIAN_POINT('',(-78.0530394275436,3.00000000005006,44.7680177483765)) ;
#195318=CARTESIAN_POINT('',(-78.3933730292715,-2.99999999994994,44.1698858934927)) ;
#195319=CARTESIAN_POINT('',(-78.3933730292715,3.00000000005006,44.1698858934927)) ;
#195320=CARTESIAN_POINT('',(-78.0530394275436,-2.99999999994994,44.7680177483764)) ;
#195321=CARTESIAN_POINT('Ctrl Pts',(-78.3933730292716,3.00000000005006,
44.1698858934927)) ;
#195322=CARTESIAN_POINT('Ctrl Pts',(-78.3933730292716,-4.19999999994994,
44.1698858934927)) ;
#195323=CARTESIAN_POINT('Ctrl Pts',(-78.3921955146446,3.00000000005006,
44.1692968938833)) ;
#195324=CARTESIAN_POINT('Ctrl Pts',(-78.3921955146446,-4.19999999994994,
44.1692968938832)) ;
#195325=CARTESIAN_POINT('Ctrl Pts',(-78.3910188494957,3.00000000005006,
44.1687062014689)) ;
#195326=CARTESIAN_POINT('Ctrl Pts',(-78.3910188494957,-4.19999999994994,
44.1687062014688)) ;
#195327=CARTESIAN_POINT('Ctrl Pts',(-74.8968207049898,3.00000000005008,
42.4145994025118)) ;
#195328=CARTESIAN_POINT('Ctrl Pts',(-74.8968207049898,-4.19999999994992,
42.4145994025117)) ;
#195329=CARTESIAN_POINT('Ctrl Pts',(-78.6491068290692,3.00000000005016,
34.7450508231087)) ;
#195330=CARTESIAN_POINT('Ctrl Pts',(-78.6491068290692,-4.19999999994984,
34.7450508231086)) ;
#195331=CARTESIAN_POINT('',(-78.6491068290692,3.00000000005016,34.7450508231087)) ;
#195332=CARTESIAN_POINT('Origin',(-82.3091286356931,3.00000000005014,36.3637926391687)) ;
#195333=CARTESIAN_POINT('',(-78.6491068290692,-2.99999999994984,34.7450508231086)) ;
#195334=CARTESIAN_POINT('',(-78.6491068290692,3.00000000005016,34.7450508231087)) ;
#195335=CARTESIAN_POINT('Origin',(-82.3091286356924,-2.99999999994986,36.3637926391692)) ;
#195336=CARTESIAN_POINT('Origin',(-80.4791177323812,3.00000000005015,35.5544217311386)) ;
#195337=CARTESIAN_POINT('',(-82.3091286356932,3.00000000005014,36.3637926391685)) ;
#195338=CARTESIAN_POINT('',(-78.6491068290692,3.00000000005016,34.7450508231087)) ;
#195339=CARTESIAN_POINT('',(-82.3091286356932,-2.99999999994986,36.3637926391684)) ;
#195340=CARTESIAN_POINT('',(-82.3091286356932,3.00000000005014,36.3637926391685)) ;
#195341=CARTESIAN_POINT('',(-78.6491068290692,-2.99999999994984,34.7450508231086)) ;
#195342=CARTESIAN_POINT('Origin',(-82.447102343206,3.00000000005014,36.0485777519755)) ;
#195343=CARTESIAN_POINT('',(-82.585076050719,3.00000000005015,35.7333628647823)) ;
#195344=CARTESIAN_POINT('',(-82.3091286356932,3.00000000005014,36.3637926391685)) ;
#195345=CARTESIAN_POINT('',(-82.585076050719,-2.99999999994985,35.7333628647822)) ;
#195346=CARTESIAN_POINT('',(-82.585076050719,3.00000000005015,35.7333628647823)) ;
#195347=CARTESIAN_POINT('',(-82.3091286356932,-2.99999999994986,36.3637926391684)) ;
#195348=CARTESIAN_POINT('Ctrl Pts',(-82.5850760507189,3.00000000005015,
35.7333628647824)) ;
#195349=CARTESIAN_POINT('Ctrl Pts',(-82.5850760507189,-4.19999999994985,
35.7333628647823)) ;
#195350=CARTESIAN_POINT('Ctrl Pts',(-82.5838434194163,3.00000000005015,
35.7329001755683)) ;
#195351=CARTESIAN_POINT('Ctrl Pts',(-82.5838434194163,-4.19999999994985,
35.7329001755682)) ;
#195352=CARTESIAN_POINT('Ctrl Pts',(-82.5826114559916,3.00000000005015,
35.732435714029)) ;
#195353=CARTESIAN_POINT('Ctrl Pts',(-82.5826114559916,-4.19999999994985,
35.7324357140289)) ;
#195354=CARTESIAN_POINT('Ctrl Pts',(-78.9242008064233,3.00000000005016,
34.3531812580496)) ;
#195355=CARTESIAN_POINT('Ctrl Pts',(-78.9242008064233,-4.19999999994984,
34.3531812580496)) ;
#195356=CARTESIAN_POINT('Ctrl Pts',(-81.8542453875451,3.00000000005024,
26.3334265659522)) ;
#195357=CARTESIAN_POINT('Ctrl Pts',(-81.8542453875451,-4.19999999994976,
26.3334265659521)) ;
#195358=CARTESIAN_POINT('',(-81.854245387545,3.00000000005024,26.3334265659522)) ;
#195359=CARTESIAN_POINT('Origin',(-85.6634218062174,3.00000000005023,27.5607242899997)) ;
#195360=CARTESIAN_POINT('',(-81.854245387545,-2.99999999994976,26.3334265659521)) ;
#195361=CARTESIAN_POINT('',(-81.854245387545,3.00000000005024,26.3334265659522)) ;
#195362=CARTESIAN_POINT('Origin',(-85.6634218062175,-2.99999999994977,27.5607242899996)) ;
#195363=CARTESIAN_POINT('Origin',(-83.7588335968814,3.00000000005024,26.9470754279756)) ;
#195364=CARTESIAN_POINT('',(-85.6634218062177,3.00000000005023,27.5607242899993)) ;
#195365=CARTESIAN_POINT('',(-81.854245387545,3.00000000005024,26.3334265659522)) ;
#195366=CARTESIAN_POINT('',(-85.6634218062177,-2.99999999994977,27.5607242899992)) ;
#195367=CARTESIAN_POINT('',(-85.6634218062177,3.00000000005023,27.5607242899993)) ;
#195368=CARTESIAN_POINT('',(-81.854245387545,-2.99999999994976,26.3334265659521)) ;
#195369=CARTESIAN_POINT('Origin',(-85.7676907515672,3.00000000005023,27.2328140033222)) ;
#195370=CARTESIAN_POINT('',(-85.8719596969165,3.00000000005024,26.9049037166451)) ;
#195371=CARTESIAN_POINT('',(-85.6634218062177,3.00000000005023,27.5607242899993)) ;
#195372=CARTESIAN_POINT('',(-85.8719596969165,-2.99999999994976,26.904903716645)) ;
#195373=CARTESIAN_POINT('',(-85.8719596969165,3.00000000005024,26.9049037166451)) ;
#195374=CARTESIAN_POINT('',(-85.6634218062177,-2.99999999994977,27.5607242899992)) ;
#195375=CARTESIAN_POINT('Ctrl Pts',(-85.8719596969165,3.00000000005024,
26.9049037166451)) ;
#195376=CARTESIAN_POINT('Ctrl Pts',(-85.8719596969165,-4.19999999994976,
26.904903716645)) ;
#195377=CARTESIAN_POINT('Ctrl Pts',(-85.8706854539044,3.00000000005024,
26.904572407147)) ;
#195378=CARTESIAN_POINT('Ctrl Pts',(-85.8706854539044,-4.19999999994976,
26.9045724071469)) ;
#195379=CARTESIAN_POINT('Ctrl Pts',(-85.8694116898535,3.00000000005024,
26.9042392652197)) ;
#195380=CARTESIAN_POINT('Ctrl Pts',(-85.8694116898535,-4.19999999994976,
26.9042392652196)) ;
#195381=CARTESIAN_POINT('Ctrl Pts',(-82.0868708478705,3.00000000005025,
25.9149485526655)) ;
#195382=CARTESIAN_POINT('Ctrl Pts',(-82.0868708478705,-4.19999999994975,
25.9149485526654)) ;
#195383=CARTESIAN_POINT('Ctrl Pts',(-84.1625717044525,3.00000000005033,
17.6328538585215)) ;
#195384=CARTESIAN_POINT('Ctrl Pts',(-84.1625717044525,-4.19999999994967,
17.6328538585214)) ;
#195385=CARTESIAN_POINT('',(-84.1625717044525,3.00000000005033,17.6328538585214)) ;
#195386=CARTESIAN_POINT('Origin',(-88.0791686012115,3.00000000005033,18.4552609598614)) ;
#195387=CARTESIAN_POINT('',(-84.1625717044525,-2.99999999994967,17.6328538585214)) ;
#195388=CARTESIAN_POINT('',(-84.1625717044525,3.00000000005033,17.6328538585214)) ;
#195389=CARTESIAN_POINT('Origin',(-88.0791686012115,-2.99999999994968,18.4552609598614)) ;
#195390=CARTESIAN_POINT('Origin',(-86.1208701528312,3.00000000005033,18.0440574091923)) ;
#195391=CARTESIAN_POINT('',(-88.0791686012098,3.00000000005032,18.455260959863)) ;
#195392=CARTESIAN_POINT('',(-84.1625717044525,3.00000000005033,17.6328538585214)) ;
#195393=CARTESIAN_POINT('',(-88.0791686012098,-2.99999999994968,18.4552609598629)) ;
#195394=CARTESIAN_POINT('',(-88.0791686012098,3.00000000005032,18.455260959863)) ;
#195395=CARTESIAN_POINT('',(-84.1625717044525,-2.99999999994967,17.6328538585214)) ;
#195396=CARTESIAN_POINT('Origin',(-88.1485903920105,3.00000000005033,18.1182479274222)) ;
#195397=CARTESIAN_POINT('',(-88.2180121828115,3.00000000005033,17.7812348949813)) ;
#195398=CARTESIAN_POINT('',(-88.0791686012098,3.00000000005032,18.455260959863)) ;
#195399=CARTESIAN_POINT('',(-88.2180121828115,-2.99999999994967,17.7812348949812)) ;
#195400=CARTESIAN_POINT('',(-88.2180121828115,3.00000000005033,17.7812348949813)) ;
#195401=CARTESIAN_POINT('',(-88.0791686012098,-2.99999999994968,18.4552609598629)) ;
#195402=CARTESIAN_POINT('Ctrl Pts',(-88.2180121828114,3.00000000005033,
17.7812348949813)) ;
#195403=CARTESIAN_POINT('Ctrl Pts',(-88.2180121828114,-4.19999999994967,
17.7812348949812)) ;
#195404=CARTESIAN_POINT('Ctrl Pts',(-88.2167102889633,3.00000000005033,
17.7810385950953)) ;
#195405=CARTESIAN_POINT('Ctrl Pts',(-88.2167102889633,-4.19999999994967,
17.7810385950953)) ;
#195406=CARTESIAN_POINT('Ctrl Pts',(-88.2154086799115,3.00000000005033,
17.7808404227533)) ;
#195407=CARTESIAN_POINT('Ctrl Pts',(-88.2154086799115,-4.19999999994967,
17.7808404227532)) ;
#195408=CARTESIAN_POINT('Ctrl Pts',(-84.3501799545264,3.00000000005034,
17.1923523296933)) ;
#195409=CARTESIAN_POINT('Ctrl Pts',(-84.3501799545264,-4.19999999994966,
17.1923523296932)) ;
#195410=CARTESIAN_POINT('Ctrl Pts',(-85.5487952736159,3.00000000005042,
8.73865799611182)) ;
#195411=CARTESIAN_POINT('Ctrl Pts',(-85.5487952736159,-4.19999999994958,
8.73865799611175)) ;
#195412=CARTESIAN_POINT('',(-85.548795273616,3.00000000005042,8.7386579961118)) ;
#195413=CARTESIAN_POINT('Origin',(-89.5299015932563,3.00000000005042,9.1471640104453)) ;
#195414=CARTESIAN_POINT('',(-85.548795273616,-2.99999999994958,8.73865799611174)) ;
#195415=CARTESIAN_POINT('',(-85.548795273616,3.00000000005042,8.7386579961118)) ;
#195416=CARTESIAN_POINT('Origin',(-89.5299015932563,-2.99999999994958,9.14716401044516)) ;
#195417=CARTESIAN_POINT('Origin',(-87.539348433436,3.00000000005042,8.94291100327852)) ;
#195418=CARTESIAN_POINT('',(-89.5299015932563,3.00000000005042,9.14716401044524)) ;
#195419=CARTESIAN_POINT('',(-85.548795273616,3.00000000005042,8.7386579961118)) ;
#195420=CARTESIAN_POINT('',(-89.5299015932563,-2.99999999994958,9.14716401044518)) ;
#195421=CARTESIAN_POINT('',(-89.5299015932563,3.00000000005042,9.14716401044524)) ;
#195422=CARTESIAN_POINT('',(-85.548795273616,-2.99999999994958,8.73865799611174)) ;
#195423=CARTESIAN_POINT('Origin',(-89.563715629841,3.00000000005042,8.8047406175488)) ;
#195424=CARTESIAN_POINT('',(-89.5975296664259,3.00000000005043,8.46231722465223)) ;
#195425=CARTESIAN_POINT('',(-89.5299015932563,3.00000000005042,9.14716401044524)) ;
#195426=CARTESIAN_POINT('',(-89.5975296664259,-2.99999999994957,8.46231722465217)) ;
#195427=CARTESIAN_POINT('',(-89.5975296664259,3.00000000005042,8.46231722465223)) ;
#195428=CARTESIAN_POINT('',(-89.5299015932563,-2.99999999994958,9.14716401044518)) ;
#195429=CARTESIAN_POINT('Ctrl Pts',(-89.5975296664258,3.00000000005042,
8.46231722465223)) ;
#195430=CARTESIAN_POINT('Ctrl Pts',(-89.5975296664258,-4.19999999994958,
8.46231722465216)) ;
#195431=CARTESIAN_POINT('Ctrl Pts',(-89.5962143855632,3.00000000005042,
8.46225808508051)) ;
#195432=CARTESIAN_POINT('Ctrl Pts',(-89.5962143855632,-4.19999999994958,
8.46225808508044)) ;
#195433=CARTESIAN_POINT('Ctrl Pts',(-89.5948991922115,3.00000000005043,
8.4621970535414)) ;
#195434=CARTESIAN_POINT('Ctrl Pts',(-89.5948991922115,-4.19999999994958,
8.46219705354133)) ;
#195435=CARTESIAN_POINT('Ctrl Pts',(-85.6893308381907,3.00000000005043,
8.28095917867225)) ;
#195436=CARTESIAN_POINT('Ctrl Pts',(-85.6893308381907,-4.19999999994957,
8.28095917867218)) ;
#195437=CARTESIAN_POINT('Ctrl Pts',(-85.9977283395255,3.00000000005051,
-0.251714350178572)) ;
#195438=CARTESIAN_POINT('Ctrl Pts',(-85.9977283395255,-4.19999999994949,
-0.251714350178644)) ;
#195439=CARTESIAN_POINT('',(-85.9977283395255,3.00000000005051,-0.251714350178527)) ;
#195440=CARTESIAN_POINT('Origin',(-89.9997262481113,3.00000000005051,-0.261585100232212)) ;
#195441=CARTESIAN_POINT('',(-85.9977283395255,-2.99999999994949,-0.251714350178588)) ;
#195442=CARTESIAN_POINT('',(-85.9977283395255,3.00000000005051,-0.251714350178527)) ;
#195443=CARTESIAN_POINT('Origin',(-89.9997262481114,-2.99999999994948,-0.26158510023235)) ;
#195444=CARTESIAN_POINT('Origin',(-87.9987272938179,3.00000000005051,-0.256649725205155)) ;
#195445=CARTESIAN_POINT('',(-89.9997262481103,3.00000000005051,-0.261585100231687)) ;
#195446=CARTESIAN_POINT('',(-85.9977283395255,3.00000000005051,-0.251714350178527)) ;
#195447=CARTESIAN_POINT('',(-89.9997262481103,-2.99999999994949,-0.261585100231748)) ;
#195448=CARTESIAN_POINT('',(-89.9997262481103,3.00000000005051,-0.261585100231687)) ;
#195449=CARTESIAN_POINT('',(-85.9977283395255,-2.99999999994949,-0.251714350178588)) ;
#195450=CARTESIAN_POINT('Origin',(-89.9975620568182,3.00000000005052,-0.605667191234735)) ;
#195451=CARTESIAN_POINT('',(-89.9953978655262,3.00000000005052,-0.949749282237835)) ;
#195452=CARTESIAN_POINT('',(-89.9997262481103,3.00000000005051,-0.261585100231687)) ;
#195453=CARTESIAN_POINT('',(-89.9953978655262,-2.99999999994948,-0.949749282237896)) ;
#195454=CARTESIAN_POINT('',(-89.9953978655262,3.00000000005052,-0.949749282237835)) ;
#195455=CARTESIAN_POINT('',(-89.9997262481103,-2.99999999994949,-0.261585100231748)) ;
#195456=CARTESIAN_POINT('Ctrl Pts',(-89.9953978655262,3.00000000005052,
-0.949749282237899)) ;
#195457=CARTESIAN_POINT('Ctrl Pts',(-89.9953978655262,-4.19999999994948,
-0.949749282237972)) ;
#195458=CARTESIAN_POINT('Ctrl Pts',(-89.9940836081412,3.00000000005052,
-0.949670613549396)) ;
#195459=CARTESIAN_POINT('Ctrl Pts',(-89.9940836081412,-4.19999999994948,
-0.94967061354947)) ;
#195460=CARTESIAN_POINT('Ctrl Pts',(-89.9927692400234,3.00000000005052,
-0.949593835611227)) ;
#195461=CARTESIAN_POINT('Ctrl Pts',(-89.9927692400234,-4.19999999994948,
-0.9495938356113)) ;
#195462=CARTESIAN_POINT('Ctrl Pts',(-86.0896514815463,3.00000000005052,
-0.721595812205907)) ;
#195463=CARTESIAN_POINT('Ctrl Pts',(-86.0896514815463,-4.19999999994948,
-0.721595812205981)) ;
#195464=CARTESIAN_POINT('Ctrl Pts',(-85.5044522975653,3.00000000005061,
-9.23976277956772)) ;
#195465=CARTESIAN_POINT('Ctrl Pts',(-85.5044522975653,-4.1999999999494,
-9.23976277956779)) ;
#195466=CARTESIAN_POINT('',(-85.5044522975653,3.00000000005061,-9.23976277956773)) ;
#195467=CARTESIAN_POINT('Origin',(-89.4834950685368,3.00000000005062,-9.66790214800468)) ;
#195468=CARTESIAN_POINT('',(-85.5044522975653,-2.99999999994939,-9.23976277956779)) ;
#195469=CARTESIAN_POINT('',(-85.5044522975653,3.00000000005061,-9.23976277956773)) ;
#195470=CARTESIAN_POINT('Origin',(-89.4834950685368,-2.9999999999494,-9.66790214800469)) ;
#195471=CARTESIAN_POINT('Origin',(-87.493973683051,3.00000000005061,-9.4538324637858)) ;
#195472=CARTESIAN_POINT('',(-89.4834950685366,3.00000000005061,-9.66790214800376)) ;
#195473=CARTESIAN_POINT('',(-85.5044522975653,3.00000000005061,-9.23976277956773)) ;
#195474=CARTESIAN_POINT('',(-89.4834950685366,-2.99999999994939,-9.66790214800382)) ;
#195475=CARTESIAN_POINT('',(-89.4834950685366,3.00000000005061,-9.66790214800376)) ;
#195476=CARTESIAN_POINT('',(-85.5044522975653,-2.99999999994939,-9.23976277956779)) ;
#195477=CARTESIAN_POINT('Origin',(-89.4453763607008,3.00000000005061,-10.0098731017204)) ;
#195478=CARTESIAN_POINT('',(-89.4072576528647,3.00000000005062,-10.3518440554371)) ;
#195479=CARTESIAN_POINT('',(-89.4834950685366,3.00000000005061,-9.66790214800376)) ;
#195480=CARTESIAN_POINT('',(-89.4072576528647,-2.99999999994938,-10.3518440554372)) ;
#195481=CARTESIAN_POINT('',(-89.4072576528647,3.00000000005062,-10.3518440554371)) ;
#195482=CARTESIAN_POINT('',(-89.4834950685366,-2.99999999994939,-9.66790214800382)) ;
#195483=CARTESIAN_POINT('Ctrl Pts',(-89.4072576528647,3.00000000005062,
-10.3518440554371)) ;
#195484=CARTESIAN_POINT('Ctrl Pts',(-89.4072576528647,-4.19999999994939,
-10.3518440554372)) ;
#195485=CARTESIAN_POINT('Ctrl Pts',(-89.4059588182361,3.00000000005062,
-10.3516284403988)) ;
#195486=CARTESIAN_POINT('Ctrl Pts',(-89.4059588182361,-4.19999999994939,
-10.3516284403988)) ;
#195487=CARTESIAN_POINT('Ctrl Pts',(-89.404659675844,3.00000000005062,-10.351414694179)) ;
#195488=CARTESIAN_POINT('Ctrl Pts',(-89.404659675844,-4.19999999994939,
-10.3514146941791)) ;
#195489=CARTESIAN_POINT('Ctrl Pts',(-85.5467558878524,3.00000000005061,
-9.71667876655564)) ;
#195490=CARTESIAN_POINT('Ctrl Pts',(-85.5467558878524,-4.19999999994939,
-9.71667876655571)) ;
#195491=CARTESIAN_POINT('Ctrl Pts',(-84.074371583276,3.0000000000507,-18.1270123525924)) ;
#195492=CARTESIAN_POINT('Ctrl Pts',(-84.074371583276,-4.19999999994931,
-18.1270123525924)) ;
#195493=CARTESIAN_POINT('',(-84.074371583276,3.0000000000507,-18.1270123525923)) ;
#195494=CARTESIAN_POINT('Origin',(-87.9868639913669,3.0000000000507,-18.9687295548975)) ;
#195495=CARTESIAN_POINT('',(-84.074371583276,-2.9999999999493,-18.1270123525924)) ;
#195496=CARTESIAN_POINT('',(-84.074371583276,3.0000000000507,-18.1270123525923)) ;
#195497=CARTESIAN_POINT('Origin',(-87.9868639913669,-2.9999999999493,-18.9687295548977)) ;
#195498=CARTESIAN_POINT('Origin',(-86.0306177873215,3.0000000000507,-18.5478709537447)) ;
#195499=CARTESIAN_POINT('',(-87.9868639913672,3.00000000005071,-18.9687295548971)) ;
#195500=CARTESIAN_POINT('',(-84.074371583276,3.0000000000507,-18.1270123525923)) ;
#195501=CARTESIAN_POINT('',(-87.9868639913672,-2.9999999999493,-18.9687295548972)) ;
#195502=CARTESIAN_POINT('',(-87.9868639913672,3.00000000005071,-18.9687295548971)) ;
#195503=CARTESIAN_POINT('',(-84.074371583276,-2.9999999999493,-18.1270123525924)) ;
#195504=CARTESIAN_POINT('Origin',(-87.9132084035268,3.00000000005071,-19.3048426659964)) ;
#195505=CARTESIAN_POINT('',(-87.8395528156864,3.00000000005071,-19.6409557770956)) ;
#195506=CARTESIAN_POINT('',(-87.9868639913672,3.00000000005071,-18.9687295548971)) ;
#195507=CARTESIAN_POINT('',(-87.8395528156864,-2.99999999994929,-19.6409557770957)) ;
#195508=CARTESIAN_POINT('',(-87.8395528156864,3.00000000005071,-19.6409557770956)) ;
#195509=CARTESIAN_POINT('',(-87.9868639913672,-2.9999999999493,-18.9687295548972)) ;
#195510=CARTESIAN_POINT('Ctrl Pts',(-87.8395528156864,3.00000000005071,
-19.6409557770957)) ;
#195511=CARTESIAN_POINT('Ctrl Pts',(-87.8395528156864,-4.19999999994929,
-19.6409557770957)) ;
#195512=CARTESIAN_POINT('Ctrl Pts',(-87.8382836341185,3.00000000005071,
-19.6406055780315)) ;
#195513=CARTESIAN_POINT('Ctrl Pts',(-87.8382836341185,-4.19999999994929,
-19.6406055780316)) ;
#195514=CARTESIAN_POINT('Ctrl Pts',(-87.8370139511284,3.00000000005071,
-19.640257205378)) ;
#195515=CARTESIAN_POINT('Ctrl Pts',(-87.8370139511284,-4.19999999994929,
-19.6402572053781)) ;
#195516=CARTESIAN_POINT('Ctrl Pts',(-84.0665921348419,3.0000000000507,-18.6057376731866)) ;
#195517=CARTESIAN_POINT('Ctrl Pts',(-84.0665921348419,-4.1999999999493,
-18.6057376731866)) ;
#195518=CARTESIAN_POINT('Ctrl Pts',(-81.7231544602273,3.00000000005078,
-26.8160925031547)) ;
#195519=CARTESIAN_POINT('Ctrl Pts',(-81.7231544602273,-4.19999999994922,
-26.8160925031548)) ;
#195520=CARTESIAN_POINT('',(-81.7231544602271,3.00000000005079,-26.8160925031548)) ;
#195521=CARTESIAN_POINT('Origin',(-85.5262304198732,3.0000000000508,-28.0621655095208)) ;
#195522=CARTESIAN_POINT('',(-81.7231544602271,-2.99999999994922,-26.8160925031548)) ;
#195523=CARTESIAN_POINT('',(-81.7231544602271,3.00000000005079,-26.8160925031548)) ;
#195524=CARTESIAN_POINT('Origin',(-85.5262304198732,-2.99999999994921,-28.0621655095209)) ;
#195525=CARTESIAN_POINT('Origin',(-83.6246924400503,3.00000000005079,-27.4391290063367)) ;
#195526=CARTESIAN_POINT('',(-85.526230419873,3.0000000000508,-28.0621655095189)) ;
#195527=CARTESIAN_POINT('',(-81.7231544602271,3.00000000005079,-26.8160925031548)) ;
#195528=CARTESIAN_POINT('',(-85.526230419873,-2.9999999999492,-28.062165509519)) ;
#195529=CARTESIAN_POINT('',(-85.526230419873,3.0000000000508,-28.0621655095189)) ;
#195530=CARTESIAN_POINT('',(-81.7231544602271,-2.99999999994922,-26.8160925031548)) ;
#195531=CARTESIAN_POINT('Origin',(-85.4178449380624,3.0000000000508,-28.3887382524195)) ;
#195532=CARTESIAN_POINT('',(-85.3094594562516,3.0000000000508,-28.71531099532)) ;
#195533=CARTESIAN_POINT('',(-85.526230419873,3.0000000000508,-28.0621655095189)) ;
#195534=CARTESIAN_POINT('',(-85.3094594562516,-2.9999999999492,-28.7153109953201)) ;
#195535=CARTESIAN_POINT('',(-85.3094594562516,3.0000000000508,-28.71531099532)) ;
#195536=CARTESIAN_POINT('',(-85.526230419873,-2.9999999999492,-28.062165509519)) ;
#195537=CARTESIAN_POINT('Ctrl Pts',(-85.3094594562517,3.0000000000508,-28.71531099532)) ;
#195538=CARTESIAN_POINT('Ctrl Pts',(-85.3094594562517,-4.1999999999492,
-28.7153109953201)) ;
#195539=CARTESIAN_POINT('Ctrl Pts',(-85.308233833163,3.0000000000508,-28.714830049084)) ;
#195540=CARTESIAN_POINT('Ctrl Pts',(-85.308233833163,-4.1999999999492,-28.7148300490841)) ;
#195541=CARTESIAN_POINT('Ctrl Pts',(-85.3070075204872,3.0000000000508,-28.7143508668407)) ;
#195542=CARTESIAN_POINT('Ctrl Pts',(-85.3070075204872,-4.1999999999492,
-28.7143508668408)) ;
#195543=CARTESIAN_POINT('Ctrl Pts',(-81.6653772063365,3.00000000005079,
-27.2913821425628)) ;
#195544=CARTESIAN_POINT('Ctrl Pts',(-81.6653772063365,-4.19999999994921,
-27.2913821425629)) ;
#195545=CARTESIAN_POINT('Ctrl Pts',(-78.4765613552426,3.00000000005087,
-35.2118038508177)) ;
#195546=CARTESIAN_POINT('Ctrl Pts',(-78.4765613552426,-4.19999999994913,
-35.2118038508178)) ;
#195547=CARTESIAN_POINT('',(-78.4765613552426,3.00000000005087,-35.2118038508177)) ;
#195548=CARTESIAN_POINT('Origin',(-82.1285535703849,3.00000000005089,-36.8485804246292)) ;
#195549=CARTESIAN_POINT('',(-78.4765613552426,-2.99999999994913,-35.2118038508178)) ;
#195550=CARTESIAN_POINT('',(-78.4765613552426,3.00000000005087,-35.2118038508177)) ;
#195551=CARTESIAN_POINT('Origin',(-82.1285535703849,-2.99999999994912,-36.8485804246294)) ;
#195552=CARTESIAN_POINT('Origin',(-80.3025574628135,3.00000000005088,-36.0301921377219)) ;
#195553=CARTESIAN_POINT('',(-82.1285535703842,3.00000000005089,-36.8485804246263)) ;
#195554=CARTESIAN_POINT('',(-78.4765613552426,3.00000000005087,-35.2118038508177)) ;
#195555=CARTESIAN_POINT('',(-82.1285535703842,-2.99999999994911,-36.8485804246263)) ;
#195556=CARTESIAN_POINT('',(-82.1285535703842,3.00000000005089,-36.8485804246263)) ;
#195557=CARTESIAN_POINT('',(-78.4765613552426,-2.99999999994913,-35.2118038508178)) ;
#195558=CARTESIAN_POINT('Origin',(-81.9866256886229,3.00000000005089,-37.1620348000171)) ;
#195559=CARTESIAN_POINT('',(-81.8446978068616,3.00000000005089,-37.4754891754079)) ;
#195560=CARTESIAN_POINT('',(-82.1285535703842,3.00000000005089,-36.8485804246263)) ;
#195561=CARTESIAN_POINT('',(-81.8446978068616,-2.99999999994911,-37.475489175408)) ;
#195562=CARTESIAN_POINT('',(-81.8446978068616,3.00000000005089,-37.4754891754079)) ;
#195563=CARTESIAN_POINT('',(-82.1285535703842,-2.99999999994911,-36.8485804246264)) ;
#195564=CARTESIAN_POINT('Ctrl Pts',(-81.8446978068617,3.00000000005089,
-37.4754891754079)) ;
#195565=CARTESIAN_POINT('Ctrl Pts',(-81.8446978068617,-4.19999999994911,
-37.475489175408)) ;
#195566=CARTESIAN_POINT('Ctrl Pts',(-81.8435291704357,3.00000000005089,
-37.4748827513478)) ;
#195567=CARTESIAN_POINT('Ctrl Pts',(-81.8435291704357,-4.19999999994911,
-37.4748827513479)) ;
#195568=CARTESIAN_POINT('Ctrl Pts',(-81.8423596638125,3.00000000005089,
-37.4742780095355)) ;
#195569=CARTESIAN_POINT('Ctrl Pts',(-81.8423596638125,-4.19999999994911,
-37.4742780095356)) ;
#195570=CARTESIAN_POINT('Ctrl Pts',(-78.3694193155794,3.00000000005088,
-35.6784504362897)) ;
#195571=CARTESIAN_POINT('Ctrl Pts',(-78.3694193155794,-4.19999999994913,
-35.6784504362897)) ;
#195572=CARTESIAN_POINT('Ctrl Pts',(-74.3701626217736,3.00000000005095,
-43.2221612251409)) ;
#195573=CARTESIAN_POINT('Ctrl Pts',(-74.3701626217736,-4.19999999994906,
-43.222161225141)) ;
#195574=CARTESIAN_POINT('',(-74.3701626217736,3.00000000005095,-43.2221612251409)) ;
#195575=CARTESIAN_POINT('Origin',(-77.831059101474,3.00000000005098,-45.231708499739)) ;
#195576=CARTESIAN_POINT('',(-74.3701626217736,-2.99999999994905,-43.222161225141)) ;
#195577=CARTESIAN_POINT('',(-74.3701626217736,3.00000000005095,-43.2221612251409)) ;
#195578=CARTESIAN_POINT('Origin',(-77.8310591014741,-2.99999999994903,-45.2317084997386)) ;
#195579=CARTESIAN_POINT('Origin',(-76.1006108616236,3.00000000005096,-44.2269348624374)) ;
#195580=CARTESIAN_POINT('',(-77.831059101474,3.00000000005097,-45.2317084997338)) ;
#195581=CARTESIAN_POINT('',(-74.3701626217736,3.00000000005095,-43.2221612251409)) ;
#195582=CARTESIAN_POINT('',(-77.831059101474,-2.99999999994903,-45.2317084997339)) ;
#195583=CARTESIAN_POINT('',(-77.831059101474,3.00000000005097,-45.2317084997338)) ;
#195584=CARTESIAN_POINT('',(-74.3701626217736,-2.99999999994905,-43.222161225141)) ;
#195585=CARTESIAN_POINT('Origin',(-77.657143811335,3.00000000005098,-45.5286102358837)) ;
#195586=CARTESIAN_POINT('',(-77.4832285211961,3.00000000005098,-45.8255119720335)) ;
#195587=CARTESIAN_POINT('',(-77.831059101474,3.00000000005097,-45.2317084997338)) ;
#195588=CARTESIAN_POINT('',(-77.4832285211961,-2.99999999994902,-45.8255119720336)) ;
#195589=CARTESIAN_POINT('',(-77.4832285211961,3.00000000005098,-45.8255119720335)) ;
#195590=CARTESIAN_POINT('',(-77.831059101474,-2.99999999994903,-45.2317084997339)) ;
#195591=CARTESIAN_POINT('Ctrl Pts',(-77.4832285211961,3.00000000005098,
-45.8255119720335)) ;
#195592=CARTESIAN_POINT('Ctrl Pts',(-77.4832285211961,-4.19999999994902,
-45.8255119720336)) ;
#195593=CARTESIAN_POINT('Ctrl Pts',(-77.4821296752578,3.00000000005098,
-45.8247867142581)) ;
#195594=CARTESIAN_POINT('Ctrl Pts',(-77.4821296752578,-4.19999999994902,
-45.8247867142582)) ;
#195595=CARTESIAN_POINT('Ctrl Pts',(-77.4810297880467,3.00000000005098,
-45.8240630385544)) ;
#195596=CARTESIAN_POINT('Ctrl Pts',(-77.4810297880467,-4.19999999994902,
-45.8240630385545)) ;
#195597=CARTESIAN_POINT('Ctrl Pts',(-74.2148296669459,3.00000000005096,
-43.6750520790345)) ;
#195598=CARTESIAN_POINT('Ctrl Pts',(-74.2148296669459,-4.19999999994905,
-43.6750520790346)) ;
#195599=CARTESIAN_POINT('Ctrl Pts',(-69.4489488236634,3.00000000005103,
-50.7594014744564)) ;
#195600=CARTESIAN_POINT('Ctrl Pts',(-69.4489488236634,-4.19999999994897,
-50.7594014744564)) ;
#195601=CARTESIAN_POINT('',(-69.4489488236635,3.00000000005103,-50.7594014744564)) ;
#195602=CARTESIAN_POINT('Origin',(-72.6808312618518,3.00000000005105,-53.1197024293663)) ;
#195603=CARTESIAN_POINT('',(-69.4489488236635,-2.99999999994897,-50.7594014744565)) ;
#195604=CARTESIAN_POINT('',(-69.4489488236635,3.00000000005103,-50.7594014744564)) ;
#195605=CARTESIAN_POINT('Origin',(-72.6808312618517,-2.99999999994895,-53.1197024293665)) ;
#195606=CARTESIAN_POINT('Origin',(-71.0648900427576,3.00000000005104,-51.9395519519123)) ;
#195607=CARTESIAN_POINT('',(-72.6808312618515,3.00000000005105,-53.1197024293682)) ;
#195608=CARTESIAN_POINT('',(-69.4489488236635,3.00000000005103,-50.7594014744564)) ;
#195609=CARTESIAN_POINT('',(-72.6808312618515,-2.99999999994895,-53.1197024293683)) ;
#195610=CARTESIAN_POINT('',(-72.6808312618515,3.00000000005105,-53.1197024293682)) ;
#195611=CARTESIAN_POINT('',(-69.4489488236635,-2.99999999994897,-50.7594014744565)) ;
#195612=CARTESIAN_POINT('Origin',(-72.4768340156477,3.00000000005106,-53.3967986087252)) ;
#195613=CARTESIAN_POINT('',(-72.2728367694438,3.00000000005106,-53.6738947880823)) ;
#195614=CARTESIAN_POINT('',(-72.6808312618515,3.00000000005105,-53.1197024293682)) ;
#195615=CARTESIAN_POINT('',(-72.2728367694438,-2.99999999994894,-53.6738947880823)) ;
#195616=CARTESIAN_POINT('',(-72.2728367694438,3.00000000005106,-53.6738947880822)) ;
#195617=CARTESIAN_POINT('',(-72.6808312618515,-2.99999999994895,-53.1197024293683)) ;
#195618=CARTESIAN_POINT('Ctrl Pts',(-72.2728367694438,3.00000000005106,
-53.6738947880822)) ;
#195619=CARTESIAN_POINT('Ctrl Pts',(-72.2728367694438,-4.19999999994894,
-53.6738947880823)) ;
#195620=CARTESIAN_POINT('Ctrl Pts',(-72.2718197531795,3.00000000005106,
-53.6730586426677)) ;
#195621=CARTESIAN_POINT('Ctrl Pts',(-72.2718197531795,-4.19999999994894,
-53.6730586426678)) ;
#195622=CARTESIAN_POINT('Ctrl Pts',(-72.2708015359745,3.00000000005106,
-53.6722239618152)) ;
#195623=CARTESIAN_POINT('Ctrl Pts',(-72.2708015359745,-4.19999999994894,
-53.6722239618153)) ;
#195624=CARTESIAN_POINT('Ctrl Pts',(-69.2471268140292,3.00000000005103,
-51.1935746298029)) ;
#195625=CARTESIAN_POINT('Ctrl Pts',(-69.2471268140292,-4.19999999994897,
-51.1935746298029)) ;
#195626=CARTESIAN_POINT('Ctrl Pts',(-63.7668378091141,3.0000000000511,-57.7409450173242)) ;
#195627=CARTESIAN_POINT('Ctrl Pts',(-63.7668378091141,-4.1999999999489,
-57.7409450173243)) ;
#195628=CARTESIAN_POINT('',(-63.7668378091141,3.0000000000511,-57.7409450173242)) ;
#195629=CARTESIAN_POINT('Origin',(-66.7342970254822,3.00000000005113,-60.4261397013694)) ;
#195630=CARTESIAN_POINT('',(-63.7668378091141,-2.9999999999489,-57.7409450173243)) ;
#195631=CARTESIAN_POINT('',(-63.7668378091141,3.0000000000511,-57.7409450173242)) ;
#195632=CARTESIAN_POINT('Origin',(-66.7342970254822,-2.99999999994887,-60.4261397013694)) ;
#195633=CARTESIAN_POINT('Origin',(-65.2505674172983,3.00000000005111,-59.0835423593459)) ;
#195634=CARTESIAN_POINT('',(-66.7342970254824,3.00000000005113,-60.4261397013678)) ;
#195635=CARTESIAN_POINT('',(-63.7668378091141,3.0000000000511,-57.7409450173242)) ;
#195636=CARTESIAN_POINT('',(-66.7342970254824,-2.99999999994887,-60.4261397013679)) ;
#195637=CARTESIAN_POINT('',(-66.7342970254824,3.00000000005113,-60.4261397013678)) ;
#195638=CARTESIAN_POINT('',(-63.7668378091141,-2.9999999999489,-57.7409450173243)) ;
#195639=CARTESIAN_POINT('Origin',(-66.5024528597323,3.00000000005113,-60.6803944002046)) ;
#195640=CARTESIAN_POINT('',(-66.2706086939824,3.00000000005113,-60.9346490990415)) ;
#195641=CARTESIAN_POINT('',(-66.7342970254824,3.00000000005113,-60.4261397013678)) ;
#195642=CARTESIAN_POINT('',(-66.2706086939824,-2.99999999994887,-60.9346490990415)) ;
#195643=CARTESIAN_POINT('',(-66.2706086939824,3.00000000005113,-60.9346490990415)) ;
#195644=CARTESIAN_POINT('',(-66.7342970254824,-2.99999999994887,-60.4261397013679)) ;
#195645=CARTESIAN_POINT('Ctrl Pts',(-66.2706086939822,3.00000000005113,
-60.9346490990415)) ;
#195646=CARTESIAN_POINT('Ctrl Pts',(-66.2706086939822,-4.19999999994887,
-60.9346490990416)) ;
#195647=CARTESIAN_POINT('Ctrl Pts',(-66.2696846500344,3.00000000005113,
-60.9337112269716)) ;
#195648=CARTESIAN_POINT('Ctrl Pts',(-66.2696846500344,-4.19999999994888,
-60.9337112269717)) ;
#195649=CARTESIAN_POINT('Ctrl Pts',(-66.268759258637,3.00000000005113,-60.9327746859086)) ;
#195650=CARTESIAN_POINT('Ctrl Pts',(-66.268759258637,-4.19999999994888,
-60.9327746859087)) ;
#195651=CARTESIAN_POINT('Ctrl Pts',(-63.5207379488454,3.0000000000511,-58.1516435821762)) ;
#195652=CARTESIAN_POINT('Ctrl Pts',(-63.5207379488454,-4.1999999999489,
-58.1516435821762)) ;
#195653=CARTESIAN_POINT('Ctrl Pts',(-57.3860839754599,3.00000000005116,
-64.0903006017057)) ;
#195654=CARTESIAN_POINT('Ctrl Pts',(-57.3860839754599,-4.19999999994884,
-64.0903006017058)) ;
#195655=CARTESIAN_POINT('',(-57.3860839754598,3.00000000005116,-64.0903006017057)) ;
#195656=CARTESIAN_POINT('Origin',(-60.0566078658523,3.0000000000512,-67.0709694600124)) ;
#195657=CARTESIAN_POINT('',(-57.3860839754598,-2.99999999994884,-64.0903006017058)) ;
#195658=CARTESIAN_POINT('',(-57.3860839754598,3.00000000005116,-64.0903006017057)) ;
#195659=CARTESIAN_POINT('Origin',(-60.0566078658524,-2.9999999999488,-67.0709694600122)) ;
#195660=CARTESIAN_POINT('Origin',(-58.7213459206564,3.00000000005118,-65.5806350308578)) ;
#195661=CARTESIAN_POINT('',(-60.0566078658526,3.00000000005119,-67.0709694600098)) ;
#195662=CARTESIAN_POINT('',(-57.3860839754598,3.00000000005116,-64.0903006017057)) ;
#195663=CARTESIAN_POINT('',(-60.0566078658526,-2.99999999994881,-67.0709694600099)) ;
#195664=CARTESIAN_POINT('',(-60.0566078658526,3.00000000005119,-67.0709694600098)) ;
#195665=CARTESIAN_POINT('',(-57.3860839754598,-2.99999999994884,-64.0903006017058)) ;
#195666=CARTESIAN_POINT('Origin',(-59.799456913753,3.0000000000512,-67.2995970106399)) ;
#195667=CARTESIAN_POINT('',(-59.5423059616533,3.0000000000512,-67.52822456127)) ;
#195668=CARTESIAN_POINT('',(-60.0566078658526,3.00000000005119,-67.0709694600098)) ;
#195669=CARTESIAN_POINT('',(-59.5423059616533,-2.9999999999488,-67.5282245612701)) ;
#195670=CARTESIAN_POINT('',(-59.5423059616533,3.0000000000512,-67.52822456127)) ;
#195671=CARTESIAN_POINT('',(-60.0566078658526,-2.99999999994881,-67.0709694600099)) ;
#195672=CARTESIAN_POINT('Ctrl Pts',(-59.5423059616532,3.0000000000512,-67.52822456127)) ;
#195673=CARTESIAN_POINT('Ctrl Pts',(-59.5423059616532,-4.19999999994881,
-67.5282245612701)) ;
#195674=CARTESIAN_POINT('Ctrl Pts',(-59.5414850140409,3.0000000000512,-67.5271952380677)) ;
#195675=CARTESIAN_POINT('Ctrl Pts',(-59.5414850140409,-4.19999999994881,
-67.5271952380678)) ;
#195676=CARTESIAN_POINT('Ctrl Pts',(-59.5406625872325,3.0000000000512,-67.5261670977339)) ;
#195677=CARTESIAN_POINT('Ctrl Pts',(-59.5406625872325,-4.19999999994881,
-67.526167097734)) ;
#195678=CARTESIAN_POINT('Ctrl Pts',(-57.0984025861253,3.00000000005117,
-64.4730248766433)) ;
#195679=CARTESIAN_POINT('Ctrl Pts',(-57.0984025861253,-4.19999999994884,
-64.4730248766434)) ;
#195680=CARTESIAN_POINT('Ctrl Pts',(-50.3765961969604,3.00000000005122,
-69.7379033591308)) ;
#195681=CARTESIAN_POINT('Ctrl Pts',(-50.3765961969604,-4.19999999994878,
-69.7379033591309)) ;
#195682=CARTESIAN_POINT('',(-50.3765961969605,3.00000000005122,-69.7379033591309)) ;
#195683=CARTESIAN_POINT('Origin',(-52.7209259427919,3.00000000005125,-72.9813895599401)) ;
#195684=CARTESIAN_POINT('',(-50.3765961969605,-2.99999999994878,-69.7379033591309)) ;
#195685=CARTESIAN_POINT('',(-50.3765961969605,3.00000000005122,-69.7379033591309)) ;
#195686=CARTESIAN_POINT('Origin',(-52.7209259427916,-2.99999999994874,-72.9813895599407)) ;
#195687=CARTESIAN_POINT('Origin',(-51.5487610698761,3.00000000005124,-71.3596464595349)) ;
#195688=CARTESIAN_POINT('',(-52.720925942792,3.00000000005125,-72.9813895599391)) ;
#195689=CARTESIAN_POINT('',(-50.3765961969605,3.00000000005122,-69.7379033591309)) ;
#195690=CARTESIAN_POINT('',(-52.720925942792,-2.99999999994875,-72.9813895599392)) ;
#195691=CARTESIAN_POINT('',(-52.7209259427919,3.00000000005125,-72.9813895599391)) ;
#195692=CARTESIAN_POINT('',(-50.3765961969605,-2.99999999994878,-69.7379033591309)) ;
#195693=CARTESIAN_POINT('Origin',(-52.4412856039857,3.00000000005126,-73.1818850710742)) ;
#195694=CARTESIAN_POINT('',(-52.1616452651797,3.00000000005126,-73.3823805822094)) ;
#195695=CARTESIAN_POINT('',(-52.7209259427919,3.00000000005125,-72.9813895599391)) ;
#195696=CARTESIAN_POINT('',(-52.1616452651797,-2.99999999994874,-73.3823805822095)) ;
#195697=CARTESIAN_POINT('',(-52.1616452651797,3.00000000005126,-73.3823805822094)) ;
#195698=CARTESIAN_POINT('',(-52.7209259427919,-2.99999999994874,-72.9813895599392)) ;
#195699=CARTESIAN_POINT('Ctrl Pts',(-52.1616452651797,3.00000000005126,
-73.3823805822094)) ;
#195700=CARTESIAN_POINT('Ctrl Pts',(-52.1616452651797,-4.19999999994875,
-73.3823805822095)) ;
#195701=CARTESIAN_POINT('Ctrl Pts',(-52.1609364083768,3.00000000005126,
-73.3812710853549)) ;
#195702=CARTESIAN_POINT('Ctrl Pts',(-52.1609364083768,-4.19999999994875,
-73.3812710853549)) ;
#195703=CARTESIAN_POINT('Ctrl Pts',(-52.1602259568379,3.00000000005126,
-73.3801626102712)) ;
#195704=CARTESIAN_POINT('Ctrl Pts',(-52.1602259568379,-4.19999999994875,
-73.3801626102713)) ;
#195705=CARTESIAN_POINT('Ctrl Pts',(-50.0504851760628,3.00000000005122,
-70.0884601369073)) ;
#195706=CARTESIAN_POINT('Ctrl Pts',(-50.0504851760628,-4.19999999994878,
-70.0884601369073)) ;
#195707=CARTESIAN_POINT('Ctrl Pts',(-42.8151718885463,3.00000000005127,
-74.6218769719522)) ;
#195708=CARTESIAN_POINT('Ctrl Pts',(-42.8151718885463,-4.19999999994874,
-74.6218769719522)) ;
#195709=CARTESIAN_POINT('',(-42.8151718885463,3.00000000005127,-74.6218769719522)) ;
#195710=CARTESIAN_POINT('Origin',(-44.8076225225372,3.00000000005131,-78.0926442017079)) ;
#195711=CARTESIAN_POINT('',(-42.8151718885463,-2.99999999994873,-74.6218769719522)) ;
#195712=CARTESIAN_POINT('',(-42.8151718885463,3.00000000005127,-74.6218769719522)) ;
#195713=CARTESIAN_POINT('Origin',(-44.8076225225367,-2.99999999994869,-78.0926442017088)) ;
#195714=CARTESIAN_POINT('Origin',(-43.8113972055423,3.00000000005129,-76.3572605868288)) ;
#195715=CARTESIAN_POINT('',(-44.8076225225385,3.00000000005131,-78.0926442017055)) ;
#195716=CARTESIAN_POINT('',(-42.8151718885463,3.00000000005127,-74.6218769719522)) ;
#195717=CARTESIAN_POINT('',(-44.8076225225385,-2.99999999994869,-78.0926442017056)) ;
#195718=CARTESIAN_POINT('',(-44.8076225225385,3.00000000005131,-78.0926442017055)) ;
#195719=CARTESIAN_POINT('',(-42.8151718885463,-2.99999999994873,-74.6218769719522)) ;
#195720=CARTESIAN_POINT('Origin',(-44.5085565950966,3.00000000005131,-78.2628110025695)) ;
#195721=CARTESIAN_POINT('',(-44.2094906676548,3.00000000005131,-78.4329778034335)) ;
#195722=CARTESIAN_POINT('',(-44.8076225225385,3.00000000005131,-78.0926442017055)) ;
#195723=CARTESIAN_POINT('',(-44.2094906676548,-2.99999999994869,-78.4329778034335)) ;
#195724=CARTESIAN_POINT('',(-44.2094906676548,3.00000000005131,-78.4329778034335)) ;
#195725=CARTESIAN_POINT('',(-44.8076225225385,-2.99999999994869,-78.0926442017056)) ;
#195726=CARTESIAN_POINT('Ctrl Pts',(-44.2094906676548,3.00000000005131,
-78.4329778034335)) ;
#195727=CARTESIAN_POINT('Ctrl Pts',(-44.2094906676548,-4.1999999999487,
-78.4329778034335)) ;
#195728=CARTESIAN_POINT('Ctrl Pts',(-44.2089016680447,3.00000000005131,
-78.4318002888068)) ;
#195729=CARTESIAN_POINT('Ctrl Pts',(-44.2089016680447,-4.19999999994869,
-78.4318002888068)) ;
#195730=CARTESIAN_POINT('Ctrl Pts',(-44.2083109756307,3.00000000005131,
-78.4306236236576)) ;
#195731=CARTESIAN_POINT('Ctrl Pts',(-44.2083109756307,-4.19999999994869,
-78.4306236236577)) ;
#195732=CARTESIAN_POINT('Ctrl Pts',(-42.4542041766736,3.00000000005127,
-74.936425479152)) ;
#195733=CARTESIAN_POINT('Ctrl Pts',(-42.4542041766736,-4.19999999994873,
-74.9364254791521)) ;
#195734=CARTESIAN_POINT('Ctrl Pts',(-34.7846555972706,3.00000000005131,
-78.6887116032311)) ;
#195735=CARTESIAN_POINT('Ctrl Pts',(-34.7846555972706,-4.19999999994869,
-78.6887116032311)) ;
#195736=CARTESIAN_POINT('',(-34.7846555972706,3.00000000005131,-78.688711603231)) ;
#195737=CARTESIAN_POINT('Origin',(-36.4033974133306,3.00000000005135,-82.3487334098553)) ;
#195738=CARTESIAN_POINT('',(-34.7846555972706,-2.99999999994869,-78.688711603231)) ;
#195739=CARTESIAN_POINT('',(-34.7846555972706,3.00000000005131,-78.688711603231)) ;
#195740=CARTESIAN_POINT('Origin',(-36.4033974133303,-2.99999999994865,-82.3487334098556)) ;
#195741=CARTESIAN_POINT('Origin',(-35.5940265053004,3.00000000005133,-80.5187225065432)) ;
#195742=CARTESIAN_POINT('',(-36.4033974133301,3.00000000005135,-82.3487334098552)) ;
#195743=CARTESIAN_POINT('',(-34.7846555972706,3.00000000005131,-78.688711603231)) ;
#195744=CARTESIAN_POINT('',(-36.4033974133301,-2.99999999994865,-82.3487334098553)) ;
#195745=CARTESIAN_POINT('',(-36.4033974133301,3.00000000005135,-82.3487334098552)) ;
#195746=CARTESIAN_POINT('',(-34.7846555972706,-2.99999999994869,-78.688711603231)) ;
#195747=CARTESIAN_POINT('Origin',(-36.0881825261373,3.00000000005135,-82.486707117368)) ;
#195748=CARTESIAN_POINT('',(-35.7729676389441,3.00000000005135,-82.6246808248807)) ;
#195749=CARTESIAN_POINT('',(-36.4033974133301,3.00000000005135,-82.3487334098552)) ;
#195750=CARTESIAN_POINT('',(-35.7729676389441,-2.99999999994865,-82.6246808248808)) ;
#195751=CARTESIAN_POINT('',(-35.7729676389441,3.00000000005135,-82.6246808248807)) ;
#195752=CARTESIAN_POINT('',(-36.4033974133301,-2.99999999994865,-82.3487334098553)) ;
#195753=CARTESIAN_POINT('Ctrl Pts',(-35.7729676389442,3.00000000005135,
-82.6246808248807)) ;
#195754=CARTESIAN_POINT('Ctrl Pts',(-35.7729676389442,-4.19999999994865,
-82.6246808248808)) ;
#195755=CARTESIAN_POINT('Ctrl Pts',(-35.7725049497304,3.00000000005135,
-82.623448193578)) ;
#195756=CARTESIAN_POINT('Ctrl Pts',(-35.7725049497304,-4.19999999994865,
-82.6234481935781)) ;
#195757=CARTESIAN_POINT('Ctrl Pts',(-35.7720404881909,3.00000000005135,
-82.6222162301533)) ;
#195758=CARTESIAN_POINT('Ctrl Pts',(-35.7720404881909,-4.19999999994865,
-82.6222162301534)) ;
#195759=CARTESIAN_POINT('Ctrl Pts',(-34.3927860322115,3.00000000005132,
-78.9638055805851)) ;
#195760=CARTESIAN_POINT('Ctrl Pts',(-34.3927860322115,-4.19999999994869,
-78.9638055805852)) ;
#195761=CARTESIAN_POINT('Ctrl Pts',(-26.3730313401139,3.00000000005135,
-81.8938501617067)) ;
#195762=CARTESIAN_POINT('Ctrl Pts',(-26.3730313401139,-4.19999999994866,
-81.8938501617068)) ;
#195763=CARTESIAN_POINT('',(-26.3730313401137,3.00000000005134,-81.8938501617067)) ;
#195764=CARTESIAN_POINT('Origin',(-27.6003290641614,3.00000000005139,-85.7030265803784)) ;
#195765=CARTESIAN_POINT('',(-26.3730313401137,-2.99999999994865,-81.8938501617068)) ;
#195766=CARTESIAN_POINT('',(-26.3730313401137,3.00000000005135,-81.8938501617067)) ;
#195767=CARTESIAN_POINT('Origin',(-27.6003290641614,-2.99999999994862,-85.7030265803784)) ;
#195768=CARTESIAN_POINT('Origin',(-26.9866802021376,3.00000000005137,-83.798438371043)) ;
#195769=CARTESIAN_POINT('',(-27.6003290641611,3.00000000005138,-85.7030265803795)) ;
#195770=CARTESIAN_POINT('',(-26.3730313401137,3.00000000005135,-81.8938501617067)) ;
#195771=CARTESIAN_POINT('',(-27.6003290641611,-2.99999999994862,-85.7030265803796)) ;
#195772=CARTESIAN_POINT('',(-27.6003290641611,3.00000000005138,-85.7030265803795)) ;
#195773=CARTESIAN_POINT('',(-26.3730313401137,-2.99999999994865,-81.8938501617068)) ;
#195774=CARTESIAN_POINT('Origin',(-27.272418777484,3.00000000005138,-85.8072955257288)) ;
#195775=CARTESIAN_POINT('',(-26.9445084908068,3.00000000005139,-85.9115644710781)) ;
#195776=CARTESIAN_POINT('',(-27.6003290641611,3.00000000005138,-85.7030265803795)) ;
#195777=CARTESIAN_POINT('',(-26.9445084908068,-2.99999999994861,-85.9115644710782)) ;
#195778=CARTESIAN_POINT('',(-26.9445084908068,3.00000000005139,-85.9115644710781)) ;
#195779=CARTESIAN_POINT('',(-27.6003290641611,-2.99999999994862,-85.7030265803796)) ;
#195780=CARTESIAN_POINT('Ctrl Pts',(-26.9445084908069,3.00000000005139,
-85.9115644710781)) ;
#195781=CARTESIAN_POINT('Ctrl Pts',(-26.9445084908069,-4.19999999994862,
-85.9115644710782)) ;
#195782=CARTESIAN_POINT('Ctrl Pts',(-26.9441771813088,3.00000000005139,
-85.9102902280661)) ;
#195783=CARTESIAN_POINT('Ctrl Pts',(-26.9441771813088,-4.19999999994862,
-85.9102902280662)) ;
#195784=CARTESIAN_POINT('Ctrl Pts',(-26.9438440393815,3.00000000005139,
-85.9090164640151)) ;
#195785=CARTESIAN_POINT('Ctrl Pts',(-26.9438440393815,-4.19999999994862,
-85.9090164640151)) ;
#195786=CARTESIAN_POINT('Ctrl Pts',(-25.9545533268275,3.00000000005135,
-82.1264756220326)) ;
#195787=CARTESIAN_POINT('Ctrl Pts',(-25.9545533268275,-4.19999999994866,
-82.1264756220326)) ;
#195788=CARTESIAN_POINT('Ctrl Pts',(-17.6724586326836,3.00000000005137,
-84.2021764786145)) ;
#195789=CARTESIAN_POINT('Ctrl Pts',(-17.6724586326836,-4.19999999994864,
-84.2021764786145)) ;
#195790=CARTESIAN_POINT('',(-17.6724586326835,3.00000000005137,-84.2021764786144)) ;
#195791=CARTESIAN_POINT('Origin',(-18.4948657340208,3.00000000005141,-88.1187733753747)) ;
#195792=CARTESIAN_POINT('',(-17.6724586326835,-2.99999999994863,-84.2021764786145)) ;
#195793=CARTESIAN_POINT('',(-17.6724586326835,3.00000000005137,-84.2021764786144)) ;
#195794=CARTESIAN_POINT('Origin',(-18.4948657340221,-2.99999999994859,-88.1187733753737)) ;
#195795=CARTESIAN_POINT('Origin',(-18.0836621833542,3.00000000005139,-86.1604749269931)) ;
#195796=CARTESIAN_POINT('',(-18.4948657340249,3.00000000005141,-88.1187733753717)) ;
#195797=CARTESIAN_POINT('',(-17.6724586326835,3.00000000005137,-84.2021764786144)) ;
#195798=CARTESIAN_POINT('',(-18.4948657340249,-2.99999999994859,-88.1187733753718)) ;
#195799=CARTESIAN_POINT('',(-18.4948657340249,3.00000000005141,-88.1187733753717)) ;
#195800=CARTESIAN_POINT('',(-17.6724586326835,-2.99999999994863,-84.2021764786145)) ;
#195801=CARTESIAN_POINT('Origin',(-18.157852701584,3.00000000005141,-88.1881951661725)) ;
#195802=CARTESIAN_POINT('',(-17.820839669143,3.00000000005141,-88.2576169569733)) ;
#195803=CARTESIAN_POINT('',(-18.4948657340249,3.00000000005141,-88.1187733753717)) ;
#195804=CARTESIAN_POINT('',(-17.820839669143,-2.99999999994859,-88.2576169569734)) ;
#195805=CARTESIAN_POINT('',(-17.820839669143,3.00000000005141,-88.2576169569733)) ;
#195806=CARTESIAN_POINT('',(-18.4948657340249,-2.99999999994859,-88.1187733753718)) ;
#195807=CARTESIAN_POINT('Ctrl Pts',(-17.8208396691431,3.00000000005141,
-88.2576169569734)) ;
#195808=CARTESIAN_POINT('Ctrl Pts',(-17.8208396691431,-4.19999999994862,
-88.2576169569734)) ;
#195809=CARTESIAN_POINT('Ctrl Pts',(-17.8206433692572,3.00000000005141,
-88.2563150631251)) ;
#195810=CARTESIAN_POINT('Ctrl Pts',(-17.8206433692572,-4.19999999994862,
-88.2563150631251)) ;
#195811=CARTESIAN_POINT('Ctrl Pts',(-17.820445196915,3.00000000005141,-88.2550134540732)) ;
#195812=CARTESIAN_POINT('Ctrl Pts',(-17.820445196915,-4.19999999994862,
-88.2550134540732)) ;
#195813=CARTESIAN_POINT('Ctrl Pts',(-17.2319571038551,3.00000000005137,
-84.3897847286881)) ;
#195814=CARTESIAN_POINT('Ctrl Pts',(-17.2319571038551,-4.19999999994866,
-84.3897847286881)) ;
#195815=CARTESIAN_POINT('Ctrl Pts',(-8.77826277027359,3.00000000005138,
-85.588400047778)) ;
#195816=CARTESIAN_POINT('Ctrl Pts',(-8.77826277027359,-4.19999999994865,
-85.588400047778)) ;
#195817=CARTESIAN_POINT('',(-8.77826277027339,3.00000000005138,-85.5884000477779)) ;
#195818=CARTESIAN_POINT('Origin',(-9.18676878460829,3.00000000005142,-89.5695063674171)) ;
#195819=CARTESIAN_POINT('',(-8.77826277027339,-2.99999999994862,-85.5884000477779)) ;
#195820=CARTESIAN_POINT('',(-8.77826277027339,3.00000000005138,-85.5884000477779)) ;
#195821=CARTESIAN_POINT('Origin',(-9.18676878460891,-2.99999999994858,-89.5695063674169)) ;
#195822=CARTESIAN_POINT('Origin',(-8.98251577744032,3.0000000000514,-87.578953207598)) ;
#195823=CARTESIAN_POINT('',(-9.18676878460678,3.00000000005142,-89.5695063674181)) ;
#195824=CARTESIAN_POINT('',(-8.77826277027339,3.00000000005138,-85.5884000477779)) ;
#195825=CARTESIAN_POINT('',(-9.18676878460678,-2.99999999994858,-89.5695063674181)) ;
#195826=CARTESIAN_POINT('',(-9.18676878460679,3.00000000005143,-89.5695063674181)) ;
#195827=CARTESIAN_POINT('',(-8.77826277027339,-2.99999999994862,-85.5884000477779)) ;
#195828=CARTESIAN_POINT('Origin',(-8.84434539171035,3.00000000005142,-89.603320404003)) ;
#195829=CARTESIAN_POINT('',(-8.50192199881371,3.00000000005142,-89.6371344405877)) ;
#195830=CARTESIAN_POINT('',(-9.18676878460679,3.00000000005143,-89.5695063674181)) ;
#195831=CARTESIAN_POINT('',(-8.50192199881371,-2.99999999994858,-89.6371344405878)) ;
#195832=CARTESIAN_POINT('',(-8.50192199881372,3.00000000005143,-89.6371344405877)) ;
#195833=CARTESIAN_POINT('',(-9.18676878460679,-2.99999999994858,-89.5695063674182)) ;
#195834=CARTESIAN_POINT('Ctrl Pts',(-8.50192199881377,3.00000000005142,
-89.6371344405878)) ;
#195835=CARTESIAN_POINT('Ctrl Pts',(-8.50192199881377,-4.19999999994858,
-89.6371344405879)) ;
#195836=CARTESIAN_POINT('Ctrl Pts',(-8.50186285924238,3.00000000005143,
-89.635819159725)) ;
#195837=CARTESIAN_POINT('Ctrl Pts',(-8.50186285924238,-4.19999999994858,
-89.6358191597251)) ;
#195838=CARTESIAN_POINT('Ctrl Pts',(-8.50180182770284,3.00000000005142,
-89.6345039663731)) ;
#195839=CARTESIAN_POINT('Ctrl Pts',(-8.50180182770284,-4.19999999994858,
-89.6345039663732)) ;
#195840=CARTESIAN_POINT('Ctrl Pts',(-8.32056395283379,3.00000000005138,
-85.7289356123527)) ;
#195841=CARTESIAN_POINT('Ctrl Pts',(-8.32056395283379,-4.19999999994862,
-85.7289356123528)) ;
#195842=CARTESIAN_POINT('Ctrl Pts',(0.212109576017282,3.00000000005139,
-86.0373331136874)) ;
#195843=CARTESIAN_POINT('Ctrl Pts',(0.212109576017282,-4.19999999994861,
-86.0373331136875)) ;
#195844=CARTESIAN_POINT('',(0.212109576017269,3.00000000005139,-86.0373331136874)) ;
#195845=CARTESIAN_POINT('Origin',(0.221980326072865,3.00000000005143,-90.0393310222739)) ;
#195846=CARTESIAN_POINT('',(0.212109576017269,-2.99999999994861,-86.0373331136874)) ;
#195847=CARTESIAN_POINT('',(0.212109576017269,3.00000000005139,-86.0373331136874)) ;
#195848=CARTESIAN_POINT('Origin',(0.221980326071444,-2.99999999994857,-90.0393310222733)) ;
#195849=CARTESIAN_POINT('Origin',(0.217044951043621,3.00000000005141,-88.0383320679796)) ;
#195850=CARTESIAN_POINT('',(0.221980326069911,3.00000000005143,-90.039331022272)) ;
#195851=CARTESIAN_POINT('',(0.212109576017269,3.00000000005139,-86.0373331136874)) ;
#195852=CARTESIAN_POINT('',(0.221980326069911,-2.99999999994857,-90.0393310222721)) ;
#195853=CARTESIAN_POINT('',(0.221980326069911,3.00000000005143,-90.039331022272)) ;
#195854=CARTESIAN_POINT('',(0.212109576017269,-2.99999999994861,-86.0373331136874)) ;
#195855=CARTESIAN_POINT('Origin',(0.56606241707283,3.00000000005143,-90.0371668309801)) ;
#195856=CARTESIAN_POINT('',(0.910144508075746,3.00000000005143,-90.0350026396881)) ;
#195857=CARTESIAN_POINT('',(0.221980326069911,3.00000000005143,-90.039331022272)) ;
#195858=CARTESIAN_POINT('',(0.910144508075746,-2.99999999994857,-90.0350026396881)) ;
#195859=CARTESIAN_POINT('',(0.910144508075746,3.00000000005143,-90.0350026396881)) ;
#195860=CARTESIAN_POINT('',(0.221980326069911,-2.99999999994857,-90.0393310222721)) ;
#195861=CARTESIAN_POINT('Ctrl Pts',(0.910144508075857,3.00000000005143,
-90.0350026396881)) ;
#195862=CARTESIAN_POINT('Ctrl Pts',(0.910144508075857,-4.19999999994857,
-90.0350026396882)) ;
#195863=CARTESIAN_POINT('Ctrl Pts',(0.910065839387194,3.00000000005143,
-90.0336883823031)) ;
#195864=CARTESIAN_POINT('Ctrl Pts',(0.910065839387194,-4.19999999994857,
-90.0336883823032)) ;
#195865=CARTESIAN_POINT('Ctrl Pts',(0.909989061449121,3.00000000005143,
-90.0323740141851)) ;
#195866=CARTESIAN_POINT('Ctrl Pts',(0.909989061449121,-4.19999999994857,
-90.0323740141852)) ;
#195867=CARTESIAN_POINT('Ctrl Pts',(0.681991038044217,3.00000000005139,
-86.1292562557081)) ;
#195868=CARTESIAN_POINT('Ctrl Pts',(0.681991038044217,-4.19999999994861,
-86.1292562557082)) ;
#195869=CARTESIAN_POINT('Ctrl Pts',(9.20015800540581,3.00000000005138,-85.544057071727)) ;
#195870=CARTESIAN_POINT('Ctrl Pts',(9.20015800540581,-4.19999999994862,
-85.5440570717271)) ;
#195871=CARTESIAN_POINT('',(9.2001580054058,3.00000000005138,-85.544057071727)) ;
#195872=CARTESIAN_POINT('Origin',(9.62829737384105,3.00000000005142,-89.5230998426979)) ;
#195873=CARTESIAN_POINT('',(9.2001580054058,-2.99999999994862,-85.5440570717271)) ;
#195874=CARTESIAN_POINT('',(9.2001580054058,3.00000000005138,-85.544057071727)) ;
#195875=CARTESIAN_POINT('Origin',(9.62829737384009,-2.99999999994858,-89.5230998426976)) ;
#195876=CARTESIAN_POINT('Origin',(9.41422768962381,3.0000000000514,-87.5335784572127)) ;
#195877=CARTESIAN_POINT('',(9.62829737384209,3.00000000005142,-89.5230998426984)) ;
#195878=CARTESIAN_POINT('',(9.2001580054058,3.00000000005138,-85.544057071727)) ;
#195879=CARTESIAN_POINT('',(9.62829737384209,-2.99999999994858,-89.5230998426985)) ;
#195880=CARTESIAN_POINT('',(9.62829737384209,3.00000000005142,-89.5230998426984)) ;
#195881=CARTESIAN_POINT('',(9.2001580054058,-2.99999999994862,-85.5440570717271)) ;
#195882=CARTESIAN_POINT('Origin',(9.97026832755857,3.00000000005142,-89.4849811348624)) ;
#195883=CARTESIAN_POINT('',(10.3122392812754,3.00000000005142,-89.4468624270263)) ;
#195884=CARTESIAN_POINT('',(9.62829737384209,3.00000000005142,-89.5230998426984)) ;
#195885=CARTESIAN_POINT('',(10.3122392812754,-2.99999999994858,-89.4468624270264)) ;
#195886=CARTESIAN_POINT('',(10.3122392812754,3.00000000005142,-89.4468624270263)) ;
#195887=CARTESIAN_POINT('',(9.62829737384209,-2.99999999994858,-89.5230998426985)) ;
#195888=CARTESIAN_POINT('Ctrl Pts',(10.3122392812753,3.00000000005142,-89.4468624270263)) ;
#195889=CARTESIAN_POINT('Ctrl Pts',(10.3122392812753,-4.19999999994858,
-89.4468624270264)) ;
#195890=CARTESIAN_POINT('Ctrl Pts',(10.312023666237,3.00000000005142,-89.4455635923977)) ;
#195891=CARTESIAN_POINT('Ctrl Pts',(10.312023666237,-4.19999999994858,-89.4455635923978)) ;
#195892=CARTESIAN_POINT('Ctrl Pts',(10.3118099200172,3.00000000005142,-89.4442644500057)) ;
#195893=CARTESIAN_POINT('Ctrl Pts',(10.3118099200172,-4.19999999994858,
-89.4442644500058)) ;
#195894=CARTESIAN_POINT('Ctrl Pts',(9.67707399239405,3.00000000005138,-85.5863606620143)) ;
#195895=CARTESIAN_POINT('Ctrl Pts',(9.67707399239405,-4.19999999994862,
-85.5863606620144)) ;
#195896=CARTESIAN_POINT('Ctrl Pts',(18.0874075784307,3.00000000005137,-84.1139763574378)) ;
#195897=CARTESIAN_POINT('Ctrl Pts',(18.0874075784307,-4.19999999994863,
-84.1139763574379)) ;
#195898=CARTESIAN_POINT('',(18.0874075784309,3.00000000005137,-84.1139763574378)) ;
#195899=CARTESIAN_POINT('Origin',(18.9291247807328,3.00000000005141,-88.0264687655279)) ;
#195900=CARTESIAN_POINT('',(18.0874075784309,-2.99999999994863,-84.1139763574379)) ;
#195901=CARTESIAN_POINT('',(18.0874075784309,3.00000000005137,-84.1139763574378)) ;
#195902=CARTESIAN_POINT('Origin',(18.9291247807335,-2.99999999994859,-88.026468765528)) ;
#195903=CARTESIAN_POINT('Origin',(18.5082661795829,3.00000000005139,-86.0702225614833)) ;
#195904=CARTESIAN_POINT('',(18.9291247807354,3.00000000005141,-88.026468765529)) ;
#195905=CARTESIAN_POINT('',(18.0874075784309,3.00000000005137,-84.1139763574378)) ;
#195906=CARTESIAN_POINT('',(18.9291247807354,-2.99999999994859,-88.026468765529)) ;
#195907=CARTESIAN_POINT('',(18.9291247807354,3.00000000005141,-88.026468765529)) ;
#195908=CARTESIAN_POINT('',(18.0874075784309,-2.99999999994863,-84.1139763574379)) ;
#195909=CARTESIAN_POINT('Origin',(19.2652378918346,3.00000000005141,-87.9528131776886)) ;
#195910=CARTESIAN_POINT('',(19.6013510029341,3.00000000005141,-87.8791575898483)) ;
#195911=CARTESIAN_POINT('',(18.9291247807354,3.00000000005141,-88.026468765529)) ;
#195912=CARTESIAN_POINT('',(19.6013510029341,-2.99999999994859,-87.8791575898484)) ;
#195913=CARTESIAN_POINT('',(19.6013510029341,3.00000000005141,-87.8791575898483)) ;
#195914=CARTESIAN_POINT('',(18.9291247807354,-2.99999999994859,-88.026468765529)) ;
#195915=CARTESIAN_POINT('Ctrl Pts',(19.601351002934,3.00000000005141,-87.8791575898484)) ;
#195916=CARTESIAN_POINT('Ctrl Pts',(19.601351002934,-4.19999999994859,-87.8791575898484)) ;
#195917=CARTESIAN_POINT('Ctrl Pts',(19.6010008038698,3.00000000005141,-87.8778884082803)) ;
#195918=CARTESIAN_POINT('Ctrl Pts',(19.6010008038698,-4.19999999994859,
-87.8778884082804)) ;
#195919=CARTESIAN_POINT('Ctrl Pts',(19.6006524312164,3.00000000005141,-87.8766187252903)) ;
#195920=CARTESIAN_POINT('Ctrl Pts',(19.6006524312164,-4.19999999994859,
-87.8766187252903)) ;
#195921=CARTESIAN_POINT('Ctrl Pts',(18.5661328990248,3.00000000005137,-84.1061969090035)) ;
#195922=CARTESIAN_POINT('Ctrl Pts',(18.5661328990248,-4.19999999994863,
-84.1061969090036)) ;
#195923=CARTESIAN_POINT('Ctrl Pts',(26.7764877289929,3.00000000005134,-81.7627592343891)) ;
#195924=CARTESIAN_POINT('Ctrl Pts',(26.7764877289929,-4.19999999994866,
-81.7627592343892)) ;
#195925=CARTESIAN_POINT('',(26.7764877289931,3.00000000005134,-81.7627592343891)) ;
#195926=CARTESIAN_POINT('Origin',(28.0225607353579,3.00000000005138,-85.5658351940353)) ;
#195927=CARTESIAN_POINT('',(26.7764877289931,-2.99999999994866,-81.7627592343891)) ;
#195928=CARTESIAN_POINT('',(26.7764877289931,3.00000000005134,-81.7627592343891)) ;
#195929=CARTESIAN_POINT('Origin',(28.022560735356,-2.99999999994862,-85.5658351940352)) ;
#195930=CARTESIAN_POINT('Origin',(27.399524232175,3.00000000005136,-83.6642972142119)) ;
#195931=CARTESIAN_POINT('',(28.0225607353573,3.00000000005138,-85.5658351940347)) ;
#195932=CARTESIAN_POINT('',(26.7764877289931,3.00000000005134,-81.7627592343891)) ;
#195933=CARTESIAN_POINT('',(28.0225607353573,-2.99999999994862,-85.5658351940348)) ;
#195934=CARTESIAN_POINT('',(28.0225607353573,3.00000000005138,-85.5658351940347)) ;
#195935=CARTESIAN_POINT('',(26.7764877289931,-2.99999999994866,-81.7627592343891)) ;
#195936=CARTESIAN_POINT('Origin',(28.3491334782577,3.00000000005138,-85.4574497122239)) ;
#195937=CARTESIAN_POINT('',(28.6757062211584,3.00000000005138,-85.3490642304132)) ;
#195938=CARTESIAN_POINT('',(28.0225607353573,3.00000000005138,-85.5658351940347)) ;
#195939=CARTESIAN_POINT('',(28.6757062211584,-2.99999999994862,-85.3490642304132)) ;
#195940=CARTESIAN_POINT('',(28.6757062211584,3.00000000005138,-85.3490642304132)) ;
#195941=CARTESIAN_POINT('',(28.0225607353573,-2.99999999994862,-85.5658351940348)) ;
#195942=CARTESIAN_POINT('Ctrl Pts',(28.6757062211582,3.00000000005138,-85.3490642304131)) ;
#195943=CARTESIAN_POINT('Ctrl Pts',(28.6757062211582,-4.19999999994862,
-85.3490642304132)) ;
#195944=CARTESIAN_POINT('Ctrl Pts',(28.6752252749223,3.00000000005138,-85.3478386073249)) ;
#195945=CARTESIAN_POINT('Ctrl Pts',(28.6752252749223,-4.19999999994862,
-85.347838607325)) ;
#195946=CARTESIAN_POINT('Ctrl Pts',(28.6747460926787,3.00000000005138,-85.3466122946489)) ;
#195947=CARTESIAN_POINT('Ctrl Pts',(28.6747460926787,-4.19999999994862,
-85.346612294649)) ;
#195948=CARTESIAN_POINT('Ctrl Pts',(27.2517773684009,3.00000000005134,-81.704981980498)) ;
#195949=CARTESIAN_POINT('Ctrl Pts',(27.2517773684009,-4.19999999994866,
-81.7049819804981)) ;
#195950=CARTESIAN_POINT('Ctrl Pts',(35.1721990766558,3.00000000005131,-78.5161661294042)) ;
#195951=CARTESIAN_POINT('Ctrl Pts',(35.1721990766558,-4.19999999994869,
-78.5161661294042)) ;
#195952=CARTESIAN_POINT('',(35.1721990766558,3.00000000005131,-78.5161661294041)) ;
#195953=CARTESIAN_POINT('Origin',(36.8089756504653,3.00000000005135,-82.1681583445459)) ;
#195954=CARTESIAN_POINT('',(35.1721990766558,-2.99999999994869,-78.5161661294042)) ;
#195955=CARTESIAN_POINT('',(35.1721990766558,3.00000000005131,-78.5161661294041)) ;
#195956=CARTESIAN_POINT('Origin',(36.8089756504651,-2.99999999994865,-82.168158344546)) ;
#195957=CARTESIAN_POINT('Origin',(35.9905873635602,3.00000000005133,-80.3421622369752)) ;
#195958=CARTESIAN_POINT('',(36.8089756504646,3.00000000005135,-82.1681583445461)) ;
#195959=CARTESIAN_POINT('',(35.1721990766558,3.00000000005131,-78.5161661294041)) ;
#195960=CARTESIAN_POINT('',(36.8089756504646,-2.99999999994865,-82.1681583445461)) ;
#195961=CARTESIAN_POINT('',(36.8089756504646,3.00000000005135,-82.1681583445461)) ;
#195962=CARTESIAN_POINT('',(35.1721990766558,-2.99999999994869,-78.5161661294042)) ;
#195963=CARTESIAN_POINT('Origin',(37.1224300258553,3.00000000005135,-82.0262304627848)) ;
#195964=CARTESIAN_POINT('',(37.4358844012462,3.00000000005135,-81.8843025810235)) ;
#195965=CARTESIAN_POINT('',(36.8089756504646,3.00000000005135,-82.1681583445461)) ;
#195966=CARTESIAN_POINT('',(37.4358844012462,-2.99999999994866,-81.8843025810236)) ;
#195967=CARTESIAN_POINT('',(37.4358844012462,3.00000000005135,-81.8843025810235)) ;
#195968=CARTESIAN_POINT('',(36.8089756504646,-2.99999999994865,-82.1681583445461)) ;
#195969=CARTESIAN_POINT('Ctrl Pts',(37.4358844012461,3.00000000005135,-81.8843025810236)) ;
#195970=CARTESIAN_POINT('Ctrl Pts',(37.4358844012461,-4.19999999994867,
-81.8843025810236)) ;
#195971=CARTESIAN_POINT('Ctrl Pts',(37.4352779771861,3.00000000005135,-81.8831339445975)) ;
#195972=CARTESIAN_POINT('Ctrl Pts',(37.4352779771861,-4.19999999994867,
-81.8831339445976)) ;
#195973=CARTESIAN_POINT('Ctrl Pts',(37.4346732353735,3.00000000005135,-81.8819644379744)) ;
#195974=CARTESIAN_POINT('Ctrl Pts',(37.4346732353735,-4.19999999994867,
-81.8819644379745)) ;
#195975=CARTESIAN_POINT('Ctrl Pts',(35.6388456621278,3.00000000005131,-78.4090240897414)) ;
#195976=CARTESIAN_POINT('Ctrl Pts',(35.6388456621278,-4.1999999999487,-78.4090240897414)) ;
#195977=CARTESIAN_POINT('Ctrl Pts',(43.1825564509792,3.00000000005127,-74.4097673959352)) ;
#195978=CARTESIAN_POINT('Ctrl Pts',(43.1825564509792,-4.19999999994874,
-74.4097673959353)) ;
#195979=CARTESIAN_POINT('',(43.1825564509793,3.00000000005127,-74.4097673959352)) ;
#195980=CARTESIAN_POINT('Origin',(45.1921037255721,3.00000000005131,-77.8706638756356)) ;
#195981=CARTESIAN_POINT('',(43.1825564509793,-2.99999999994873,-74.4097673959353)) ;
#195982=CARTESIAN_POINT('',(43.1825564509793,3.00000000005127,-74.4097673959352)) ;
#195983=CARTESIAN_POINT('Origin',(45.1921037255727,-2.99999999994869,-77.8706638756356)) ;
#195984=CARTESIAN_POINT('Origin',(44.1873300882756,3.00000000005129,-76.1402156357854)) ;
#195985=CARTESIAN_POINT('',(45.1921037255719,3.0000000000513,-77.8706638756355)) ;
#195986=CARTESIAN_POINT('',(43.1825564509793,3.00000000005127,-74.4097673959352)) ;
#195987=CARTESIAN_POINT('',(45.1921037255719,-2.9999999999487,-77.8706638756356)) ;
#195988=CARTESIAN_POINT('',(45.1921037255719,3.00000000005131,-77.8706638756356)) ;
#195989=CARTESIAN_POINT('',(43.1825564509793,-2.99999999994873,-74.4097673959353)) ;
#195990=CARTESIAN_POINT('Origin',(45.4890054617218,3.0000000000513,-77.6967485854965)) ;
#195991=CARTESIAN_POINT('',(45.7859071978719,3.0000000000513,-77.5228332953575)) ;
#195992=CARTESIAN_POINT('',(45.1921037255719,3.00000000005131,-77.8706638756356)) ;
#195993=CARTESIAN_POINT('',(45.7859071978719,-2.9999999999487,-77.5228332953575)) ;
#195994=CARTESIAN_POINT('',(45.7859071978719,3.0000000000513,-77.5228332953575)) ;
#195995=CARTESIAN_POINT('',(45.1921037255719,-2.9999999999487,-77.8706638756356)) ;
#195996=CARTESIAN_POINT('Ctrl Pts',(45.7859071978719,3.0000000000513,-77.5228332953575)) ;
#195997=CARTESIAN_POINT('Ctrl Pts',(45.7859071978719,-4.1999999999487,-77.5228332953576)) ;
#195998=CARTESIAN_POINT('Ctrl Pts',(45.7851819400962,3.0000000000513,-77.5217344494193)) ;
#195999=CARTESIAN_POINT('Ctrl Pts',(45.7851819400962,-4.1999999999487,-77.5217344494194)) ;
#196000=CARTESIAN_POINT('Ctrl Pts',(45.7844582643926,3.0000000000513,-77.5206345622083)) ;
#196001=CARTESIAN_POINT('Ctrl Pts',(45.7844582643926,-4.1999999999487,-77.5206345622084)) ;
#196002=CARTESIAN_POINT('Ctrl Pts',(43.6354473048724,3.00000000005127,-74.2544344411075)) ;
#196003=CARTESIAN_POINT('Ctrl Pts',(43.6354473048724,-4.19999999994873,
-74.2544344411076)) ;
#196004=CARTESIAN_POINT('Ctrl Pts',(50.7197967002949,3.00000000005122,-69.4885535978252)) ;
#196005=CARTESIAN_POINT('Ctrl Pts',(50.7197967002949,-4.19999999994878,
-69.4885535978253)) ;
#196006=CARTESIAN_POINT('',(50.719796700295,3.00000000005122,-69.4885535978252)) ;
#196007=CARTESIAN_POINT('Origin',(53.0800976552053,3.00000000005125,-72.7204360360131)) ;
#196008=CARTESIAN_POINT('',(50.719796700295,-2.99999999994878,-69.4885535978253)) ;
#196009=CARTESIAN_POINT('',(50.719796700295,3.00000000005122,-69.4885535978252)) ;
#196010=CARTESIAN_POINT('Origin',(53.0800976552044,-2.99999999994875,-72.7204360360132)) ;
#196011=CARTESIAN_POINT('Origin',(51.8999471777507,3.00000000005124,-71.1044948169192)) ;
#196012=CARTESIAN_POINT('',(53.0800976552065,3.00000000005125,-72.7204360360133)) ;
#196013=CARTESIAN_POINT('',(50.719796700295,3.00000000005122,-69.4885535978252)) ;
#196014=CARTESIAN_POINT('',(53.0800976552065,-2.99999999994875,-72.7204360360134)) ;
#196015=CARTESIAN_POINT('',(53.0800976552065,3.00000000005125,-72.7204360360133)) ;
#196016=CARTESIAN_POINT('',(50.719796700295,-2.99999999994878,-69.4885535978253)) ;
#196017=CARTESIAN_POINT('Origin',(53.3571938345634,3.00000000005125,-72.5164387898095)) ;
#196018=CARTESIAN_POINT('',(53.6342900139205,3.00000000005125,-72.3124415436058)) ;
#196019=CARTESIAN_POINT('',(53.0800976552065,3.00000000005125,-72.7204360360133)) ;
#196020=CARTESIAN_POINT('',(53.6342900139205,-2.99999999994875,-72.3124415436058)) ;
#196021=CARTESIAN_POINT('',(53.6342900139205,3.00000000005125,-72.3124415436058)) ;
#196022=CARTESIAN_POINT('',(53.0800976552065,-2.99999999994875,-72.7204360360134)) ;
#196023=CARTESIAN_POINT('Ctrl Pts',(53.6342900139204,3.00000000005125,-72.3124415436058)) ;
#196024=CARTESIAN_POINT('Ctrl Pts',(53.6342900139204,-4.19999999994875,
-72.3124415436059)) ;
#196025=CARTESIAN_POINT('Ctrl Pts',(53.6334538685055,3.00000000005125,-72.3114245273411)) ;
#196026=CARTESIAN_POINT('Ctrl Pts',(53.6334538685055,-4.19999999994875,
-72.3114245273412)) ;
#196027=CARTESIAN_POINT('Ctrl Pts',(53.6326191876532,3.00000000005125,-72.3104063101364)) ;
#196028=CARTESIAN_POINT('Ctrl Pts',(53.6326191876532,-4.19999999994875,
-72.3104063101364)) ;
#196029=CARTESIAN_POINT('Ctrl Pts',(51.153969855641,3.00000000005122,-69.2867315881914)) ;
#196030=CARTESIAN_POINT('Ctrl Pts',(51.153969855641,-4.19999999994878,-69.2867315881915)) ;
#196031=CARTESIAN_POINT('Ctrl Pts',(57.7013402431622,3.00000000005116,-63.8064425832762)) ;
#196032=CARTESIAN_POINT('Ctrl Pts',(57.7013402431622,-4.19999999994884,
-63.8064425832763)) ;
#196033=CARTESIAN_POINT('',(57.7013402431622,3.00000000005116,-63.8064425832762)) ;
#196034=CARTESIAN_POINT('Origin',(60.38653492721,3.00000000005119,-66.7739017996431)) ;
#196035=CARTESIAN_POINT('',(57.7013402431622,-2.99999999994884,-63.8064425832763)) ;
#196036=CARTESIAN_POINT('',(57.7013402431622,3.00000000005116,-63.8064425832763)) ;
#196037=CARTESIAN_POINT('Origin',(60.3865349272097,-2.99999999994881,-66.7739017996433)) ;
#196038=CARTESIAN_POINT('Origin',(59.0439375851841,3.00000000005118,-65.2901721914601)) ;
#196039=CARTESIAN_POINT('',(60.386534927206,3.00000000005119,-66.7739017996442)) ;
#196040=CARTESIAN_POINT('',(57.7013402431622,3.00000000005116,-63.8064425832763)) ;
#196041=CARTESIAN_POINT('',(60.386534927206,-2.99999999994881,-66.7739017996442)) ;
#196042=CARTESIAN_POINT('',(60.386534927206,3.00000000005119,-66.7739017996442)) ;
#196043=CARTESIAN_POINT('',(57.7013402431622,-2.99999999994884,-63.8064425832763)) ;
#196044=CARTESIAN_POINT('Origin',(60.6407896260427,3.00000000005119,-66.5420576338941)) ;
#196045=CARTESIAN_POINT('',(60.8950443248793,3.00000000005119,-66.3102134681442)) ;
#196046=CARTESIAN_POINT('',(60.386534927206,3.00000000005119,-66.7739017996442)) ;
#196047=CARTESIAN_POINT('',(60.8950443248793,-2.99999999994881,-66.3102134681442)) ;
#196048=CARTESIAN_POINT('',(60.8950443248793,3.00000000005119,-66.3102134681442)) ;
#196049=CARTESIAN_POINT('',(60.386534927206,-2.99999999994881,-66.7739017996443)) ;
#196050=CARTESIAN_POINT('Ctrl Pts',(60.8950443248792,3.00000000005119,-66.3102134681441)) ;
#196051=CARTESIAN_POINT('Ctrl Pts',(60.8950443248792,-4.19999999994881,
-66.3102134681442)) ;
#196052=CARTESIAN_POINT('Ctrl Pts',(60.8941064528093,3.00000000005119,-66.3092894241962)) ;
#196053=CARTESIAN_POINT('Ctrl Pts',(60.8941064528093,-4.19999999994881,
-66.3092894241963)) ;
#196054=CARTESIAN_POINT('Ctrl Pts',(60.8931699117464,3.00000000005119,-66.3083640327988)) ;
#196055=CARTESIAN_POINT('Ctrl Pts',(60.8931699117464,-4.19999999994881,
-66.3083640327988)) ;
#196056=CARTESIAN_POINT('Ctrl Pts',(58.1120388080142,3.00000000005116,-63.5603427230073)) ;
#196057=CARTESIAN_POINT('Ctrl Pts',(58.1120388080142,-4.19999999994884,
-63.5603427230074)) ;
#196058=CARTESIAN_POINT('Ctrl Pts',(64.0506958275435,3.0000000000511,-57.4256887496219)) ;
#196059=CARTESIAN_POINT('Ctrl Pts',(64.0506958275435,-4.1999999999489,-57.425688749622)) ;
#196060=CARTESIAN_POINT('',(64.0506958275436,3.0000000000511,-57.4256887496218)) ;
#196061=CARTESIAN_POINT('Origin',(67.0313646858498,3.00000000005112,-60.0962126400144)) ;
#196062=CARTESIAN_POINT('',(64.0506958275436,-2.9999999999489,-57.4256887496219)) ;
#196063=CARTESIAN_POINT('',(64.0506958275436,3.0000000000511,-57.4256887496218)) ;
#196064=CARTESIAN_POINT('Origin',(67.0313646858495,-2.99999999994887,-60.0962126400146)) ;
#196065=CARTESIAN_POINT('Origin',(65.5410302566959,3.00000000005111,-58.7609506948182)) ;
#196066=CARTESIAN_POINT('',(67.0313646858483,3.00000000005112,-60.0962126400146)) ;
#196067=CARTESIAN_POINT('',(64.0506958275436,3.0000000000511,-57.4256887496218)) ;
#196068=CARTESIAN_POINT('',(67.0313646858483,-2.99999999994888,-60.0962126400146)) ;
#196069=CARTESIAN_POINT('',(67.0313646858483,3.00000000005112,-60.0962126400146)) ;
#196070=CARTESIAN_POINT('',(64.0506958275436,-2.9999999999489,-57.4256887496219)) ;
#196071=CARTESIAN_POINT('Origin',(67.2599922364783,3.00000000005112,-59.8390616879149)) ;
#196072=CARTESIAN_POINT('',(67.4886197871085,3.00000000005112,-59.5819107358151)) ;
#196073=CARTESIAN_POINT('',(67.0313646858483,3.00000000005112,-60.0962126400146)) ;
#196074=CARTESIAN_POINT('',(67.4886197871085,-2.99999999994888,-59.5819107358151)) ;
#196075=CARTESIAN_POINT('',(67.4886197871085,3.00000000005112,-59.5819107358151)) ;
#196076=CARTESIAN_POINT('',(67.0313646858483,-2.99999999994888,-60.0962126400146)) ;
#196077=CARTESIAN_POINT('Ctrl Pts',(67.4886197871084,3.00000000005112,-59.5819107358151)) ;
#196078=CARTESIAN_POINT('Ctrl Pts',(67.4886197871084,-4.19999999994888,
-59.5819107358152)) ;
#196079=CARTESIAN_POINT('Ctrl Pts',(67.487590463906,3.00000000005112,-59.5810897882029)) ;
#196080=CARTESIAN_POINT('Ctrl Pts',(67.487590463906,-4.19999999994888,-59.581089788203)) ;
#196081=CARTESIAN_POINT('Ctrl Pts',(67.4865623235722,3.00000000005112,-59.5802673613943)) ;
#196082=CARTESIAN_POINT('Ctrl Pts',(67.4865623235722,-4.19999999994888,
-59.5802673613944)) ;
#196083=CARTESIAN_POINT('Ctrl Pts',(64.4334201024814,3.00000000005109,-57.1380073602873)) ;
#196084=CARTESIAN_POINT('Ctrl Pts',(64.4334201024814,-4.19999999994891,
-57.1380073602874)) ;
#196085=CARTESIAN_POINT('Ctrl Pts',(69.6982985849691,3.00000000005102,-50.4162009711221)) ;
#196086=CARTESIAN_POINT('Ctrl Pts',(69.6982985849691,-4.19999999994898,
-50.4162009711222)) ;
#196087=CARTESIAN_POINT('',(69.6982985849692,3.00000000005102,-50.4162009711221)) ;
#196088=CARTESIAN_POINT('Origin',(72.9417847857807,3.00000000005105,-52.7605307169523)) ;
#196089=CARTESIAN_POINT('',(69.6982985849692,-2.99999999994898,-50.4162009711222)) ;
#196090=CARTESIAN_POINT('',(69.6982985849692,3.00000000005102,-50.4162009711221)) ;
#196091=CARTESIAN_POINT('Origin',(72.9417847857812,-2.99999999994895,-52.7605307169521)) ;
#196092=CARTESIAN_POINT('Origin',(71.3200416853732,3.00000000005104,-51.5883658440379)) ;
#196093=CARTESIAN_POINT('',(72.9417847857773,3.00000000005105,-52.7605307169534)) ;
#196094=CARTESIAN_POINT('',(69.6982985849692,3.00000000005102,-50.4162009711221)) ;
#196095=CARTESIAN_POINT('',(72.9417847857773,-2.99999999994895,-52.7605307169535)) ;
#196096=CARTESIAN_POINT('',(72.9417847857773,3.00000000005105,-52.7605307169534)) ;
#196097=CARTESIAN_POINT('',(69.6982985849692,-2.99999999994898,-50.4162009711222)) ;
#196098=CARTESIAN_POINT('Origin',(73.1422802969124,3.00000000005105,-52.4808903781475)) ;
#196099=CARTESIAN_POINT('',(73.3427758080477,3.00000000005104,-52.2012500393414)) ;
#196100=CARTESIAN_POINT('',(72.9417847857773,3.00000000005105,-52.7605307169534)) ;
#196101=CARTESIAN_POINT('',(73.3427758080477,-2.99999999994896,-52.2012500393415)) ;
#196102=CARTESIAN_POINT('',(73.3427758080477,3.00000000005104,-52.2012500393414)) ;
#196103=CARTESIAN_POINT('',(72.9417847857773,-2.99999999994895,-52.7605307169535)) ;
#196104=CARTESIAN_POINT('Ctrl Pts',(73.3427758080477,3.00000000005104,-52.2012500393414)) ;
#196105=CARTESIAN_POINT('Ctrl Pts',(73.3427758080477,-4.19999999994896,
-52.2012500393415)) ;
#196106=CARTESIAN_POINT('Ctrl Pts',(73.3416663111929,3.00000000005104,-52.2005411825387)) ;
#196107=CARTESIAN_POINT('Ctrl Pts',(73.3416663111929,-4.19999999994896,
-52.2005411825388)) ;
#196108=CARTESIAN_POINT('Ctrl Pts',(73.3405578361089,3.00000000005104,-52.1998307309995)) ;
#196109=CARTESIAN_POINT('Ctrl Pts',(73.3405578361089,-4.19999999994896,
-52.1998307309995)) ;
#196110=CARTESIAN_POINT('Ctrl Pts',(70.0488553627452,3.00000000005102,-50.0900899502248)) ;
#196111=CARTESIAN_POINT('Ctrl Pts',(70.0488553627452,-4.19999999994898,
-50.0900899502248)) ;
#196112=CARTESIAN_POINT('Ctrl Pts',(74.5822721977904,3.00000000005095,-42.8547766627078)) ;
#196113=CARTESIAN_POINT('Ctrl Pts',(74.5822721977904,-4.19999999994905,
-42.8547766627079)) ;
#196114=CARTESIAN_POINT('',(74.5822721977904,3.00000000005095,-42.8547766627078)) ;
#196115=CARTESIAN_POINT('Origin',(78.0530394275431,3.00000000005097,-44.8472272966999)) ;
#196116=CARTESIAN_POINT('',(74.5822721977904,-2.99999999994905,-42.8547766627079)) ;
#196117=CARTESIAN_POINT('',(74.5822721977904,3.00000000005095,-42.8547766627078)) ;
#196118=CARTESIAN_POINT('Origin',(78.053039427543,-2.99999999994903,-44.8472272967)) ;
#196119=CARTESIAN_POINT('Origin',(76.3176558126671,3.00000000005096,-43.851001979704)) ;
#196120=CARTESIAN_POINT('',(78.0530394275438,3.00000000005097,-44.8472272967001)) ;
#196121=CARTESIAN_POINT('',(74.5822721977904,3.00000000005095,-42.8547766627078)) ;
#196122=CARTESIAN_POINT('',(78.0530394275438,-2.99999999994903,-44.8472272967002)) ;
#196123=CARTESIAN_POINT('',(78.0530394275438,3.00000000005097,-44.8472272967001)) ;
#196124=CARTESIAN_POINT('',(74.5822721977904,-2.99999999994905,-42.8547766627079)) ;
#196125=CARTESIAN_POINT('Origin',(78.2232062284078,3.00000000005097,-44.5481613692583)) ;
#196126=CARTESIAN_POINT('',(78.3933730292717,3.00000000005096,-44.2490954418165)) ;
#196127=CARTESIAN_POINT('',(78.0530394275438,3.00000000005097,-44.8472272967001)) ;
#196128=CARTESIAN_POINT('',(78.3933730292717,-2.99999999994904,-44.2490954418166)) ;
#196129=CARTESIAN_POINT('',(78.3933730292717,3.00000000005096,-44.2490954418165)) ;
#196130=CARTESIAN_POINT('',(78.0530394275438,-2.99999999994903,-44.8472272967002)) ;
#196131=CARTESIAN_POINT('Ctrl Pts',(78.3933730292716,3.00000000005096,-44.2490954418165)) ;
#196132=CARTESIAN_POINT('Ctrl Pts',(78.3933730292716,-4.19999999994904,
-44.2490954418165)) ;
#196133=CARTESIAN_POINT('Ctrl Pts',(78.392195514644,3.00000000005096,-44.2485064422069)) ;
#196134=CARTESIAN_POINT('Ctrl Pts',(78.392195514644,-4.19999999994904,-44.248506442207)) ;
#196135=CARTESIAN_POINT('Ctrl Pts',(78.391018849496,3.00000000005096,-44.2479157497924)) ;
#196136=CARTESIAN_POINT('Ctrl Pts',(78.391018849496,-4.19999999994904,-44.2479157497925)) ;
#196137=CARTESIAN_POINT('Ctrl Pts',(74.8968207049897,3.00000000005094,-42.4938089508354)) ;
#196138=CARTESIAN_POINT('Ctrl Pts',(74.8968207049897,-4.19999999994906,
-42.4938089508355)) ;
#196139=CARTESIAN_POINT('Ctrl Pts',(78.6491068290694,3.00000000005087,-34.8242603714322)) ;
#196140=CARTESIAN_POINT('Ctrl Pts',(78.6491068290694,-4.19999999994914,
-34.8242603714323)) ;
#196141=CARTESIAN_POINT('',(78.6491068290693,3.00000000005087,-34.8242603714323)) ;
#196142=CARTESIAN_POINT('Origin',(82.3091286356952,3.00000000005088,-36.4430021874914)) ;
#196143=CARTESIAN_POINT('',(78.6491068290693,-2.99999999994913,-34.8242603714324)) ;
#196144=CARTESIAN_POINT('',(78.6491068290693,3.00000000005087,-34.8242603714323)) ;
#196145=CARTESIAN_POINT('Origin',(82.3091286356951,-2.99999999994912,-36.4430021874917)) ;
#196146=CARTESIAN_POINT('Origin',(80.4791177323813,3.00000000005087,-35.6336312794621)) ;
#196147=CARTESIAN_POINT('',(82.3091286356934,3.00000000005088,-36.4430021874921)) ;
#196148=CARTESIAN_POINT('',(78.6491068290693,3.00000000005087,-34.8242603714323)) ;
#196149=CARTESIAN_POINT('',(82.3091286356934,-2.99999999994912,-36.4430021874922)) ;
#196150=CARTESIAN_POINT('',(82.3091286356934,3.00000000005088,-36.4430021874921)) ;
#196151=CARTESIAN_POINT('',(78.6491068290693,-2.99999999994913,-34.8242603714324)) ;
#196152=CARTESIAN_POINT('Origin',(82.4471023432062,3.00000000005088,-36.1277873002989)) ;
#196153=CARTESIAN_POINT('',(82.5850760507188,3.00000000005088,-35.812572413106)) ;
#196154=CARTESIAN_POINT('',(82.3091286356934,3.00000000005088,-36.4430021874921)) ;
#196155=CARTESIAN_POINT('',(82.5850760507188,-2.99999999994912,-35.8125724131061)) ;
#196156=CARTESIAN_POINT('',(82.5850760507188,3.00000000005088,-35.812572413106)) ;
#196157=CARTESIAN_POINT('',(82.3091286356934,-2.99999999994912,-36.4430021874921)) ;
#196158=CARTESIAN_POINT('Ctrl Pts',(82.5850760507189,3.00000000005088,-35.8125724131059)) ;
#196159=CARTESIAN_POINT('Ctrl Pts',(82.5850760507189,-4.19999999994912,
-35.812572413106)) ;
#196160=CARTESIAN_POINT('Ctrl Pts',(82.5838434194159,3.00000000005088,-35.8121097238921)) ;
#196161=CARTESIAN_POINT('Ctrl Pts',(82.5838434194159,-4.19999999994912,
-35.8121097238922)) ;
#196162=CARTESIAN_POINT('Ctrl Pts',(82.5826114559914,3.00000000005088,-35.8116452623523)) ;
#196163=CARTESIAN_POINT('Ctrl Pts',(82.5826114559914,-4.19999999994912,
-35.8116452623524)) ;
#196164=CARTESIAN_POINT('Ctrl Pts',(78.9242008064232,3.00000000005086,-34.4323908063735)) ;
#196165=CARTESIAN_POINT('Ctrl Pts',(78.9242008064232,-4.19999999994914,
-34.4323908063736)) ;
#196166=CARTESIAN_POINT('Ctrl Pts',(81.8542453875446,3.00000000005078,-26.4126361142756)) ;
#196167=CARTESIAN_POINT('Ctrl Pts',(81.8542453875446,-4.19999999994922,
-26.4126361142757)) ;
#196168=CARTESIAN_POINT('',(81.8542453875448,3.00000000005078,-26.4126361142757)) ;
#196169=CARTESIAN_POINT('Origin',(85.6634218062183,3.00000000005079,-27.6399338383216)) ;
#196170=CARTESIAN_POINT('',(81.8542453875448,-2.99999999994922,-26.4126361142757)) ;
#196171=CARTESIAN_POINT('',(81.8542453875448,3.00000000005078,-26.4126361142757)) ;
#196172=CARTESIAN_POINT('Origin',(85.6634218062184,-2.99999999994921,-27.6399338383216)) ;
#196173=CARTESIAN_POINT('Origin',(83.7588335968811,3.00000000005079,-27.0262849762992)) ;
#196174=CARTESIAN_POINT('',(85.6634218062177,3.00000000005079,-27.6399338383229)) ;
#196175=CARTESIAN_POINT('',(81.8542453875448,3.00000000005078,-26.4126361142757)) ;
#196176=CARTESIAN_POINT('',(85.6634218062177,-2.99999999994921,-27.639933838323)) ;
#196177=CARTESIAN_POINT('',(85.6634218062177,3.00000000005079,-27.6399338383229)) ;
#196178=CARTESIAN_POINT('',(81.8542453875448,-2.99999999994922,-26.4126361142757)) ;
#196179=CARTESIAN_POINT('Origin',(85.7676907515669,3.00000000005079,-27.3120235516457)) ;
#196180=CARTESIAN_POINT('',(85.8719596969164,3.00000000005079,-26.9841132649686)) ;
#196181=CARTESIAN_POINT('',(85.6634218062177,3.00000000005079,-27.6399338383229)) ;
#196182=CARTESIAN_POINT('',(85.8719596969164,-2.99999999994921,-26.9841132649687)) ;
#196183=CARTESIAN_POINT('',(85.8719596969164,3.00000000005079,-26.9841132649686)) ;
#196184=CARTESIAN_POINT('',(85.6634218062177,-2.99999999994921,-27.639933838323)) ;
#196185=CARTESIAN_POINT('Ctrl Pts',(85.8719596969164,3.00000000005079,-26.9841132649686)) ;
#196186=CARTESIAN_POINT('Ctrl Pts',(85.8719596969164,-4.19999999994922,
-26.9841132649687)) ;
#196187=CARTESIAN_POINT('Ctrl Pts',(85.8706854539043,3.00000000005079,-26.9837819554707)) ;
#196188=CARTESIAN_POINT('Ctrl Pts',(85.8706854539043,-4.19999999994922,
-26.9837819554707)) ;
#196189=CARTESIAN_POINT('Ctrl Pts',(85.8694116898534,3.00000000005079,-26.9834488135434)) ;
#196190=CARTESIAN_POINT('Ctrl Pts',(85.8694116898534,-4.19999999994922,
-26.9834488135435)) ;
#196191=CARTESIAN_POINT('Ctrl Pts',(82.0868708478707,3.00000000005078,-25.9941581009892)) ;
#196192=CARTESIAN_POINT('Ctrl Pts',(82.0868708478707,-4.19999999994923,
-25.9941581009893)) ;
#196193=CARTESIAN_POINT('Ctrl Pts',(84.1625717044526,3.00000000005069,-17.7120634068452)) ;
#196194=CARTESIAN_POINT('Ctrl Pts',(84.1625717044526,-4.19999999994931,
-17.7120634068453)) ;
#196195=CARTESIAN_POINT('',(84.1625717044528,3.00000000005069,-17.7120634068453)) ;
#196196=CARTESIAN_POINT('Origin',(88.0791686012132,3.0000000000507,-18.5344705081823)) ;
#196197=CARTESIAN_POINT('',(84.1625717044528,-2.99999999994931,-17.7120634068454)) ;
#196198=CARTESIAN_POINT('',(84.1625717044528,3.00000000005069,-17.7120634068453)) ;
#196199=CARTESIAN_POINT('Origin',(88.0791686012132,-2.9999999999493,-18.5344705081823)) ;
#196200=CARTESIAN_POINT('Origin',(86.1208701528311,3.0000000000507,-18.1232669575159)) ;
#196201=CARTESIAN_POINT('',(88.0791686012095,3.0000000000507,-18.5344705081866)) ;
#196202=CARTESIAN_POINT('',(84.1625717044528,3.00000000005069,-17.7120634068453)) ;
#196203=CARTESIAN_POINT('',(88.0791686012095,-2.9999999999493,-18.5344705081866)) ;
#196204=CARTESIAN_POINT('',(88.0791686012095,3.0000000000507,-18.5344705081866)) ;
#196205=CARTESIAN_POINT('',(84.1625717044528,-2.99999999994931,-17.7120634068453)) ;
#196206=CARTESIAN_POINT('Origin',(88.1485903920104,3.0000000000507,-18.1974574757458)) ;
#196207=CARTESIAN_POINT('',(88.2180121828114,3.00000000005069,-17.8604444433051)) ;
#196208=CARTESIAN_POINT('',(88.0791686012095,3.0000000000507,-18.5344705081866)) ;
#196209=CARTESIAN_POINT('',(88.2180121828114,-2.99999999994931,-17.8604444433052)) ;
#196210=CARTESIAN_POINT('',(88.2180121828114,3.00000000005069,-17.8604444433051)) ;
#196211=CARTESIAN_POINT('',(88.0791686012095,-2.9999999999493,-18.5344705081866)) ;
#196212=CARTESIAN_POINT('Ctrl Pts',(88.2180121828113,3.00000000005069,-17.8604444433051)) ;
#196213=CARTESIAN_POINT('Ctrl Pts',(88.2180121828113,-4.19999999994931,
-17.8604444433051)) ;
#196214=CARTESIAN_POINT('Ctrl Pts',(88.2167102889633,3.00000000005069,-17.8602481434188)) ;
#196215=CARTESIAN_POINT('Ctrl Pts',(88.2167102889633,-4.19999999994931,
-17.8602481434189)) ;
#196216=CARTESIAN_POINT('Ctrl Pts',(88.2154086799115,3.00000000005069,-17.8600499710769)) ;
#196217=CARTESIAN_POINT('Ctrl Pts',(88.2154086799115,-4.19999999994931,
-17.860049971077)) ;
#196218=CARTESIAN_POINT('Ctrl Pts',(84.3501799545264,3.00000000005069,-17.2715618780168)) ;
#196219=CARTESIAN_POINT('Ctrl Pts',(84.3501799545264,-4.19999999994932,
-17.2715618780169)) ;
#196220=CARTESIAN_POINT('Ctrl Pts',(85.5487952736163,3.0000000000506,-8.81786754443537)) ;
#196221=CARTESIAN_POINT('Ctrl Pts',(85.5487952736163,-4.1999999999494,-8.81786754443545)) ;
#196222=CARTESIAN_POINT('',(85.5487952736163,3.0000000000506,-8.81786754443542)) ;
#196223=CARTESIAN_POINT('Origin',(89.5299015932572,3.00000000005061,-9.22637355876851)) ;
#196224=CARTESIAN_POINT('',(85.5487952736163,-2.9999999999494,-8.81786754443548)) ;
#196225=CARTESIAN_POINT('',(85.5487952736163,3.0000000000506,-8.81786754443542)) ;
#196226=CARTESIAN_POINT('Origin',(89.5299015932573,-2.99999999994939,-9.2263735587685)) ;
#196227=CARTESIAN_POINT('Origin',(87.5393484334361,3.0000000000506,-9.02212055160212)) ;
#196228=CARTESIAN_POINT('',(89.5299015932564,3.0000000000506,-9.22637355876897)) ;
#196229=CARTESIAN_POINT('',(85.5487952736163,3.0000000000506,-8.81786754443542)) ;
#196230=CARTESIAN_POINT('',(89.5299015932564,-2.9999999999494,-9.22637355876903)) ;
#196231=CARTESIAN_POINT('',(89.5299015932564,3.0000000000506,-9.22637355876897)) ;
#196232=CARTESIAN_POINT('',(85.5487952736163,-2.9999999999494,-8.81786754443549)) ;
#196233=CARTESIAN_POINT('Origin',(89.5637156298411,3.0000000000506,-8.88395016587238)) ;
#196234=CARTESIAN_POINT('',(89.5975296664262,3.0000000000506,-8.54152677297597)) ;
#196235=CARTESIAN_POINT('',(89.5299015932564,3.0000000000506,-9.22637355876897)) ;
#196236=CARTESIAN_POINT('',(89.5975296664262,-2.9999999999494,-8.54152677297603)) ;
#196237=CARTESIAN_POINT('',(89.5975296664262,3.0000000000506,-8.54152677297597)) ;
#196238=CARTESIAN_POINT('',(89.5299015932564,-2.9999999999494,-9.22637355876903)) ;
#196239=CARTESIAN_POINT('Ctrl Pts',(89.597529666426,3.0000000000506,-8.54152677297593)) ;
#196240=CARTESIAN_POINT('Ctrl Pts',(89.597529666426,-4.1999999999494,-8.541526772976)) ;
#196241=CARTESIAN_POINT('Ctrl Pts',(89.5962143855631,3.0000000000506,-8.54146763340456)) ;
#196242=CARTESIAN_POINT('Ctrl Pts',(89.5962143855631,-4.1999999999494,-8.54146763340463)) ;
#196243=CARTESIAN_POINT('Ctrl Pts',(89.5948991922115,3.0000000000506,-8.54140660186496)) ;
#196244=CARTESIAN_POINT('Ctrl Pts',(89.5948991922115,-4.1999999999494,-8.54140660186504)) ;
#196245=CARTESIAN_POINT('Ctrl Pts',(85.6893308381908,3.0000000000506,-8.36016872699591)) ;
#196246=CARTESIAN_POINT('Ctrl Pts',(85.6893308381908,-4.19999999994941,
-8.36016872699598)) ;
#196247=CARTESIAN_POINT('Ctrl Pts',(85.9977283395256,3.00000000005051,0.172504801855261)) ;
#196248=CARTESIAN_POINT('Ctrl Pts',(85.9977283395256,-4.19999999994949,
0.172504801855188)) ;
#196249=CARTESIAN_POINT('',(85.9977283395256,3.00000000005051,0.172504801855252)) ;
#196250=CARTESIAN_POINT('Origin',(89.999726248113,3.00000000005051,0.182375551912067)) ;
#196251=CARTESIAN_POINT('',(85.9977283395256,-2.99999999994949,0.172504801855191)) ;
#196252=CARTESIAN_POINT('',(85.9977283395256,3.00000000005051,0.172504801855252)) ;
#196253=CARTESIAN_POINT('Origin',(89.999726248113,-2.99999999994949,0.182375551911981)) ;
#196254=CARTESIAN_POINT('Origin',(87.9987272938181,3.00000000005051,0.177440176881581)) ;
#196255=CARTESIAN_POINT('',(89.9997262481107,3.00000000005051,0.182375551907936)) ;
#196256=CARTESIAN_POINT('',(85.9977283395256,3.00000000005051,0.172504801855252)) ;
#196257=CARTESIAN_POINT('',(89.9997262481107,-2.99999999994949,0.182375551907875)) ;
#196258=CARTESIAN_POINT('',(89.9997262481107,3.00000000005051,0.182375551907936)) ;
#196259=CARTESIAN_POINT('',(85.9977283395256,-2.99999999994949,0.172504801855191)) ;
#196260=CARTESIAN_POINT('Origin',(89.9975620568185,3.00000000005051,0.52645764291101)) ;
#196261=CARTESIAN_POINT('',(89.9953978655267,3.0000000000505,0.870539733914034)) ;
#196262=CARTESIAN_POINT('',(89.9997262481107,3.00000000005051,0.182375551907936)) ;
#196263=CARTESIAN_POINT('',(89.9953978655267,-2.9999999999495,0.870539733913973)) ;
#196264=CARTESIAN_POINT('',(89.9953978655267,3.0000000000505,0.870539733914034)) ;
#196265=CARTESIAN_POINT('',(89.9997262481107,-2.99999999994949,0.182375551907875)) ;
#196266=CARTESIAN_POINT('Ctrl Pts',(89.9953978655265,3.0000000000505,0.870539733914057)) ;
#196267=CARTESIAN_POINT('Ctrl Pts',(89.9953978655265,-4.1999999999495,0.870539733913984)) ;
#196268=CARTESIAN_POINT('Ctrl Pts',(89.9940836081412,3.0000000000505,0.870461065225228)) ;
#196269=CARTESIAN_POINT('Ctrl Pts',(89.9940836081412,-4.1999999999495,0.870461065225154)) ;
#196270=CARTESIAN_POINT('Ctrl Pts',(89.9927692400232,3.0000000000505,0.870384287287441)) ;
#196271=CARTESIAN_POINT('Ctrl Pts',(89.9927692400232,-4.1999999999495,0.870384287287368)) ;
#196272=CARTESIAN_POINT('Ctrl Pts',(86.0896514815462,3.0000000000505,0.642386263882138)) ;
#196273=CARTESIAN_POINT('Ctrl Pts',(86.0896514815462,-4.1999999999495,0.642386263882064)) ;
#196274=CARTESIAN_POINT('Ctrl Pts',(85.5044522975655,3.00000000005042,9.16055323124422)) ;
#196275=CARTESIAN_POINT('Ctrl Pts',(85.5044522975655,-4.19999999994958,
9.16055323124414)) ;
#196276=CARTESIAN_POINT('',(85.5044522975654,3.00000000005042,9.16055323124416)) ;
#196277=CARTESIAN_POINT('Origin',(89.4834950685362,3.00000000005041,9.58869259967878)) ;
#196278=CARTESIAN_POINT('',(85.5044522975654,-2.99999999994958,9.1605532312441)) ;
#196279=CARTESIAN_POINT('',(85.5044522975654,3.00000000005042,9.16055323124416)) ;
#196280=CARTESIAN_POINT('Origin',(89.4834950685362,-2.99999999994959,9.58869259967875)) ;
#196281=CARTESIAN_POINT('Origin',(87.4939736830512,3.00000000005042,9.37462291546208)) ;
#196282=CARTESIAN_POINT('',(89.4834950685366,3.00000000005041,9.58869259968009)) ;
#196283=CARTESIAN_POINT('',(85.5044522975654,3.00000000005042,9.16055323124416)) ;
#196284=CARTESIAN_POINT('',(89.4834950685366,-2.99999999994959,9.58869259968003)) ;
#196285=CARTESIAN_POINT('',(89.4834950685366,3.00000000005041,9.58869259968009)) ;
#196286=CARTESIAN_POINT('',(85.5044522975654,-2.99999999994958,9.1605532312441)) ;
#196287=CARTESIAN_POINT('Origin',(89.4453763607007,3.00000000005041,9.93066355339673)) ;
#196288=CARTESIAN_POINT('',(89.4072576528648,3.00000000005041,10.2726345071134)) ;
#196289=CARTESIAN_POINT('',(89.4834950685366,3.00000000005041,9.58869259968009)) ;
#196290=CARTESIAN_POINT('',(89.4072576528648,-2.99999999994959,10.2726345071134)) ;
#196291=CARTESIAN_POINT('',(89.4072576528648,3.00000000005041,10.2726345071134)) ;
#196292=CARTESIAN_POINT('',(89.4834950685366,-2.99999999994959,9.58869259968003)) ;
#196293=CARTESIAN_POINT('Ctrl Pts',(89.4072576528647,3.00000000005041,10.2726345071135)) ;
#196294=CARTESIAN_POINT('Ctrl Pts',(89.4072576528647,-4.19999999994959,
10.2726345071134)) ;
#196295=CARTESIAN_POINT('Ctrl Pts',(89.4059588182358,3.00000000005041,10.2724188920751)) ;
#196296=CARTESIAN_POINT('Ctrl Pts',(89.4059588182358,-4.19999999994959,
10.2724188920751)) ;
#196297=CARTESIAN_POINT('Ctrl Pts',(89.404659675844,3.00000000005041,10.2722051458554)) ;
#196298=CARTESIAN_POINT('Ctrl Pts',(89.404659675844,-4.19999999994959,10.2722051458553)) ;
#196299=CARTESIAN_POINT('Ctrl Pts',(85.5467558878525,3.00000000005041,9.63746921823198)) ;
#196300=CARTESIAN_POINT('Ctrl Pts',(85.5467558878525,-4.19999999994959,
9.63746921823191)) ;
#196301=CARTESIAN_POINT('Ctrl Pts',(84.0743715832764,3.00000000005033,18.0478028042689)) ;
#196302=CARTESIAN_POINT('Ctrl Pts',(84.0743715832764,-4.19999999994967,
18.0478028042688)) ;
#196303=CARTESIAN_POINT('',(84.0743715832764,3.00000000005033,18.0478028042688)) ;
#196304=CARTESIAN_POINT('Origin',(87.986863991367,3.00000000005032,18.8895200065722)) ;
#196305=CARTESIAN_POINT('',(84.0743715832764,-2.99999999994967,18.0478028042687)) ;
#196306=CARTESIAN_POINT('',(84.0743715832764,3.00000000005033,18.0478028042688)) ;
#196307=CARTESIAN_POINT('Origin',(87.986863991367,-2.99999999994968,18.8895200065722)) ;
#196308=CARTESIAN_POINT('Origin',(86.0306177873216,3.00000000005032,18.4686614054212)) ;
#196309=CARTESIAN_POINT('',(87.9868639913669,3.00000000005032,18.8895200065734)) ;
#196310=CARTESIAN_POINT('',(84.0743715832764,3.00000000005033,18.0478028042688)) ;
#196311=CARTESIAN_POINT('',(87.9868639913669,-2.99999999994968,18.8895200065733)) ;
#196312=CARTESIAN_POINT('',(87.9868639913669,3.00000000005032,18.8895200065734)) ;
#196313=CARTESIAN_POINT('',(84.0743715832764,-2.99999999994967,18.0478028042687)) ;
#196314=CARTESIAN_POINT('Origin',(87.9132084035267,3.00000000005032,19.2256331176729)) ;
#196315=CARTESIAN_POINT('',(87.8395528156865,3.00000000005031,19.5617462287721)) ;
#196316=CARTESIAN_POINT('',(87.9868639913669,3.00000000005032,18.8895200065734)) ;
#196317=CARTESIAN_POINT('',(87.8395528156865,-2.99999999994969,19.5617462287721)) ;
#196318=CARTESIAN_POINT('',(87.8395528156865,3.00000000005031,19.5617462287721)) ;
#196319=CARTESIAN_POINT('',(87.9868639913669,-2.99999999994968,18.8895200065733)) ;
#196320=CARTESIAN_POINT('Ctrl Pts',(87.8395528156866,3.00000000005031,19.5617462287722)) ;
#196321=CARTESIAN_POINT('Ctrl Pts',(87.8395528156866,-4.19999999994969,
19.5617462287721)) ;
#196322=CARTESIAN_POINT('Ctrl Pts',(87.8382836341184,3.00000000005031,19.5613960297078)) ;
#196323=CARTESIAN_POINT('Ctrl Pts',(87.8382836341184,-4.19999999994969,
19.5613960297077)) ;
#196324=CARTESIAN_POINT('Ctrl Pts',(87.8370139511282,3.00000000005031,19.5610476570545)) ;
#196325=CARTESIAN_POINT('Ctrl Pts',(87.8370139511282,-4.19999999994969,
19.5610476570545)) ;
#196326=CARTESIAN_POINT('Ctrl Pts',(84.0665921348418,3.00000000005032,18.526528124863)) ;
#196327=CARTESIAN_POINT('Ctrl Pts',(84.0665921348418,-4.19999999994968,
18.5265281248629)) ;
#196328=CARTESIAN_POINT('Ctrl Pts',(81.7231544602271,3.00000000005024,26.7368829548309)) ;
#196329=CARTESIAN_POINT('Ctrl Pts',(81.7231544602271,-4.19999999994976,
26.7368829548308)) ;
#196330=CARTESIAN_POINT('',(81.723154460227,3.00000000005024,26.7368829548309)) ;
#196331=CARTESIAN_POINT('Origin',(85.5262304198725,3.00000000005022,27.9829559611932)) ;
#196332=CARTESIAN_POINT('',(81.723154460227,-2.99999999994976,26.7368829548309)) ;
#196333=CARTESIAN_POINT('',(81.723154460227,3.00000000005024,26.7368829548309)) ;
#196334=CARTESIAN_POINT('Origin',(85.5262304198726,-2.99999999994977,27.9829559611934)) ;
#196335=CARTESIAN_POINT('Origin',(83.6246924400499,3.00000000005023,27.359919458013)) ;
#196336=CARTESIAN_POINT('',(85.5262304198725,3.00000000005023,27.9829559611952)) ;
#196337=CARTESIAN_POINT('',(81.723154460227,3.00000000005024,26.7368829548309)) ;
#196338=CARTESIAN_POINT('',(85.5262304198725,-2.99999999994977,27.9829559611951)) ;
#196339=CARTESIAN_POINT('',(85.5262304198725,3.00000000005023,27.9829559611952)) ;
#196340=CARTESIAN_POINT('',(81.723154460227,-2.99999999994976,26.7368829548309)) ;
#196341=CARTESIAN_POINT('Origin',(85.4178449380619,3.00000000005022,28.3095287040958)) ;
#196342=CARTESIAN_POINT('',(85.3094594562511,3.00000000005022,28.6361014469966)) ;
#196343=CARTESIAN_POINT('',(85.5262304198725,3.00000000005023,27.9829559611952)) ;
#196344=CARTESIAN_POINT('',(85.3094594562511,-2.99999999994978,28.6361014469965)) ;
#196345=CARTESIAN_POINT('',(85.3094594562511,3.00000000005022,28.6361014469966)) ;
#196346=CARTESIAN_POINT('',(85.5262304198725,-2.99999999994977,27.9829559611951)) ;
#196347=CARTESIAN_POINT('Ctrl Pts',(85.3094594562513,3.00000000005022,28.6361014469965)) ;
#196348=CARTESIAN_POINT('Ctrl Pts',(85.3094594562513,-4.19999999994978,
28.6361014469964)) ;
#196349=CARTESIAN_POINT('Ctrl Pts',(85.3082338331627,3.00000000005022,28.6356205007604)) ;
#196350=CARTESIAN_POINT('Ctrl Pts',(85.3082338331627,-4.19999999994978,
28.6356205007604)) ;
#196351=CARTESIAN_POINT('Ctrl Pts',(85.3070075204873,3.00000000005022,28.635141318517)) ;
#196352=CARTESIAN_POINT('Ctrl Pts',(85.3070075204873,-4.19999999994978,
28.635141318517)) ;
#196353=CARTESIAN_POINT('Ctrl Pts',(81.6653772063361,3.00000000005024,27.212172594239)) ;
#196354=CARTESIAN_POINT('Ctrl Pts',(81.6653772063361,-4.19999999994977,
27.212172594239)) ;
#196355=CARTESIAN_POINT('Ctrl Pts',(78.4765613552424,3.00000000005015,35.1325943024941)) ;
#196356=CARTESIAN_POINT('Ctrl Pts',(78.4765613552424,-4.19999999994985,
35.132594302494)) ;
#196357=CARTESIAN_POINT('',(78.4765613552424,3.00000000005015,35.1325943024941)) ;
#196358=CARTESIAN_POINT('Origin',(82.1285535703842,3.00000000005014,36.7693708763001)) ;
#196359=CARTESIAN_POINT('',(78.4765613552424,-2.99999999994985,35.132594302494)) ;
#196360=CARTESIAN_POINT('',(78.4765613552424,3.00000000005015,35.1325943024941)) ;
#196361=CARTESIAN_POINT('Origin',(82.1285535703842,-2.99999999994986,36.7693708763003)) ;
#196362=CARTESIAN_POINT('Origin',(80.3025574628131,3.00000000005015,35.9509825893984)) ;
#196363=CARTESIAN_POINT('',(82.1285535703842,3.00000000005014,36.7693708763029)) ;
#196364=CARTESIAN_POINT('',(78.4765613552424,3.00000000005015,35.1325943024941)) ;
#196365=CARTESIAN_POINT('',(82.1285535703842,-2.99999999994986,36.7693708763028)) ;
#196366=CARTESIAN_POINT('',(82.1285535703842,3.00000000005014,36.7693708763029)) ;
#196367=CARTESIAN_POINT('',(78.4765613552424,-2.99999999994985,35.132594302494)) ;
#196368=CARTESIAN_POINT('Origin',(81.9866256886228,3.00000000005013,37.0828252516937)) ;
#196369=CARTESIAN_POINT('',(81.8446978068619,3.00000000005013,37.3962796270845)) ;
#196370=CARTESIAN_POINT('',(82.1285535703842,3.00000000005014,36.7693708763029)) ;
#196371=CARTESIAN_POINT('',(81.8446978068619,-2.99999999994987,37.3962796270845)) ;
#196372=CARTESIAN_POINT('',(81.8446978068619,3.00000000005013,37.3962796270845)) ;
#196373=CARTESIAN_POINT('',(82.1285535703842,-2.99999999994986,36.7693708763028)) ;
#196374=CARTESIAN_POINT('Ctrl Pts',(81.8446978068617,3.00000000005013,37.3962796270845)) ;
#196375=CARTESIAN_POINT('Ctrl Pts',(81.8446978068617,-4.19999999994988,
37.3962796270845)) ;
#196376=CARTESIAN_POINT('Ctrl Pts',(81.8435291704356,3.00000000005013,37.3956732030243)) ;
#196377=CARTESIAN_POINT('Ctrl Pts',(81.8435291704356,-4.19999999994988,
37.3956732030242)) ;
#196378=CARTESIAN_POINT('Ctrl Pts',(81.8423596638126,3.00000000005013,37.3950684612118)) ;
#196379=CARTESIAN_POINT('Ctrl Pts',(81.8423596638126,-4.19999999994988,
37.3950684612117)) ;
#196380=CARTESIAN_POINT('Ctrl Pts',(78.3694193155791,3.00000000005015,35.5992408879661)) ;
#196381=CARTESIAN_POINT('Ctrl Pts',(78.3694193155791,-4.19999999994986,
35.599240887966)) ;
#196382=CARTESIAN_POINT('Ctrl Pts',(74.3701626217736,3.00000000005007,43.1429516768174)) ;
#196383=CARTESIAN_POINT('Ctrl Pts',(74.3701626217736,-4.19999999994994,
43.1429516768174)) ;
#196384=CARTESIAN_POINT('',(74.3701626217736,3.00000000005007,43.1429516768173)) ;
#196385=CARTESIAN_POINT('Origin',(77.8310591014742,3.00000000005005,45.1524989514095)) ;
#196386=CARTESIAN_POINT('',(74.3701626217736,-2.99999999994993,43.1429516768173)) ;
#196387=CARTESIAN_POINT('',(74.3701626217736,3.00000000005007,43.1429516768173)) ;
#196388=CARTESIAN_POINT('Origin',(77.8310591014742,-2.99999999994995,45.152498951409)) ;
#196389=CARTESIAN_POINT('Origin',(76.1006108616236,3.00000000005006,44.1477253141138)) ;
#196390=CARTESIAN_POINT('',(77.8310591014736,3.00000000005005,45.1524989514102)) ;
#196391=CARTESIAN_POINT('',(74.3701626217736,3.00000000005007,43.1429516768173)) ;
#196392=CARTESIAN_POINT('',(77.8310591014736,-2.99999999994995,45.1524989514101)) ;
#196393=CARTESIAN_POINT('',(77.8310591014736,3.00000000005005,45.1524989514102)) ;
#196394=CARTESIAN_POINT('',(74.3701626217736,-2.99999999994993,43.1429516768173)) ;
#196395=CARTESIAN_POINT('Origin',(77.6571438113347,3.00000000005005,45.4494006875601)) ;
#196396=CARTESIAN_POINT('',(77.4832285211958,3.00000000005005,45.74630242371)) ;
#196397=CARTESIAN_POINT('',(77.8310591014736,3.00000000005005,45.1524989514102)) ;
#196398=CARTESIAN_POINT('',(77.4832285211958,-2.99999999994995,45.7463024237099)) ;
#196399=CARTESIAN_POINT('',(77.4832285211958,3.00000000005004,45.7463024237099)) ;
#196400=CARTESIAN_POINT('',(77.8310591014736,-2.99999999994995,45.1524989514101)) ;
#196401=CARTESIAN_POINT('Ctrl Pts',(77.4832285211958,3.00000000005004,45.7463024237099)) ;
#196402=CARTESIAN_POINT('Ctrl Pts',(77.4832285211958,-4.19999999994996,
45.7463024237099)) ;
#196403=CARTESIAN_POINT('Ctrl Pts',(77.4821296752576,3.00000000005005,45.7455771659345)) ;
#196404=CARTESIAN_POINT('Ctrl Pts',(77.4821296752576,-4.19999999994995,
45.7455771659344)) ;
#196405=CARTESIAN_POINT('Ctrl Pts',(77.4810297880463,3.00000000005005,45.7448534902309)) ;
#196406=CARTESIAN_POINT('Ctrl Pts',(77.4810297880463,-4.19999999994995,
45.7448534902308)) ;
#196407=CARTESIAN_POINT('Ctrl Pts',(74.2148296669458,3.00000000005007,43.5958425307108)) ;
#196408=CARTESIAN_POINT('Ctrl Pts',(74.2148296669458,-4.19999999994993,
43.5958425307107)) ;
#196409=CARTESIAN_POINT('Ctrl Pts',(69.4489488236634,3.00000000005,50.6801919261331)) ;
#196410=CARTESIAN_POINT('Ctrl Pts',(69.4489488236634,-4.19999999995,50.680191926133)) ;
#196411=CARTESIAN_POINT('',(69.4489488236634,3.00000000005,50.6801919261331)) ;
#196412=CARTESIAN_POINT('Origin',(72.680831261851,3.00000000004997,53.0404928810471)) ;
#196413=CARTESIAN_POINT('',(69.4489488236634,-2.99999999995,50.680191926133)) ;
#196414=CARTESIAN_POINT('',(69.4489488236634,3.00000000005,50.6801919261331)) ;
#196415=CARTESIAN_POINT('Origin',(72.6808312618511,-2.99999999995003,53.0404928810464)) ;
#196416=CARTESIAN_POINT('Origin',(71.0648900427574,3.00000000004998,51.8603424035888)) ;
#196417=CARTESIAN_POINT('',(72.6808312618513,3.00000000004997,53.0404928810446)) ;
#196418=CARTESIAN_POINT('',(69.4489488236634,3.00000000005,50.6801919261331)) ;
#196419=CARTESIAN_POINT('',(72.6808312618513,-2.99999999995003,53.0404928810445)) ;
#196420=CARTESIAN_POINT('',(72.6808312618513,3.00000000004997,53.0404928810446)) ;
#196421=CARTESIAN_POINT('',(69.4489488236634,-2.99999999995,50.680191926133)) ;
#196422=CARTESIAN_POINT('Origin',(72.4768340156477,3.00000000004997,53.3175890604016)) ;
#196423=CARTESIAN_POINT('',(72.2728367694436,3.00000000004997,53.5946852397585)) ;
#196424=CARTESIAN_POINT('',(72.6808312618513,3.00000000004997,53.0404928810446)) ;
#196425=CARTESIAN_POINT('',(72.2728367694436,-2.99999999995003,53.5946852397584)) ;
#196426=CARTESIAN_POINT('',(72.2728367694436,3.00000000004997,53.5946852397585)) ;
#196427=CARTESIAN_POINT('',(72.6808312618513,-2.99999999995003,53.0404928810445)) ;
#196428=CARTESIAN_POINT('Ctrl Pts',(72.2728367694439,3.00000000004997,53.5946852397585)) ;
#196429=CARTESIAN_POINT('Ctrl Pts',(72.2728367694439,-4.19999999995003,
53.5946852397584)) ;
#196430=CARTESIAN_POINT('Ctrl Pts',(72.2718197531794,3.00000000004997,53.5938490943438)) ;
#196431=CARTESIAN_POINT('Ctrl Pts',(72.2718197531794,-4.19999999995003,
53.5938490943437)) ;
#196432=CARTESIAN_POINT('Ctrl Pts',(72.2708015359745,3.00000000004997,53.5930144134914)) ;
#196433=CARTESIAN_POINT('Ctrl Pts',(72.2708015359745,-4.19999999995003,
53.5930144134913)) ;
#196434=CARTESIAN_POINT('Ctrl Pts',(69.2471268140295,3.00000000004999,51.1143650814791)) ;
#196435=CARTESIAN_POINT('Ctrl Pts',(69.2471268140295,-4.19999999995001,
51.114365081479)) ;
#196436=CARTESIAN_POINT('Ctrl Pts',(63.7668378091141,3.00000000004992,57.6617354690004)) ;
#196437=CARTESIAN_POINT('Ctrl Pts',(63.7668378091141,-4.19999999995008,
57.6617354690003)) ;
#196438=CARTESIAN_POINT('',(63.7668378091141,3.00000000004992,57.6617354690004)) ;
#196439=CARTESIAN_POINT('Origin',(66.7342970254818,3.0000000000499,60.3469301530462)) ;
#196440=CARTESIAN_POINT('',(63.7668378091141,-2.99999999995008,57.6617354690003)) ;
#196441=CARTESIAN_POINT('',(63.7668378091141,3.00000000004992,57.6617354690003)) ;
#196442=CARTESIAN_POINT('Origin',(66.7342970254818,-2.9999999999501,60.3469301530459)) ;
#196443=CARTESIAN_POINT('Origin',(65.2505674172981,3.00000000004991,59.0043328110222)) ;
#196444=CARTESIAN_POINT('',(66.7342970254824,3.0000000000499,60.3469301530442)) ;
#196445=CARTESIAN_POINT('',(63.7668378091141,3.00000000004992,57.6617354690003)) ;
#196446=CARTESIAN_POINT('',(66.7342970254824,-2.9999999999501,60.3469301530441)) ;
#196447=CARTESIAN_POINT('',(66.7342970254824,3.0000000000499,60.3469301530442)) ;
#196448=CARTESIAN_POINT('',(63.7668378091141,-2.99999999995008,57.6617354690003)) ;
#196449=CARTESIAN_POINT('Origin',(66.5024528597322,3.00000000004989,60.6011848518809)) ;
#196450=CARTESIAN_POINT('',(66.2706086939821,3.00000000004989,60.8554395507177)) ;
#196451=CARTESIAN_POINT('',(66.7342970254824,3.0000000000499,60.3469301530442)) ;
#196452=CARTESIAN_POINT('',(66.2706086939821,-2.99999999995011,60.8554395507176)) ;
#196453=CARTESIAN_POINT('',(66.2706086939821,3.00000000004989,60.8554395507176)) ;
#196454=CARTESIAN_POINT('',(66.7342970254824,-2.9999999999501,60.3469301530441)) ;
#196455=CARTESIAN_POINT('Ctrl Pts',(66.2706086939821,3.00000000004989,60.8554395507177)) ;
#196456=CARTESIAN_POINT('Ctrl Pts',(66.2706086939821,-4.19999999995012,
60.8554395507177)) ;
#196457=CARTESIAN_POINT('Ctrl Pts',(66.2696846500344,3.00000000004989,60.8545016786479)) ;
#196458=CARTESIAN_POINT('Ctrl Pts',(66.2696846500344,-4.19999999995012,
60.8545016786478)) ;
#196459=CARTESIAN_POINT('Ctrl Pts',(66.2687592586371,3.00000000004989,60.853565137585)) ;
#196460=CARTESIAN_POINT('Ctrl Pts',(66.2687592586371,-4.19999999995012,
60.8535651375849)) ;
#196461=CARTESIAN_POINT('Ctrl Pts',(63.5207379488458,3.00000000004992,58.0724340338524)) ;
#196462=CARTESIAN_POINT('Ctrl Pts',(63.5207379488458,-4.19999999995009,
58.0724340338523)) ;
#196463=CARTESIAN_POINT('Ctrl Pts',(57.3860839754601,3.00000000004986,64.0110910533819)) ;
#196464=CARTESIAN_POINT('Ctrl Pts',(57.3860839754601,-4.19999999995015,
64.0110910533819)) ;
#196465=CARTESIAN_POINT('',(57.3860839754601,3.00000000004986,64.0110910533819)) ;
#196466=CARTESIAN_POINT('Origin',(60.0566078658524,3.00000000004983,66.9917599116882)) ;
#196467=CARTESIAN_POINT('',(57.3860839754601,-2.99999999995014,64.0110910533818)) ;
#196468=CARTESIAN_POINT('',(57.3860839754601,3.00000000004986,64.0110910533819)) ;
#196469=CARTESIAN_POINT('Origin',(60.0566078658524,-2.99999999995017,66.9917599116879)) ;
#196470=CARTESIAN_POINT('Origin',(58.7213459206563,3.00000000004985,65.5014254825341)) ;
#196471=CARTESIAN_POINT('',(57.3860839754601,3.00000000004986,64.0110910533819)) ;
#196472=CARTESIAN_POINT('',(57.3860839754601,-2.99999999995014,64.0110910533818)) ;
#196473=CARTESIAN_POINT('Origin',(60.0566078658528,3.00000000004983,66.9917599116864)) ;
#196474=CARTESIAN_POINT('',(-46.0841176604154,3.00000000005113,-60.613533327286)) ;
#196475=CARTESIAN_POINT('',(-5.85091647147829,3.00000000005069,-17.9146369823475)) ;
#196476=CARTESIAN_POINT('',(-46.0841176604154,3.00000000005113,-60.613533327286)) ;
#196477=CARTESIAN_POINT('',(-45.712767762275,3.00000000005117,-64.3658262435518)) ;
#196478=CARTESIAN_POINT('Origin',(-44.2645963709399,3.00000000005114,-62.3279843406267)) ;
#196479=CARTESIAN_POINT('',(35.6411531528819,3.00000000005123,-70.4471903523474)) ;
#196480=CARTESIAN_POINT('Origin',(4.44089209850063E-15,3.00000000005052,
-0.039604774162747)) ;
#196481=CARTESIAN_POINT('',(36.5662411594172,3.00000000005119,-66.7918086956022)) ;
#196482=CARTESIAN_POINT('Origin',(34.512048509326,3.0000000000512,-68.2166920439193)) ;
#196483=CARTESIAN_POINT('',(3.12835464206557,3.0000000000507,-18.5858549944469)) ;
#196484=CARTESIAN_POINT('',(3.12835464206557,3.0000000000507,-18.5858549944469)) ;
#196485=CARTESIAN_POINT('',(0.939891742978034,3.00000000005069,-17.5143466466889)) ;
#196486=CARTESIAN_POINT('Origin',(1.07416199197492,3.00000000005071,-20.0107383427636)) ;
#196487=CARTESIAN_POINT('',(-3.52747078425273,3.00000000005069,-17.1804025929978)) ;
#196488=CARTESIAN_POINT('Origin',(-7.0832228971085E-13,3.00000000005055,
-0.0396047741727124)) ;
#196489=CARTESIAN_POINT('Origin',(-4.03139518200323,3.00000000005071,-19.6290879956887)) ;
#196490=CARTESIAN_POINT('',(-7.97774182302844,3.00000000005051,0.556746971962394)) ;
#196491=CARTESIAN_POINT('Origin',(4.21884749357559E-14,3.00000000005051,
-0.0396047741617706)) ;
#196492=CARTESIAN_POINT('',(-71.8500049958893,3.00000000005026,25.0706222855197)) ;
#196493=CARTESIAN_POINT('',(-18.8081984829363,3.00000000005051,0.00125873500750827)) ;
#196494=CARTESIAN_POINT('',(-71.8500049958893,3.00000000005026,25.0706222855197)) ;
#196495=CARTESIAN_POINT('',(-75.3038941955674,3.00000000005027,23.5579252660689)) ;
#196496=CARTESIAN_POINT('Origin',(-72.9182818039207,3.00000000005028,22.8103602074803)) ;
#196497=CARTESIAN_POINT('',(-55.9478710373819,3.00000000005108,-55.6934962050514)) ;
#196498=CARTESIAN_POINT('Origin',(-1.36779476633819E-12,3.00000000005052,
-0.0396047741619743)) ;
#196499=CARTESIAN_POINT('',(-52.1855285778765,3.00000000005108,-55.4437321289526)) ;
#196500=CARTESIAN_POINT('Origin',(-54.1754536098524,3.00000000005106,-53.9303919929892)) ;
#196501=CARTESIAN_POINT('',(-16.671817376013,3.0000000000506,-8.74595334177845)) ;
#196502=CARTESIAN_POINT('',(-16.671817376013,3.0000000000506,-8.74595334177845)) ;
#196503=CARTESIAN_POINT('',(-16.3290246069902,3.00000000005058,-6.3334871518594)) ;
#196504=CARTESIAN_POINT('Origin',(-18.6617424079881,3.00000000005057,-7.23261320581606)) ;
#196505=CARTESIAN_POINT('',(-17.3919158795974,3.00000000005053,-1.98157852192261)) ;
#196506=CARTESIAN_POINT('Origin',(-1.83275616905121E-11,3.00000000005052,
-0.0396047741661859)) ;
#196507=CARTESIAN_POINT('Origin',(-19.8764752909687,3.00000000005054,-2.25900334303152)) ;
#196508=CARTESIAN_POINT('',(1.67837248110618,3.00000000004974,76.0532975670735)) ;
#196509=CARTESIAN_POINT('',(-5.77318945813033,3.00000000005033,17.8606824715907)) ;
#196510=CARTESIAN_POINT('',(1.67837248110618,3.00000000004974,76.0532975670735)) ;
#196511=CARTESIAN_POINT('',(-0.827598335811217,3.00000000004971,78.8706923106381)) ;
#196512=CARTESIAN_POINT('Origin',(-0.801380185125995,3.00000000004973,76.3708297927037)) ;
#196513=CARTESIAN_POINT('',(-70.2188390521795,3.00000000005014,35.9719842935381)) ;
#196514=CARTESIAN_POINT('Origin',(-6.21724893790088E-13,3.00000000005051,
-0.0396047741604288)) ;
#196515=CARTESIAN_POINT('',(-68.8186715414237,3.00000000005018,32.4709653249907)) ;
#196516=CARTESIAN_POINT('Origin',(-67.9943201961579,3.00000000005016,34.8311443138723)) ;
#196517=CARTESIAN_POINT('',(-13.4321044346723,3.00000000005038,13.1258261134328)) ;
#196518=CARTESIAN_POINT('',(-13.4321044346723,3.00000000005038,13.1258261134328)) ;
#196519=CARTESIAN_POINT('',(-11.0317839532312,3.00000000005037,13.5453038677549)) ;
#196520=CARTESIAN_POINT('Origin',(-12.6077530894068,3.00000000005033,15.4860051023136)) ;
#196521=CARTESIAN_POINT('',(-7.22132435881713,3.00000000005035,15.9009872632986)) ;
#196522=CARTESIAN_POINT('Origin',(-6.28497254240301E-12,3.00000000005062,
-0.0396047741513206)) ;
#196523=CARTESIAN_POINT('Origin',(-8.25294212436289,3.00000000005033,18.1782146972216)) ;
#196524=CARTESIAN_POINT('',(72.8872962349953,3.00000000005029,21.8781681156668)) ;
#196525=CARTESIAN_POINT('',(15.240171174319,3.0000000000504,10.9825176429304)) ;
#196526=CARTESIAN_POINT('',(72.8872962349953,3.00000000005029,21.8781681156668)) ;
#196527=CARTESIAN_POINT('',(74.7924102950029,3.00000000005026,25.1321108463659)) ;
#196528=CARTESIAN_POINT('Origin',(72.423001611602,3.00000000005026,24.3346759016687)) ;
#196529=CARTESIAN_POINT('',(12.5502418525765,3.00000000004972,77.8706726894606)) ;
#196530=CARTESIAN_POINT('Origin',(7.48290318597356E-13,3.00000000005051,
-0.0396047741607486)) ;
#196531=CARTESIAN_POINT('',(9.65325050466174,3.00000000004974,75.4571598955414)) ;
#196532=CARTESIAN_POINT('Origin',(12.1526526866832,3.00000000004974,75.402490594241)) ;
#196533=CARTESIAN_POINT('',(8.37032029494708,3.00000000005034,16.8034275585261)) ;
#196534=CARTESIAN_POINT('',(8.37032029494708,3.00000000005034,16.8034275585261)) ;
#196535=CARTESIAN_POINT('',(9.51100716734754,3.00000000005036,14.6502128783026)) ;
#196536=CARTESIAN_POINT('Origin',(10.869722476968,3.00000000005034,16.7487582572255)) ;
#196537=CARTESIAN_POINT('',(12.9288919820607,3.00000000005039,11.7541966535456)) ;
#196538=CARTESIAN_POINT('Origin',(4.6385117968839E-12,3.00000000005017,
-0.0396047741558747)) ;
#196539=CARTESIAN_POINT('Origin',(14.7758765509265,3.00000000005038,13.4390254289324)) ;
#196540=CARTESIAN_POINT('',(43.3684539402033,3.00000000005115,-62.5865785117813)) ;
#196541=CARTESIAN_POINT('',(15.192133238226,3.00000000005062,-11.1278457379885)) ;
#196542=CARTESIAN_POINT('',(43.3684539402033,3.00000000005115,-62.5865785117813)) ;
#196543=CARTESIAN_POINT('',(47.0518499986506,3.00000000005116,-63.3929260503283)) ;
#196544=CARTESIAN_POINT('Origin',(45.5612567483845,3.00000000005113,-61.3859054320336)) ;
#196545=CARTESIAN_POINT('',(77.9753150841032,3.00000000005039,12.1000057035926)) ;
#196546=CARTESIAN_POINT('Origin',(1.30562227695918E-12,3.00000000005051,
-0.0396047741618544)) ;
#196547=CARTESIAN_POINT('',(74.7847084552218,3.00000000005037,14.109391733215)) ;
#196548=CARTESIAN_POINT('Origin',(75.5050726100008,3.00000000005039,11.7154252579882)) ;
#196549=CARTESIAN_POINT('',(18.6052468736726,3.00000000005054,-2.79546920654119)) ;
#196550=CARTESIAN_POINT('',(18.6052468736726,3.00000000005054,-2.79546920654119)) ;
#196551=CARTESIAN_POINT('',(16.909909649896,3.00000000005056,-4.54570681831662)) ;
#196552=CARTESIAN_POINT('Origin',(19.3256110284515,3.00000000005055,-5.1894356817668)) ;
#196553=CARTESIAN_POINT('',(15.2118190406069,3.0000000000506,-8.69122667273134)) ;
#196554=CARTESIAN_POINT('Origin',(8.04245559038463E-12,3.0000000000501,
-0.0396047741647687)) ;
#196555=CARTESIAN_POINT('Origin',(17.3849360464078,3.00000000005063,-9.92717265824142)) ;
#196556=CARTESIAN_POINT('Origin',(60.0566078658528,-2.99999999995017,66.9917599116863)) ;
#196557=CARTESIAN_POINT('',(-1.38175761627864,-2.99999999994865,-83.3427827144731)) ;
#196558=CARTESIAN_POINT('Origin',(4.413136522885E-14,-2.99999999994949,
-0.0396047741616457)) ;
#196559=CARTESIAN_POINT('Origin',(-7.51482209793153E-13,5.05127219874221E-11,
-0.0396047741696215)) ;
#196560=CARTESIAN_POINT('',(0.939891742978034,-2.99999999994931,-17.5143466466889)) ;
#196561=CARTESIAN_POINT('',(0.939891742978034,3.00000000005069,-17.5143466466889)) ;
#196562=CARTESIAN_POINT('',(-3.52747078425273,-2.99999999994931,-17.1804025929979)) ;
#196563=CARTESIAN_POINT('Origin',(-8.10462807976364E-13,-2.99999999994978,
-0.0396047741726324)) ;
#196564=CARTESIAN_POINT('',(-3.52747078425273,3.00000000005069,-17.1804025929978)) ;
#196565=CARTESIAN_POINT('Origin',(-4.0313951820033,5.07108855651976E-11,
-19.6290879956884)) ;
#196566=CARTESIAN_POINT('',(-5.85091647147829,-2.99999999994931,-17.9146369823476)) ;
#196567=CARTESIAN_POINT('Origin',(-4.03139518200323,-2.99999999994929,-19.6290879956887)) ;
#196568=CARTESIAN_POINT('',(-5.85091647147829,3.00000000005069,-17.9146369823475)) ;
#196569=CARTESIAN_POINT('Origin',(-5.85091647147829,5.06927833043846E-11,
-17.9146369823476)) ;
#196570=CARTESIAN_POINT('',(-46.0841176604154,-2.99999999994887,-60.6135333272861)) ;
#196571=CARTESIAN_POINT('',(-46.0841176604154,3.00000000005113,-60.613533327286)) ;
#196572=CARTESIAN_POINT('',(-46.0841176604154,-2.99999999994887,-60.6135333272861)) ;
#196573=CARTESIAN_POINT('Origin',(-44.2645963709396,5.11477689214468E-11,
-62.3279843406269)) ;
#196574=CARTESIAN_POINT('',(-45.712767762275,-2.99999999994883,-64.3658262435519)) ;
#196575=CARTESIAN_POINT('Origin',(-44.2645963709399,-2.99999999994886,-62.3279843406268)) ;
#196576=CARTESIAN_POINT('',(-45.712767762275,3.00000000005117,-64.3658262435518)) ;
#196577=CARTESIAN_POINT('Origin',(-4.44089209850063E-13,5.05069715077991E-11,
-0.0396047741635108)) ;
#196578=CARTESIAN_POINT('',(35.6411531528819,-2.99999999994877,-70.4471903523475)) ;
#196579=CARTESIAN_POINT('Origin',(4.44089209850063E-15,-2.99999999994949,
-0.0396047741628003)) ;
#196580=CARTESIAN_POINT('',(35.6411531528819,3.00000000005123,-70.4471903523474)) ;
#196581=CARTESIAN_POINT('Origin',(34.5120485093257,5.12090018418964E-11,
-68.2166920439191)) ;
#196582=CARTESIAN_POINT('',(36.5662411594172,-2.99999999994881,-66.7918086956023)) ;
#196583=CARTESIAN_POINT('Origin',(34.512048509326,-2.99999999994881,-68.2166920439194)) ;
#196584=CARTESIAN_POINT('',(36.5662411594172,3.00000000005119,-66.7918086956022)) ;
#196585=CARTESIAN_POINT('Origin',(36.5662411594171,5.11901632194167E-11,
-66.7918086956023)) ;
#196586=CARTESIAN_POINT('',(3.12835464206557,-2.9999999999493,-18.5858549944469)) ;
#196587=CARTESIAN_POINT('',(3.12835464206557,-2.9999999999493,-18.5858549944469)) ;
#196588=CARTESIAN_POINT('',(3.12835464206557,3.0000000000507,-18.5858549944469)) ;
#196589=CARTESIAN_POINT('Origin',(1.07416199197442,5.07138545131367E-11,
-20.0107383427642)) ;
#196590=CARTESIAN_POINT('Origin',(1.07416199197492,-2.99999999994927,-20.0107383427637)) ;
#196591=CARTESIAN_POINT('Origin',(-7.66053886991358E-14,5.05179569195172E-11,
-0.0396047741617249)) ;
#196592=CARTESIAN_POINT('',(-7.97774182302844,-2.99999999994949,0.556746971962333)) ;
#196593=CARTESIAN_POINT('Origin',(3.99680288865056E-14,-2.99999999994949,
-0.0396047741618317)) ;
#196594=CARTESIAN_POINT('',(-7.97774182302844,5.05118844343928E-11,0.556746971962363)) ;
#196595=CARTESIAN_POINT('Origin',(-1.30118138486068E-11,5.0511046670509E-11,
-0.0396047741651795)) ;
#196596=CARTESIAN_POINT('',(-16.3290246069902,-2.99999999994942,-6.33348715185946)) ;
#196597=CARTESIAN_POINT('',(-16.3290246069902,3.00000000005058,-6.3334871518594)) ;
#196598=CARTESIAN_POINT('',(-17.3919158795974,-2.99999999994947,-1.98157852192267)) ;
#196599=CARTESIAN_POINT('Origin',(-1.83542070431031E-11,-2.99999999994958,
-0.0396047741661992)) ;
#196600=CARTESIAN_POINT('',(-17.3919158795974,3.00000000005053,-1.98157852192261)) ;
#196601=CARTESIAN_POINT('Origin',(-19.8764752909685,5.05335163215292E-11,
-2.25900334303148)) ;
#196602=CARTESIAN_POINT('',(-18.8081984829363,-2.99999999994949,0.00125873500744717)) ;
#196603=CARTESIAN_POINT('Origin',(-19.8764752909687,-2.99999999994946,-2.25900334303158)) ;
#196604=CARTESIAN_POINT('',(-18.8081984829363,3.00000000005051,0.00125873500750827)) ;
#196605=CARTESIAN_POINT('Origin',(-18.8081984829363,5.05107067283461E-11,
0.00125873500742087)) ;
#196606=CARTESIAN_POINT('',(-71.8500049958893,-2.99999999994974,25.0706222855196)) ;
#196607=CARTESIAN_POINT('',(-71.8500049958893,3.00000000005026,25.0706222855197)) ;
#196608=CARTESIAN_POINT('',(-71.8500049958893,-2.99999999994974,25.0706222855196)) ;
#196609=CARTESIAN_POINT('Origin',(-72.9182818039209,5.02782135032148E-11,
22.8103602074799)) ;
#196610=CARTESIAN_POINT('',(-75.3038941955674,-2.99999999994973,23.5579252660688)) ;
#196611=CARTESIAN_POINT('Origin',(-72.9182818039207,-2.99999999994972,22.8103602074803)) ;
#196612=CARTESIAN_POINT('',(-75.3038941955674,3.00000000005027,23.5579252660689)) ;
#196613=CARTESIAN_POINT('Origin',(-1.87405646556726E-12,5.05125615832167E-11,
-0.0396047741619432)) ;
#196614=CARTESIAN_POINT('',(-55.9478710373819,-2.99999999994892,-55.6934962050515)) ;
#196615=CARTESIAN_POINT('Origin',(-1.4299672557172E-12,-2.99999999994949,
-0.0396047741618766)) ;
#196616=CARTESIAN_POINT('',(-55.9478710373819,3.00000000005108,-55.6934962050514)) ;
#196617=CARTESIAN_POINT('Origin',(-54.1754536098523,5.10588644666463E-11,
-53.9303919929891)) ;
#196618=CARTESIAN_POINT('',(-52.1855285778765,-2.99999999994892,-55.4437321289526)) ;
#196619=CARTESIAN_POINT('Origin',(-54.1754536098524,-2.99999999994894,-53.9303919929893)) ;
#196620=CARTESIAN_POINT('',(-52.1855285778765,3.00000000005108,-55.4437321289526)) ;
#196621=CARTESIAN_POINT('Origin',(-52.1855285778767,5.1076920470905E-11,
-55.4437321289526)) ;
#196622=CARTESIAN_POINT('',(-16.671817376013,-2.9999999999494,-8.74595334177851)) ;
#196623=CARTESIAN_POINT('',(-16.671817376013,-2.9999999999494,-8.74595334177851)) ;
#196624=CARTESIAN_POINT('',(-16.671817376013,3.0000000000506,-8.74595334177845)) ;
#196625=CARTESIAN_POINT('Origin',(-18.6617424079886,5.05884672997123E-11,
-7.23261320581591)) ;
#196626=CARTESIAN_POINT('Origin',(-18.6617424079882,-2.99999999994939,-7.23261320581612)) ;
#196627=CARTESIAN_POINT('Origin',(-5.98188165668034E-12,5.05112930172867E-11,
-0.0396047741518712)) ;
#196628=CARTESIAN_POINT('',(-11.0317839532312,-2.99999999994963,13.5453038677548)) ;
#196629=CARTESIAN_POINT('',(-11.0317839532312,3.00000000005037,13.5453038677549)) ;
#196630=CARTESIAN_POINT('',(-7.22132435881713,-2.99999999994965,15.9009872632985)) ;
#196631=CARTESIAN_POINT('Origin',(-6.17617068598975E-12,-2.99999999994964,
-0.0396047741515204)) ;
#196632=CARTESIAN_POINT('',(-7.22132435881713,3.00000000005035,15.9009872632986)) ;
#196633=CARTESIAN_POINT('Origin',(-8.25294212436249,5.0325584525273E-11,
18.1782146972211)) ;
#196634=CARTESIAN_POINT('',(-5.77318945813033,-2.99999999994967,17.8606824715907)) ;
#196635=CARTESIAN_POINT('Origin',(-8.25294212436291,-2.99999999994968,18.1782146972216)) ;
#196636=CARTESIAN_POINT('',(-5.77318945813033,3.00000000005033,17.8606824715907)) ;
#196637=CARTESIAN_POINT('Origin',(-5.77318945813045,5.03308505983568E-11,
17.8606824715907)) ;
#196638=CARTESIAN_POINT('',(1.67837248110618,-2.99999999995026,76.0532975670734)) ;
#196639=CARTESIAN_POINT('',(1.67837248110618,3.00000000004974,76.0532975670735)) ;
#196640=CARTESIAN_POINT('',(1.67837248110618,-2.99999999995026,76.0532975670734)) ;
#196641=CARTESIAN_POINT('Origin',(-0.801380185126325,4.97325191999056E-11,
76.3708297927036)) ;
#196642=CARTESIAN_POINT('',(-0.827598335811217,-2.99999999995029,78.870692310638)) ;
#196643=CARTESIAN_POINT('Origin',(-0.801380185126014,-2.99999999995027,
76.3708297927036)) ;
#196644=CARTESIAN_POINT('',(-0.827598335811217,3.00000000004971,78.8706923106381)) ;
#196645=CARTESIAN_POINT('Origin',(-8.15458811587177E-13,5.0476842336372E-11,
-0.0396047741597982)) ;
#196646=CARTESIAN_POINT('',(-70.2188390521795,-2.99999999994985,35.971984293538)) ;
#196647=CARTESIAN_POINT('Origin',(-6.21724893790088E-13,-2.99999999994948,
-0.039604774160491)) ;
#196648=CARTESIAN_POINT('',(-70.2188390521795,3.00000000005014,35.9719842935381)) ;
#196649=CARTESIAN_POINT('Origin',(-67.9943201961576,5.01582369534571E-11,
34.8311443138724)) ;
#196650=CARTESIAN_POINT('',(-68.8186715414237,-2.99999999994982,32.4709653249907)) ;
#196651=CARTESIAN_POINT('Origin',(-67.9943201961579,-2.99999999994984,34.8311443138722)) ;
#196652=CARTESIAN_POINT('',(-68.8186715414237,3.00000000005018,32.4709653249907)) ;
#196653=CARTESIAN_POINT('Origin',(-68.8186715414238,5.01776398209586E-11,
32.4709653249907)) ;
#196654=CARTESIAN_POINT('',(-13.4321044346723,-2.99999999994962,13.1258261134327)) ;
#196655=CARTESIAN_POINT('',(-13.4321044346723,-2.99999999994962,13.1258261134327)) ;
#196656=CARTESIAN_POINT('',(-13.4321044346723,3.00000000005038,13.1258261134328)) ;
#196657=CARTESIAN_POINT('Origin',(-12.6077530894068,5.03536114333649E-11,
15.4860051023138)) ;
#196658=CARTESIAN_POINT('Origin',(-12.6077530894068,-2.99999999994965,15.4860051023136)) ;
#196659=CARTESIAN_POINT('Origin',(4.57522908448027E-12,5.05123757157332E-11,
-0.0396047741559635)) ;
#196660=CARTESIAN_POINT('',(9.51100716734754,-2.99999999994964,14.6502128783025)) ;
#196661=CARTESIAN_POINT('',(9.51100716734754,3.00000000005036,14.6502128783026)) ;
#196662=CARTESIAN_POINT('',(12.9288919820607,-2.99999999994961,11.7541966535455)) ;
#196663=CARTESIAN_POINT('Origin',(4.49862369578113E-12,-2.99999999994982,
-0.0396047741559302)) ;
#196664=CARTESIAN_POINT('',(12.9288919820607,3.00000000005039,11.7541966535456)) ;
#196665=CARTESIAN_POINT('Origin',(14.7758765509261,5.03736560984678E-11,
13.4390254289319)) ;
#196666=CARTESIAN_POINT('',(15.240171174319,-2.9999999999496,10.9825176429303)) ;
#196667=CARTESIAN_POINT('Origin',(14.7758765509265,-2.99999999994962,13.4390254289324)) ;
#196668=CARTESIAN_POINT('',(15.240171174319,3.0000000000504,10.9825176429304)) ;
#196669=CARTESIAN_POINT('Origin',(15.240171174319,5.04019048719329E-11,
10.9825176429304)) ;
#196670=CARTESIAN_POINT('',(72.8872962349953,-2.99999999994971,21.8781681156667)) ;
#196671=CARTESIAN_POINT('',(72.8872962349953,3.00000000005029,21.8781681156668)) ;
#196672=CARTESIAN_POINT('',(72.8872962349953,-2.99999999994971,21.8781681156667)) ;
#196673=CARTESIAN_POINT('Origin',(72.4230016116015,5.02615989705098E-11,
24.3346759016693)) ;
#196674=CARTESIAN_POINT('',(74.7924102950029,-2.99999999994974,25.1321108463658)) ;
#196675=CARTESIAN_POINT('Origin',(72.423001611602,-2.99999999994973,24.3346759016686)) ;
#196676=CARTESIAN_POINT('',(74.7924102950029,3.00000000005026,25.1321108463659)) ;
#196677=CARTESIAN_POINT('Origin',(7.8159700933611E-13,5.0513139743634E-11,
-0.0396047741607131)) ;
#196678=CARTESIAN_POINT('',(12.5502418525765,-2.99999999995028,77.8706726894606)) ;
#196679=CARTESIAN_POINT('Origin',(7.105427357601E-13,-2.99999999994951,
-0.0396047741608285)) ;
#196680=CARTESIAN_POINT('',(12.5502418525765,3.00000000004972,77.8706726894606)) ;
#196681=CARTESIAN_POINT('Origin',(12.1526526866834,4.97404318529672E-11,
75.4024905942403)) ;
#196682=CARTESIAN_POINT('',(9.65325050466174,-2.99999999995026,75.4571598955413)) ;
#196683=CARTESIAN_POINT('Origin',(12.1526526866832,-2.99999999995026,75.402490594241)) ;
#196684=CARTESIAN_POINT('',(9.65325050466174,3.00000000004974,75.4571598955414)) ;
#196685=CARTESIAN_POINT('Origin',(9.65325050466163,4.97402119492563E-11,
75.4571598955414)) ;
#196686=CARTESIAN_POINT('',(8.37032029494708,-2.99999999994966,16.8034275585261)) ;
#196687=CARTESIAN_POINT('',(8.37032029494708,-2.99999999994966,16.8034275585261)) ;
#196688=CARTESIAN_POINT('',(8.37032029494708,3.00000000005034,16.8034275585261)) ;
#196689=CARTESIAN_POINT('Origin',(10.8697224769681,5.03425161977803E-11,
16.7487582572254)) ;
#196690=CARTESIAN_POINT('Origin',(10.869722476968,-2.99999999994966,16.7487582572254)) ;
#196691=CARTESIAN_POINT('Origin',(6.82343070934621E-12,5.05114052809432E-11,
-0.0396047741643929)) ;
#196692=CARTESIAN_POINT('',(16.909909649896,-2.99999999994944,-4.54570681831668)) ;
#196693=CARTESIAN_POINT('',(16.909909649896,3.00000000005056,-4.54570681831662)) ;
#196694=CARTESIAN_POINT('',(15.2118190406069,-2.9999999999494,-8.6912266727314)) ;
#196695=CARTESIAN_POINT('Origin',(8.07576228112339E-12,-2.99999999994975,
-0.0396047741648997)) ;
#196696=CARTESIAN_POINT('',(15.2118190406069,3.0000000000506,-8.69122667273134)) ;
#196697=CARTESIAN_POINT('Origin',(17.3849360464075,5.0614323268569E-11,
-9.92717265824137)) ;
#196698=CARTESIAN_POINT('',(15.192133238226,-2.99999999994937,-11.1278457379886)) ;
#196699=CARTESIAN_POINT('Origin',(17.3849360464078,-2.99999999994938,-9.92717265824148)) ;
#196700=CARTESIAN_POINT('',(15.192133238226,3.00000000005062,-11.1278457379885)) ;
#196701=CARTESIAN_POINT('Origin',(15.1921332382259,5.06217290308086E-11,
-11.1278457379886)) ;
#196702=CARTESIAN_POINT('',(43.3684539402033,-2.99999999994885,-62.5865785117814)) ;
#196703=CARTESIAN_POINT('',(43.3684539402033,3.00000000005115,-62.5865785117813)) ;
#196704=CARTESIAN_POINT('',(43.3684539402033,-2.99999999994885,-62.5865785117814)) ;
#196705=CARTESIAN_POINT('Origin',(45.5612567483847,5.11356786146817E-11,
-61.3859054320333)) ;
#196706=CARTESIAN_POINT('',(47.0518499986506,-2.99999999994884,-63.3929260503284)) ;
#196707=CARTESIAN_POINT('Origin',(45.5612567483845,-2.99999999994886,-61.3859054320336)) ;
#196708=CARTESIAN_POINT('',(47.0518499986506,3.00000000005116,-63.3929260503283)) ;
#196709=CARTESIAN_POINT('Origin',(1.58983937126322E-12,5.05264937529502E-11,
-0.0396047741621075)) ;
#196710=CARTESIAN_POINT('',(77.9753150841032,-2.99999999994961,12.1000057035925)) ;
#196711=CARTESIAN_POINT('Origin',(1.34114941374719E-12,-2.99999999994948,
-0.0396047741619077)) ;
#196712=CARTESIAN_POINT('',(77.9753150841032,3.00000000005039,12.1000057035926)) ;
#196713=CARTESIAN_POINT('Origin',(75.5050726100009,5.03925206957646E-11,
11.7154252579883)) ;
#196714=CARTESIAN_POINT('',(74.7847084552218,-2.99999999994963,14.109391733215)) ;
#196715=CARTESIAN_POINT('Origin',(75.5050726100008,-2.99999999994961,11.7154252579881)) ;
#196716=CARTESIAN_POINT('',(74.7847084552218,3.00000000005037,14.109391733215)) ;
#196717=CARTESIAN_POINT('Origin',(74.7847084552217,5.03663777351449E-11,
14.109391733215)) ;
#196718=CARTESIAN_POINT('',(18.6052468736726,-2.99999999994946,-2.79546920654126)) ;
#196719=CARTESIAN_POINT('',(18.6052468736726,-2.99999999994946,-2.79546920654126)) ;
#196720=CARTESIAN_POINT('',(18.6052468736726,3.00000000005054,-2.79546920654119)) ;
#196721=CARTESIAN_POINT('Origin',(19.3256110284516,5.05639742890559E-11,
-5.18943568176694)) ;
#196722=CARTESIAN_POINT('Origin',(19.3256110284515,-2.99999999994942,-5.18943568176686)) ;
#196723=CARTESIAN_POINT('Origin',(8.99280649946377E-14,-4.74303254878962,
-0.0396047741615924)) ;
#196724=CARTESIAN_POINT('',(-1.38175761627864,-1.60984001328294,-83.3427827144731)) ;
#196725=CARTESIAN_POINT('',(-1.38175761627864,-4.74303254878868,-83.3427827144731)) ;
#196726=CARTESIAN_POINT('Origin',(1.51545442861334E-13,-1.60984001328399,
-0.0396047741615924)) ;
#196727=CARTESIAN_POINT('Origin',(1.96231919602496E-13,-4.74303254878962,
-0.0396047741618233)) ;
#196728=CARTESIAN_POINT('',(-1.34527102914679,-1.60984001328296,-81.1430852968819)) ;
#196729=CARTESIAN_POINT('Origin',(5.63438184997267E-14,-1.60984001328399,
-0.0396047741615391)) ;
#196730=CARTESIAN_POINT('',(-1.34527102914679,-2.99999999994868,-81.1430852968819)) ;
#196731=CARTESIAN_POINT('',(-1.34527102914679,-4.7430325487887,-81.1430852968819)) ;
#196732=CARTESIAN_POINT('Origin',(8.79851747015437E-14,-2.99999999994949,
-0.0396047741615924)) ;
#196733=CARTESIAN_POINT('Origin',(1.34527102914717,-1.60984001328482,81.0638757485583)) ;
#196734=CARTESIAN_POINT('Origin',(60.0566078658528,-2.99999999995017,66.9917599116863)) ;
#196737=UNCERTAINTY_MEASURE_WITH_UNIT(LENGTH_MEASURE(0.01),#196742,
'DISTANCE_ACCURACY_VALUE',
'Maximum model space distance between geometric entities at asserted c
onnectivities') ;
#196738=UNCERTAINTY_MEASURE_WITH_UNIT(LENGTH_MEASURE(0.01),#196742,
'DISTANCE_ACCURACY_VALUE',
'Maximum model space distance between geometric entities at asserted c
onnectivities') ;
#196740=(
GEOMETRIC_REPRESENTATION_CONTEXT(3)
GLOBAL_UNCERTAINTY_ASSIGNED_CONTEXT((#196737))
GLOBAL_UNIT_ASSIGNED_CONTEXT((#196742,#196744,#196745))
REPRESENTATION_CONTEXT('','3D')
) ;
#196741=(
GEOMETRIC_REPRESENTATION_CONTEXT(3)
GLOBAL_UNCERTAINTY_ASSIGNED_CONTEXT((#196738))
GLOBAL_UNIT_ASSIGNED_CONTEXT((#196742,#196744,#196745))
REPRESENTATION_CONTEXT('','3D')
) ;
#196742=(
LENGTH_UNIT()
NAMED_UNIT(*)
SI_UNIT(.MILLI.,.METRE.)
) ;
#196744=(
NAMED_UNIT(*)
PLANE_ANGLE_UNIT()
SI_UNIT($,.RADIAN.)
) ;
#196745=(
NAMED_UNIT(*)
SI_UNIT($,.STERADIAN.)
SOLID_ANGLE_UNIT()
) ;
#196753=PRODUCT_DEFINITION_CONTEXT('part definition',#196761,'design') ;
#196761=APPLICATION_CONTEXT(
'Core Data for Automotive Mechanical Design Process') ;
#196762=PRODUCT_CONTEXT('part definition',#196761,'mechanical') ;
#196765=PRESENTATION_STYLE_ASSIGNMENT((#196767)) ;
#196767=SURFACE_STYLE_USAGE(.BOTH.,#196769) ;
#196769=SURFACE_SIDE_STYLE('',(#196771)) ;
#196771=SURFACE_STYLE_FILL_AREA(#196773) ;
#196773=FILL_AREA_STYLE('Steel - Satin',(#196775)) ;
#196775=FILL_AREA_STYLE_COLOUR('Steel - Satin',#196777) ;
#196777=COLOUR_RGB('Steel - Satin', 0.09019608, 0.27058824, 0.51372549) ;
#197211=CARTESIAN_POINT ( '', ( 0.0, 0.0, 0.0 ) ) ;
#197212=DIRECTION ( '', ( 0.0, 0.0, 1.0 ) ) ;
#197213=DIRECTION ( '', ( 1.0, 0.0, 0.0 ) ) ;
#197214=AXIS2_PLACEMENT_3D ( '', #197211, #197212, #197213 ) ;
#197215=ADVANCED_BREP_SHAPE_REPRESENTATION ( 'Escape Wheel', ( #356, #197214, #197225, #197472 ), #196740 ) ;
#197216=PRODUCT( 'Escape Wheel', 'Escape Wheel', '', ( #196762 ) ) ;
#197217=PRODUCT_DEFINITION_FORMATION ( '', '', #197216 ) ;
#197218=PRODUCT_DEFINITION( 'Escape Wheel', 'Escape Wheel', #197217, #196753 ) ;
#197219=PRODUCT_DEFINITION_SHAPE ( '', '', #197218 ) ;
#197220=SHAPE_DEFINITION_REPRESENTATION ( #197219, #197215 ) ;
#197222=CARTESIAN_POINT ( '', ( 0.0, 0.0, 0.0 ) ) ;
#197223=DIRECTION ( '', ( 0.0, 0.0, 1.0 ) ) ;
#197224=DIRECTION ( '', ( 1.0, 0.0, 0.0 ) ) ;
#197225=AXIS2_PLACEMENT_3D ( '', #197222, #197223, #197224 ) ;
#197469=CARTESIAN_POINT ( '', ( 0.0, 0.0, 0.0 ) ) ;
#197470=DIRECTION ( '', ( 0.0, 0.0, 1.0 ) ) ;
#197471=DIRECTION ( '', ( 1.0, 0.0, 0.0 ) ) ;
#197472=AXIS2_PLACEMENT_3D ( '', #197469, #197470, #197471 ) ;
ENDSEC;
END-ISO-10303-21;
